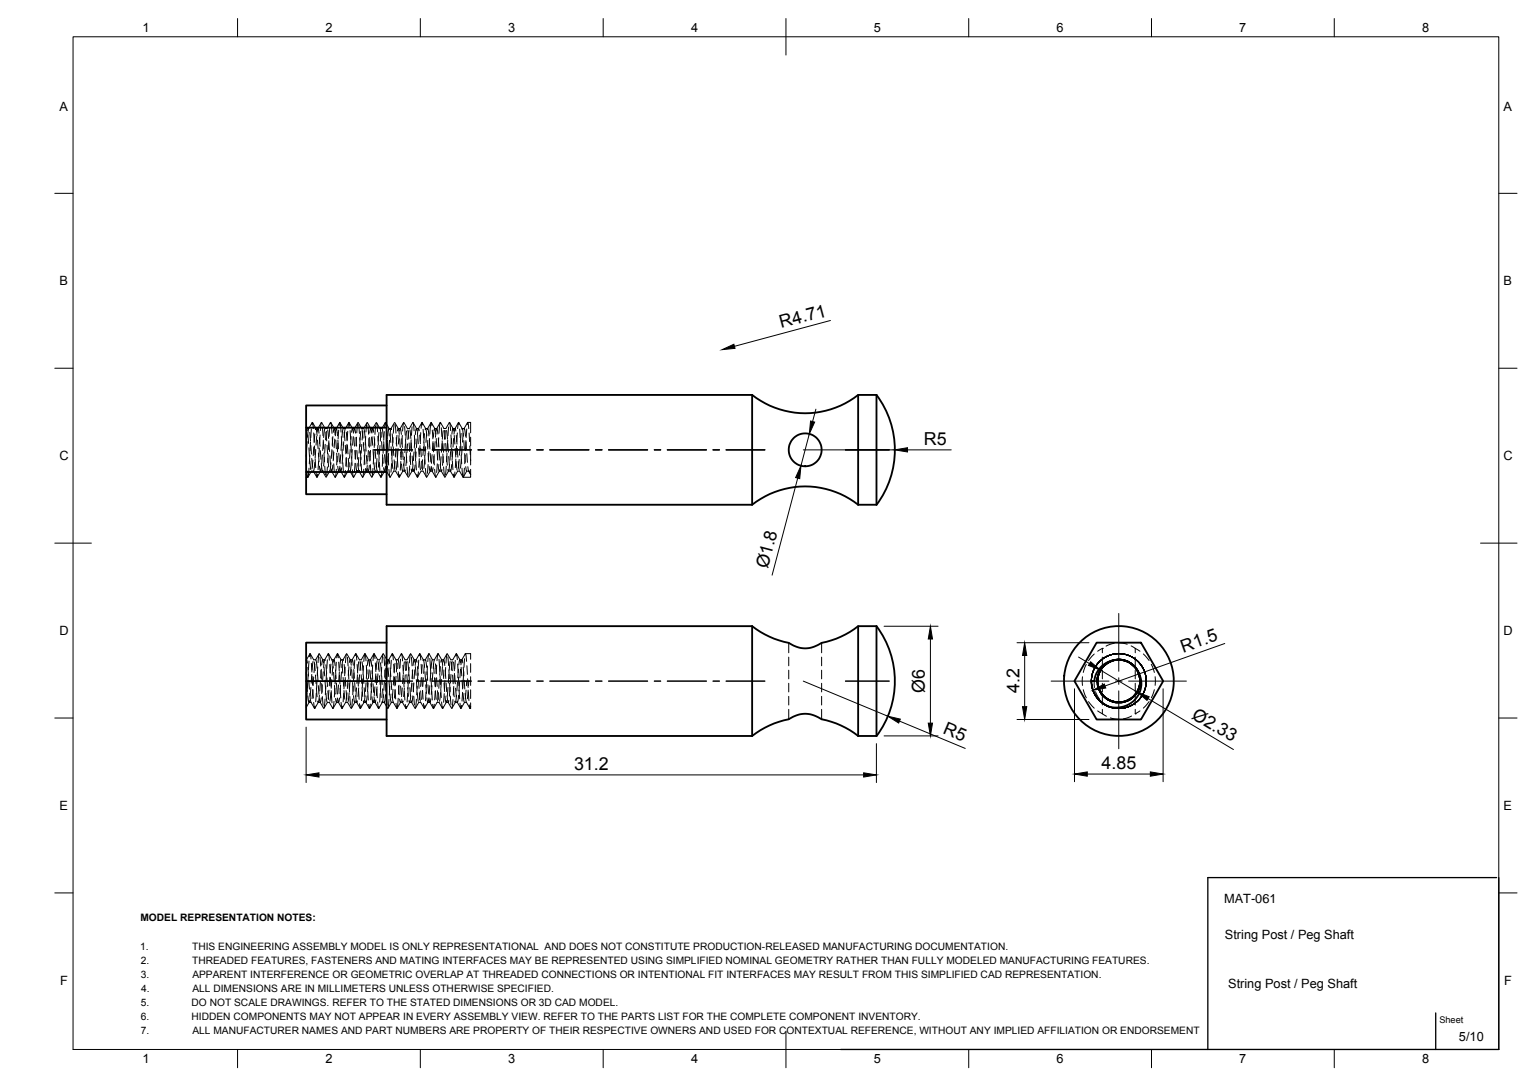
ISO-10303-21;
HEADER;
/* Generated by software containing ST-Developer
 * from STEP Tools, Inc. (www.steptools.com) 
 */

FILE_DESCRIPTION(
/* description */ ('', 'CAx-IF Rec.Pracs.---Representation and Presentation of Product Manufa
cturing Information (PMI)---4.0---2014-10-13'),
/* implementation_level */ '2;1');

FILE_NAME(
/* name */ 'String Post _ Peg Shaft.step',
/* time_stamp */ '2026-10-28T14:45:12+01:00',
/* author */ (''),
/* organization */ (''),
/* preprocessor_version */ 'ST-DEVELOPER v20.2',
/* originating_system */ 'Autodesk Translation Framework v15.17.0.0',
/* authorisation */ '');

FILE_SCHEMA (('AP242_MANAGED_MODEL_BASED_3D_ENGINEERING_MIM_LF { 1 0 10303 442 2 1 4 }'));
ENDSEC;

DATA;
#10=MECHANICAL_DESIGN_GEOMETRIC_PRESENTATION_REPRESENTATION('',(#260),#52164);
#207=TOROIDAL_SURFACE('',#9675,6.705,4.705);
#234=SHAPE_REPRESENTATION_RELATIONSHIP('SRR','None',#52213,#247);
#247=ADVANCED_BREP_SHAPE_REPRESENTATION('',(#273),#52153);
#260=STYLED_ITEM('',(#52318),#273);
#273=MANIFOLD_SOLID_BREP('Body1',#9120);
#285=SPHERICAL_SURFACE('',#9677,5.);
#293=FACE_BOUND('',#1236,.T.);
#294=FACE_BOUND('',#1240,.T.);
#295=FACE_BOUND('',#1241,.T.);
#296=FACE_BOUND('',#1251,.T.);
#343=B_SPLINE_SURFACE_WITH_KNOTS('',3,3,((#20414,#20415,#20416,#20417,#20418,
#20419,#20420,#20421,#20422,#20423,#20424,#20425,#20426,#20427,#20428,#20429,
#20430,#20431,#20432,#20433,#20434,#20435,#20436,#20437,#20438,#20439,#20440,
#20441,#20442,#20443,#20444,#20445,#20446,#20447,#20448),(#20449,#20450,
#20451,#20452,#20453,#20454,#20455,#20456,#20457,#20458,#20459,#20460,#20461,
#20462,#20463,#20464,#20465,#20466,#20467,#20468,#20469,#20470,#20471,#20472,
#20473,#20474,#20475,#20476,#20477,#20478,#20479,#20480,#20481,#20482,#20483),
(#20484,#20485,#20486,#20487,#20488,#20489,#20490,#20491,#20492,#20493,
#20494,#20495,#20496,#20497,#20498,#20499,#20500,#20501,#20502,#20503,#20504,
#20505,#20506,#20507,#20508,#20509,#20510,#20511,#20512,#20513,#20514,#20515,
#20516,#20517,#20518),(#20519,#20520,#20521,#20522,#20523,#20524,#20525,
#20526,#20527,#20528,#20529,#20530,#20531,#20532,#20533,#20534,#20535,#20536,
#20537,#20538,#20539,#20540,#20541,#20542,#20543,#20544,#20545,#20546,#20547,
#20548,#20549,#20550,#20551,#20552,#20553)),.UNSPECIFIED.,.F.,.F.,.F.,(4,
4),(4,1,1,1,1,1,1,1,1,1,1,1,1,1,1,1,1,1,1,1,1,1,1,1,1,1,1,1,1,1,1,1,4),
(-0.1053316651847,1.105331665185),(-0.01760502747868,0.01100314217417,0.03961131182703,
0.06821948147988,0.09682765113273,0.1254358207856,0.1540439904384,0.1826521600913,
0.2112603297441,0.239868499397,0.2684766690498,0.2970848387027,0.3256930083555,
0.3543011780084,0.3829093476613,0.4115175173141,0.440125686967,0.4687338566198,
0.4973420262727,0.5259501959255,0.5545583655784,0.5831665352312,0.6117747048841,
0.6403828745369,0.6689910441898,0.6975992138426,0.7262073834955,0.7548155531483,
0.7834237228012,0.812031892454,0.8406400621069,0.8692482317597,0.8978564014126),
 .UNSPECIFIED.);
#344=B_SPLINE_SURFACE_WITH_KNOTS('',3,3,((#20875,#20876,#20877,#20878,#20879,
#20880,#20881,#20882,#20883,#20884,#20885,#20886,#20887,#20888,#20889,#20890,
#20891,#20892,#20893,#20894,#20895,#20896,#20897,#20898,#20899,#20900,#20901,
#20902,#20903,#20904,#20905,#20906,#20907,#20908,#20909),(#20910,#20911,
#20912,#20913,#20914,#20915,#20916,#20917,#20918,#20919,#20920,#20921,#20922,
#20923,#20924,#20925,#20926,#20927,#20928,#20929,#20930,#20931,#20932,#20933,
#20934,#20935,#20936,#20937,#20938,#20939,#20940,#20941,#20942,#20943,#20944),
(#20945,#20946,#20947,#20948,#20949,#20950,#20951,#20952,#20953,#20954,
#20955,#20956,#20957,#20958,#20959,#20960,#20961,#20962,#20963,#20964,#20965,
#20966,#20967,#20968,#20969,#20970,#20971,#20972,#20973,#20974,#20975,#20976,
#20977,#20978,#20979),(#20980,#20981,#20982,#20983,#20984,#20985,#20986,
#20987,#20988,#20989,#20990,#20991,#20992,#20993,#20994,#20995,#20996,#20997,
#20998,#20999,#21000,#21001,#21002,#21003,#21004,#21005,#21006,#21007,#21008,
#21009,#21010,#21011,#21012,#21013,#21014)),.UNSPECIFIED.,.F.,.F.,.F.,(4,
4),(4,1,1,1,1,1,1,1,1,1,1,1,1,1,1,1,1,1,1,1,1,1,1,1,1,1,1,1,1,1,1,1,4),
(-0.1053316651848,1.105331665185),(-0.02,0.0125,0.045,0.0775,0.11,0.1425,
0.175,0.2075,0.24,0.2725,0.305,0.3375,0.37,0.4025,0.435,0.4675,0.5,0.5325,
0.565,0.5975,0.63,0.6625,0.695,0.7275,0.76,0.7925,0.825,0.8575,0.89,0.9225,
0.955,0.9875,1.02),.UNSPECIFIED.);
#345=B_SPLINE_SURFACE_WITH_KNOTS('',3,3,((#21330,#21331,#21332,#21333,#21334,
#21335,#21336,#21337,#21338,#21339,#21340,#21341,#21342,#21343,#21344,#21345,
#21346,#21347,#21348,#21349,#21350,#21351,#21352,#21353,#21354,#21355,#21356,
#21357,#21358,#21359,#21360,#21361,#21362,#21363,#21364),(#21365,#21366,
#21367,#21368,#21369,#21370,#21371,#21372,#21373,#21374,#21375,#21376,#21377,
#21378,#21379,#21380,#21381,#21382,#21383,#21384,#21385,#21386,#21387,#21388,
#21389,#21390,#21391,#21392,#21393,#21394,#21395,#21396,#21397,#21398,#21399),
(#21400,#21401,#21402,#21403,#21404,#21405,#21406,#21407,#21408,#21409,
#21410,#21411,#21412,#21413,#21414,#21415,#21416,#21417,#21418,#21419,#21420,
#21421,#21422,#21423,#21424,#21425,#21426,#21427,#21428,#21429,#21430,#21431,
#21432,#21433,#21434),(#21435,#21436,#21437,#21438,#21439,#21440,#21441,
#21442,#21443,#21444,#21445,#21446,#21447,#21448,#21449,#21450,#21451,#21452,
#21453,#21454,#21455,#21456,#21457,#21458,#21459,#21460,#21461,#21462,#21463,
#21464,#21465,#21466,#21467,#21468,#21469)),.UNSPECIFIED.,.F.,.F.,.F.,(4,
4),(4,1,1,1,1,1,1,1,1,1,1,1,1,1,1,1,1,1,1,1,1,1,1,1,1,1,1,1,1,1,1,1,4),
(-0.3507678241798,1.35076782418),(-0.01888802807688,0.01180501754805,0.04249806317297,
0.0731911087979,0.1038841544228,0.1345772000478,0.1652702456727,0.1959632912976,
0.2266563369225,0.2573493825475,0.2880424281724,0.3187354737973,0.3494285194222,
0.3801215650472,0.4108146106721,0.441507656297,0.4722007019219,0.5028937475469,
0.5335867931718,0.5642798387967,0.5949728844216,0.6256659300466,0.6563589756715,
0.6870520212964,0.7177450669213,0.7484381125463,0.7791311581712,0.8098242037961,
0.840517249421,0.871210295046,0.9019033406709,0.9325963862958,0.9632894319207),
 .UNSPECIFIED.);
#346=B_SPLINE_SURFACE_WITH_KNOTS('',3,3,((#21471,#21472,#21473,#21474,#21475,
#21476,#21477,#21478,#21479,#21480,#21481,#21482,#21483,#21484,#21485,#21486,
#21487,#21488,#21489,#21490,#21491,#21492,#21493,#21494,#21495,#21496,#21497,
#21498,#21499,#21500,#21501,#21502,#21503,#21504,#21505),(#21506,#21507,
#21508,#21509,#21510,#21511,#21512,#21513,#21514,#21515,#21516,#21517,#21518,
#21519,#21520,#21521,#21522,#21523,#21524,#21525,#21526,#21527,#21528,#21529,
#21530,#21531,#21532,#21533,#21534,#21535,#21536,#21537,#21538,#21539,#21540),
(#21541,#21542,#21543,#21544,#21545,#21546,#21547,#21548,#21549,#21550,
#21551,#21552,#21553,#21554,#21555,#21556,#21557,#21558,#21559,#21560,#21561,
#21562,#21563,#21564,#21565,#21566,#21567,#21568,#21569,#21570,#21571,#21572,
#21573,#21574,#21575),(#21576,#21577,#21578,#21579,#21580,#21581,#21582,
#21583,#21584,#21585,#21586,#21587,#21588,#21589,#21590,#21591,#21592,#21593,
#21594,#21595,#21596,#21597,#21598,#21599,#21600,#21601,#21602,#21603,#21604,
#21605,#21606,#21607,#21608,#21609,#21610)),.UNSPECIFIED.,.F.,.F.,.F.,(4,
4),(4,1,1,1,1,1,1,1,1,1,1,1,1,1,1,1,1,1,1,1,1,1,1,1,1,1,1,1,1,1,1,1,4),
(-0.3507678241798,1.35076782418),(-0.02,0.0125,0.045,0.0775,0.11,0.1425,
0.175,0.2075,0.24,0.2725,0.305,0.3375,0.37,0.4025,0.435,0.4675,0.5,0.5325,
0.565,0.5975,0.63,0.6625,0.695,0.7275,0.76,0.7925,0.825,0.8575,0.89,0.9225,
0.955,0.9875,1.02),.UNSPECIFIED.);
#347=B_SPLINE_SURFACE_WITH_KNOTS('',3,3,((#21858,#21859,#21860,#21861,#21862,
#21863,#21864,#21865,#21866,#21867,#21868,#21869,#21870,#21871,#21872,#21873,
#21874,#21875,#21876,#21877,#21878,#21879,#21880,#21881,#21882,#21883,#21884,
#21885,#21886,#21887,#21888,#21889,#21890,#21891,#21892),(#21893,#21894,
#21895,#21896,#21897,#21898,#21899,#21900,#21901,#21902,#21903,#21904,#21905,
#21906,#21907,#21908,#21909,#21910,#21911,#21912,#21913,#21914,#21915,#21916,
#21917,#21918,#21919,#21920,#21921,#21922,#21923,#21924,#21925,#21926,#21927),
(#21928,#21929,#21930,#21931,#21932,#21933,#21934,#21935,#21936,#21937,
#21938,#21939,#21940,#21941,#21942,#21943,#21944,#21945,#21946,#21947,#21948,
#21949,#21950,#21951,#21952,#21953,#21954,#21955,#21956,#21957,#21958,#21959,
#21960,#21961,#21962),(#21963,#21964,#21965,#21966,#21967,#21968,#21969,
#21970,#21971,#21972,#21973,#21974,#21975,#21976,#21977,#21978,#21979,#21980,
#21981,#21982,#21983,#21984,#21985,#21986,#21987,#21988,#21989,#21990,#21991,
#21992,#21993,#21994,#21995,#21996,#21997)),.UNSPECIFIED.,.F.,.F.,.F.,(4,
4),(4,1,1,1,1,1,1,1,1,1,1,1,1,1,1,1,1,1,1,1,1,1,1,1,1,1,1,1,1,1,1,1,4),
(-0.3507678241798,1.35076782418),(-0.02,0.0125,0.045,0.0775,0.11,0.1425,
0.175,0.2075,0.24,0.2725,0.305,0.3375,0.37,0.4025,0.435,0.4675,0.5,0.5325,
0.565,0.5975,0.63,0.6625,0.695,0.7275,0.76,0.7925,0.825,0.8575,0.89,0.9225,
0.955,0.9875,1.02),.UNSPECIFIED.);
#348=B_SPLINE_SURFACE_WITH_KNOTS('',3,3,((#22245,#22246,#22247,#22248,#22249,
#22250,#22251,#22252,#22253,#22254,#22255,#22256,#22257,#22258,#22259,#22260,
#22261,#22262,#22263,#22264,#22265,#22266,#22267,#22268,#22269,#22270,#22271,
#22272,#22273,#22274,#22275,#22276,#22277,#22278,#22279),(#22280,#22281,
#22282,#22283,#22284,#22285,#22286,#22287,#22288,#22289,#22290,#22291,#22292,
#22293,#22294,#22295,#22296,#22297,#22298,#22299,#22300,#22301,#22302,#22303,
#22304,#22305,#22306,#22307,#22308,#22309,#22310,#22311,#22312,#22313,#22314),
(#22315,#22316,#22317,#22318,#22319,#22320,#22321,#22322,#22323,#22324,
#22325,#22326,#22327,#22328,#22329,#22330,#22331,#22332,#22333,#22334,#22335,
#22336,#22337,#22338,#22339,#22340,#22341,#22342,#22343,#22344,#22345,#22346,
#22347,#22348,#22349),(#22350,#22351,#22352,#22353,#22354,#22355,#22356,
#22357,#22358,#22359,#22360,#22361,#22362,#22363,#22364,#22365,#22366,#22367,
#22368,#22369,#22370,#22371,#22372,#22373,#22374,#22375,#22376,#22377,#22378,
#22379,#22380,#22381,#22382,#22383,#22384)),.UNSPECIFIED.,.F.,.F.,.F.,(4,
4),(4,1,1,1,1,1,1,1,1,1,1,1,1,1,1,1,1,1,1,1,1,1,1,1,1,1,1,1,1,1,1,1,4),
(-0.3507678241798,1.35076782418),(-0.02,0.0125,0.045,0.0775,0.11,0.1425,
0.175,0.2075,0.24,0.2725,0.305,0.3375,0.37,0.4025,0.435,0.4675,0.5,0.5325,
0.565,0.5975,0.63,0.6625,0.695,0.7275,0.76,0.7925,0.825,0.8575,0.89,0.9225,
0.955,0.9875,1.02),.UNSPECIFIED.);
#349=B_SPLINE_SURFACE_WITH_KNOTS('',3,3,((#22632,#22633,#22634,#22635,#22636,
#22637,#22638,#22639,#22640,#22641,#22642,#22643,#22644,#22645,#22646,#22647,
#22648,#22649,#22650,#22651,#22652,#22653,#22654,#22655,#22656,#22657,#22658,
#22659,#22660,#22661,#22662,#22663,#22664,#22665,#22666),(#22667,#22668,
#22669,#22670,#22671,#22672,#22673,#22674,#22675,#22676,#22677,#22678,#22679,
#22680,#22681,#22682,#22683,#22684,#22685,#22686,#22687,#22688,#22689,#22690,
#22691,#22692,#22693,#22694,#22695,#22696,#22697,#22698,#22699,#22700,#22701),
(#22702,#22703,#22704,#22705,#22706,#22707,#22708,#22709,#22710,#22711,
#22712,#22713,#22714,#22715,#22716,#22717,#22718,#22719,#22720,#22721,#22722,
#22723,#22724,#22725,#22726,#22727,#22728,#22729,#22730,#22731,#22732,#22733,
#22734,#22735,#22736),(#22737,#22738,#22739,#22740,#22741,#22742,#22743,
#22744,#22745,#22746,#22747,#22748,#22749,#22750,#22751,#22752,#22753,#22754,
#22755,#22756,#22757,#22758,#22759,#22760,#22761,#22762,#22763,#22764,#22765,
#22766,#22767,#22768,#22769,#22770,#22771)),.UNSPECIFIED.,.F.,.F.,.F.,(4,
4),(4,1,1,1,1,1,1,1,1,1,1,1,1,1,1,1,1,1,1,1,1,1,1,1,1,1,1,1,1,1,1,1,4),
(-0.3507678241798,1.35076782418),(-0.02,0.0125,0.045,0.0775,0.11,0.1425,
0.175,0.2075,0.24,0.2725,0.305,0.3375,0.37,0.4025,0.435,0.4675,0.5,0.5325,
0.565,0.5975,0.63,0.6625,0.695,0.7275,0.76,0.7925,0.825,0.8575,0.89,0.9225,
0.955,0.9875,1.02),.UNSPECIFIED.);
#350=B_SPLINE_SURFACE_WITH_KNOTS('',3,3,((#23060,#23061,#23062,#23063,#23064,
#23065,#23066,#23067,#23068,#23069,#23070,#23071,#23072,#23073,#23074,#23075,
#23076,#23077,#23078,#23079,#23080,#23081,#23082,#23083,#23084,#23085,#23086,
#23087,#23088,#23089,#23090,#23091,#23092,#23093,#23094),(#23095,#23096,
#23097,#23098,#23099,#23100,#23101,#23102,#23103,#23104,#23105,#23106,#23107,
#23108,#23109,#23110,#23111,#23112,#23113,#23114,#23115,#23116,#23117,#23118,
#23119,#23120,#23121,#23122,#23123,#23124,#23125,#23126,#23127,#23128,#23129),
(#23130,#23131,#23132,#23133,#23134,#23135,#23136,#23137,#23138,#23139,
#23140,#23141,#23142,#23143,#23144,#23145,#23146,#23147,#23148,#23149,#23150,
#23151,#23152,#23153,#23154,#23155,#23156,#23157,#23158,#23159,#23160,#23161,
#23162,#23163,#23164),(#23165,#23166,#23167,#23168,#23169,#23170,#23171,
#23172,#23173,#23174,#23175,#23176,#23177,#23178,#23179,#23180,#23181,#23182,
#23183,#23184,#23185,#23186,#23187,#23188,#23189,#23190,#23191,#23192,#23193,
#23194,#23195,#23196,#23197,#23198,#23199)),.UNSPECIFIED.,.F.,.F.,.F.,(4,
4),(4,1,1,1,1,1,1,1,1,1,1,1,1,1,1,1,1,1,1,1,1,1,1,1,1,1,1,1,1,1,1,1,4),
(-0.1053316651848,1.105331665185),(-0.02,0.0125,0.045,0.0775,0.11,0.1425,
0.175,0.2075,0.24,0.2725,0.305,0.3375,0.37,0.4025,0.435,0.4675,0.5,0.5325,
0.565,0.5975,0.63,0.6625,0.695,0.7275,0.76,0.7925,0.825,0.8575,0.89,0.9225,
0.955,0.9875,1.02),.UNSPECIFIED.);
#351=B_SPLINE_SURFACE_WITH_KNOTS('',3,3,((#23447,#23448,#23449,#23450,#23451,
#23452,#23453,#23454,#23455,#23456,#23457,#23458,#23459,#23460,#23461,#23462,
#23463,#23464,#23465,#23466,#23467,#23468,#23469,#23470,#23471,#23472,#23473,
#23474,#23475,#23476,#23477,#23478,#23479,#23480,#23481),(#23482,#23483,
#23484,#23485,#23486,#23487,#23488,#23489,#23490,#23491,#23492,#23493,#23494,
#23495,#23496,#23497,#23498,#23499,#23500,#23501,#23502,#23503,#23504,#23505,
#23506,#23507,#23508,#23509,#23510,#23511,#23512,#23513,#23514,#23515,#23516),
(#23517,#23518,#23519,#23520,#23521,#23522,#23523,#23524,#23525,#23526,
#23527,#23528,#23529,#23530,#23531,#23532,#23533,#23534,#23535,#23536,#23537,
#23538,#23539,#23540,#23541,#23542,#23543,#23544,#23545,#23546,#23547,#23548,
#23549,#23550,#23551),(#23552,#23553,#23554,#23555,#23556,#23557,#23558,
#23559,#23560,#23561,#23562,#23563,#23564,#23565,#23566,#23567,#23568,#23569,
#23570,#23571,#23572,#23573,#23574,#23575,#23576,#23577,#23578,#23579,#23580,
#23581,#23582,#23583,#23584,#23585,#23586)),.UNSPECIFIED.,.F.,.F.,.F.,(4,
4),(4,1,1,1,1,1,1,1,1,1,1,1,1,1,1,1,1,1,1,1,1,1,1,1,1,1,1,1,1,1,1,1,4),
(-0.1053316651847,1.105331665185),(-0.02,0.0125,0.045,0.0775,0.11,0.1425,
0.175,0.2075,0.24,0.2725,0.305,0.3375,0.37,0.4025,0.435,0.4675,0.5,0.5325,
0.565,0.5975,0.63,0.6625,0.695,0.7275,0.76,0.7925,0.825,0.8575,0.89,0.9225,
0.955,0.9875,1.02),.UNSPECIFIED.);
#352=B_SPLINE_SURFACE_WITH_KNOTS('',3,3,((#23641,#23642,#23643,#23644,#23645,
#23646,#23647,#23648,#23649,#23650,#23651,#23652,#23653,#23654,#23655,#23656,
#23657,#23658,#23659,#23660,#23661,#23662,#23663,#23664,#23665,#23666,#23667,
#23668,#23669,#23670,#23671,#23672,#23673,#23674,#23675),(#23676,#23677,
#23678,#23679,#23680,#23681,#23682,#23683,#23684,#23685,#23686,#23687,#23688,
#23689,#23690,#23691,#23692,#23693,#23694,#23695,#23696,#23697,#23698,#23699,
#23700,#23701,#23702,#23703,#23704,#23705,#23706,#23707,#23708,#23709,#23710),
(#23711,#23712,#23713,#23714,#23715,#23716,#23717,#23718,#23719,#23720,
#23721,#23722,#23723,#23724,#23725,#23726,#23727,#23728,#23729,#23730,#23731,
#23732,#23733,#23734,#23735,#23736,#23737,#23738,#23739,#23740,#23741,#23742,
#23743,#23744,#23745),(#23746,#23747,#23748,#23749,#23750,#23751,#23752,
#23753,#23754,#23755,#23756,#23757,#23758,#23759,#23760,#23761,#23762,#23763,
#23764,#23765,#23766,#23767,#23768,#23769,#23770,#23771,#23772,#23773,#23774,
#23775,#23776,#23777,#23778,#23779,#23780)),.UNSPECIFIED.,.F.,.F.,.F.,(4,
4),(4,1,1,1,1,1,1,1,1,1,1,1,1,1,1,1,1,1,1,1,1,1,1,1,1,1,1,1,1,1,1,1,4),
(-0.1053316651847,1.105331665185),(-0.02,0.0125,0.045,0.0775,0.11,0.1425,
0.175,0.2075,0.24,0.2725,0.305,0.3375,0.37,0.4025,0.435,0.4675,0.5,0.5325,
0.565,0.5975,0.63,0.6625,0.695,0.7275,0.76,0.7925,0.825,0.8575,0.89,0.9225,
0.955,0.9875,1.02),.UNSPECIFIED.);
#353=B_SPLINE_SURFACE_WITH_KNOTS('',3,3,((#24018,#24019,#24020,#24021,#24022,
#24023,#24024,#24025,#24026,#24027,#24028,#24029,#24030,#24031,#24032,#24033,
#24034,#24035,#24036,#24037,#24038,#24039,#24040,#24041,#24042,#24043,#24044,
#24045,#24046,#24047,#24048,#24049,#24050,#24051,#24052),(#24053,#24054,
#24055,#24056,#24057,#24058,#24059,#24060,#24061,#24062,#24063,#24064,#24065,
#24066,#24067,#24068,#24069,#24070,#24071,#24072,#24073,#24074,#24075,#24076,
#24077,#24078,#24079,#24080,#24081,#24082,#24083,#24084,#24085,#24086,#24087),
(#24088,#24089,#24090,#24091,#24092,#24093,#24094,#24095,#24096,#24097,
#24098,#24099,#24100,#24101,#24102,#24103,#24104,#24105,#24106,#24107,#24108,
#24109,#24110,#24111,#24112,#24113,#24114,#24115,#24116,#24117,#24118,#24119,
#24120,#24121,#24122),(#24123,#24124,#24125,#24126,#24127,#24128,#24129,
#24130,#24131,#24132,#24133,#24134,#24135,#24136,#24137,#24138,#24139,#24140,
#24141,#24142,#24143,#24144,#24145,#24146,#24147,#24148,#24149,#24150,#24151,
#24152,#24153,#24154,#24155,#24156,#24157)),.UNSPECIFIED.,.F.,.F.,.F.,(4,
4),(4,1,1,1,1,1,1,1,1,1,1,1,1,1,1,1,1,1,1,1,1,1,1,1,1,1,1,1,1,1,1,1,4),
(-0.1053316651848,1.105331665185),(-0.02,0.0125,0.045,0.0775,0.11,0.1425,
0.175,0.2075,0.24,0.2725,0.305,0.3375,0.37,0.4025,0.435,0.4675,0.5,0.5325,
0.565,0.5975,0.63,0.6625,0.695,0.7275,0.76,0.7925,0.825,0.8575,0.89,0.9225,
0.955,0.9875,1.02),.UNSPECIFIED.);
#354=B_SPLINE_SURFACE_WITH_KNOTS('',3,3,((#24159,#24160,#24161,#24162,#24163,
#24164,#24165,#24166,#24167,#24168,#24169,#24170,#24171,#24172,#24173,#24174,
#24175,#24176,#24177,#24178,#24179,#24180,#24181,#24182,#24183,#24184,#24185,
#24186,#24187,#24188,#24189,#24190,#24191,#24192,#24193),(#24194,#24195,
#24196,#24197,#24198,#24199,#24200,#24201,#24202,#24203,#24204,#24205,#24206,
#24207,#24208,#24209,#24210,#24211,#24212,#24213,#24214,#24215,#24216,#24217,
#24218,#24219,#24220,#24221,#24222,#24223,#24224,#24225,#24226,#24227,#24228),
(#24229,#24230,#24231,#24232,#24233,#24234,#24235,#24236,#24237,#24238,
#24239,#24240,#24241,#24242,#24243,#24244,#24245,#24246,#24247,#24248,#24249,
#24250,#24251,#24252,#24253,#24254,#24255,#24256,#24257,#24258,#24259,#24260,
#24261,#24262,#24263),(#24264,#24265,#24266,#24267,#24268,#24269,#24270,
#24271,#24272,#24273,#24274,#24275,#24276,#24277,#24278,#24279,#24280,#24281,
#24282,#24283,#24284,#24285,#24286,#24287,#24288,#24289,#24290,#24291,#24292,
#24293,#24294,#24295,#24296,#24297,#24298)),.UNSPECIFIED.,.F.,.F.,.F.,(4,
4),(4,1,1,1,1,1,1,1,1,1,1,1,1,1,1,1,1,1,1,1,1,1,1,1,1,1,1,1,1,1,1,1,4),
(-0.1053316651848,1.105331665185),(-0.02,0.0125,0.045,0.0775,0.11,0.1425,
0.175,0.2075,0.24,0.2725,0.305,0.3375,0.37,0.4025,0.435,0.4675,0.5,0.5325,
0.565,0.5975,0.63,0.6625,0.695,0.7275,0.76,0.7925,0.825,0.8575,0.89,0.9225,
0.955,0.9875,1.02),.UNSPECIFIED.);
#355=B_SPLINE_SURFACE_WITH_KNOTS('',3,3,((#24485,#24486,#24487,#24488,#24489,
#24490,#24491,#24492,#24493,#24494,#24495,#24496,#24497,#24498,#24499,#24500,
#24501,#24502,#24503,#24504,#24505,#24506,#24507,#24508,#24509,#24510,#24511,
#24512,#24513,#24514,#24515,#24516,#24517,#24518,#24519),(#24520,#24521,
#24522,#24523,#24524,#24525,#24526,#24527,#24528,#24529,#24530,#24531,#24532,
#24533,#24534,#24535,#24536,#24537,#24538,#24539,#24540,#24541,#24542,#24543,
#24544,#24545,#24546,#24547,#24548,#24549,#24550,#24551,#24552,#24553,#24554),
(#24555,#24556,#24557,#24558,#24559,#24560,#24561,#24562,#24563,#24564,
#24565,#24566,#24567,#24568,#24569,#24570,#24571,#24572,#24573,#24574,#24575,
#24576,#24577,#24578,#24579,#24580,#24581,#24582,#24583,#24584,#24585,#24586,
#24587,#24588,#24589),(#24590,#24591,#24592,#24593,#24594,#24595,#24596,
#24597,#24598,#24599,#24600,#24601,#24602,#24603,#24604,#24605,#24606,#24607,
#24608,#24609,#24610,#24611,#24612,#24613,#24614,#24615,#24616,#24617,#24618,
#24619,#24620,#24621,#24622,#24623,#24624)),.UNSPECIFIED.,.F.,.F.,.F.,(4,
4),(4,1,1,1,1,1,1,1,1,1,1,1,1,1,1,1,1,1,1,1,1,1,1,1,1,1,1,1,1,1,1,1,4),
(-0.1053316651847,1.105331665185),(-0.02,0.0125,0.045,0.0775,0.11,0.1425,
0.175,0.2075,0.24,0.2725,0.305,0.3375,0.37,0.4025,0.435,0.4675,0.5,0.5325,
0.565,0.5975,0.63,0.6625,0.695,0.7275,0.76,0.7925,0.825,0.8575,0.89,0.9225,
0.955,0.9875,1.02),.UNSPECIFIED.);
#356=B_SPLINE_SURFACE_WITH_KNOTS('',3,3,((#24675,#24676,#24677,#24678,#24679,
#24680,#24681,#24682,#24683,#24684,#24685,#24686,#24687,#24688,#24689,#24690,
#24691,#24692,#24693,#24694,#24695,#24696,#24697,#24698,#24699,#24700,#24701,
#24702,#24703,#24704,#24705,#24706,#24707,#24708,#24709),(#24710,#24711,
#24712,#24713,#24714,#24715,#24716,#24717,#24718,#24719,#24720,#24721,#24722,
#24723,#24724,#24725,#24726,#24727,#24728,#24729,#24730,#24731,#24732,#24733,
#24734,#24735,#24736,#24737,#24738,#24739,#24740,#24741,#24742,#24743,#24744),
(#24745,#24746,#24747,#24748,#24749,#24750,#24751,#24752,#24753,#24754,
#24755,#24756,#24757,#24758,#24759,#24760,#24761,#24762,#24763,#24764,#24765,
#24766,#24767,#24768,#24769,#24770,#24771,#24772,#24773,#24774,#24775,#24776,
#24777,#24778,#24779),(#24780,#24781,#24782,#24783,#24784,#24785,#24786,
#24787,#24788,#24789,#24790,#24791,#24792,#24793,#24794,#24795,#24796,#24797,
#24798,#24799,#24800,#24801,#24802,#24803,#24804,#24805,#24806,#24807,#24808,
#24809,#24810,#24811,#24812,#24813,#24814)),.UNSPECIFIED.,.F.,.F.,.F.,(4,
4),(4,1,1,1,1,1,1,1,1,1,1,1,1,1,1,1,1,1,1,1,1,1,1,1,1,1,1,1,1,1,1,1,4),
(-0.1053316651847,1.105331665185),(-0.02,0.0125,0.045,0.0775,0.11,0.1425,
0.175,0.2075,0.24,0.2725,0.305,0.3375,0.37,0.4025,0.435,0.4675,0.5,0.5325,
0.565,0.5975,0.63,0.6625,0.695,0.7275,0.76,0.7925,0.825,0.8575,0.89,0.9225,
0.955,0.9875,1.02),.UNSPECIFIED.);
#357=B_SPLINE_SURFACE_WITH_KNOTS('',3,3,((#24997,#24998,#24999,#25000,#25001,
#25002,#25003,#25004,#25005,#25006,#25007,#25008,#25009,#25010,#25011,#25012,
#25013,#25014,#25015,#25016,#25017,#25018,#25019,#25020,#25021,#25022,#25023,
#25024,#25025,#25026,#25027,#25028,#25029,#25030,#25031),(#25032,#25033,
#25034,#25035,#25036,#25037,#25038,#25039,#25040,#25041,#25042,#25043,#25044,
#25045,#25046,#25047,#25048,#25049,#25050,#25051,#25052,#25053,#25054,#25055,
#25056,#25057,#25058,#25059,#25060,#25061,#25062,#25063,#25064,#25065,#25066),
(#25067,#25068,#25069,#25070,#25071,#25072,#25073,#25074,#25075,#25076,
#25077,#25078,#25079,#25080,#25081,#25082,#25083,#25084,#25085,#25086,#25087,
#25088,#25089,#25090,#25091,#25092,#25093,#25094,#25095,#25096,#25097,#25098,
#25099,#25100,#25101),(#25102,#25103,#25104,#25105,#25106,#25107,#25108,
#25109,#25110,#25111,#25112,#25113,#25114,#25115,#25116,#25117,#25118,#25119,
#25120,#25121,#25122,#25123,#25124,#25125,#25126,#25127,#25128,#25129,#25130,
#25131,#25132,#25133,#25134,#25135,#25136)),.UNSPECIFIED.,.F.,.F.,.F.,(4,
4),(4,1,1,1,1,1,1,1,1,1,1,1,1,1,1,1,1,1,1,1,1,1,1,1,1,1,1,1,1,1,1,1,4),
(-0.1053316651848,1.105331665185),(-0.02,0.0125,0.045,0.0775,0.11,0.1425,
0.175,0.2075,0.24,0.2725,0.305,0.3375,0.37,0.4025,0.435,0.4675,0.5,0.5325,
0.565,0.5975,0.63,0.6625,0.695,0.7275,0.76,0.7925,0.825,0.8575,0.89,0.9225,
0.955,0.9875,1.02),.UNSPECIFIED.);
#425=PLANE('',#9668);
#426=PLANE('',#9680);
#427=PLANE('',#9681);
#428=PLANE('',#9682);
#429=PLANE('',#9683);
#430=PLANE('',#9684);
#431=PLANE('',#9685);
#432=PLANE('',#9686);
#433=PLANE('',#9689);
#434=PLANE('',#9690);
#435=PLANE('',#9693);
#693=FACE_OUTER_BOUND('',#1235,.T.);
#694=FACE_OUTER_BOUND('',#1237,.T.);
#695=FACE_OUTER_BOUND('',#1238,.T.);
#696=FACE_OUTER_BOUND('',#1239,.T.);
#697=FACE_OUTER_BOUND('',#1242,.T.);
#698=FACE_OUTER_BOUND('',#1243,.T.);
#699=FACE_OUTER_BOUND('',#1244,.T.);
#700=FACE_OUTER_BOUND('',#1245,.T.);
#701=FACE_OUTER_BOUND('',#1246,.T.);
#702=FACE_OUTER_BOUND('',#1247,.T.);
#703=FACE_OUTER_BOUND('',#1248,.T.);
#704=FACE_OUTER_BOUND('',#1249,.T.);
#705=FACE_OUTER_BOUND('',#1250,.T.);
#706=FACE_OUTER_BOUND('',#1252,.T.);
#707=FACE_OUTER_BOUND('',#1253,.T.);
#708=FACE_OUTER_BOUND('',#1254,.T.);
#709=FACE_OUTER_BOUND('',#1255,.T.);
#710=FACE_OUTER_BOUND('',#1256,.T.);
#711=FACE_OUTER_BOUND('',#1257,.T.);
#712=FACE_OUTER_BOUND('',#1258,.T.);
#713=FACE_OUTER_BOUND('',#1259,.T.);
#714=FACE_OUTER_BOUND('',#1260,.T.);
#715=FACE_OUTER_BOUND('',#1261,.T.);
#716=FACE_OUTER_BOUND('',#1262,.T.);
#717=FACE_OUTER_BOUND('',#1263,.T.);
#718=FACE_OUTER_BOUND('',#1264,.T.);
#719=FACE_OUTER_BOUND('',#1265,.T.);
#720=FACE_OUTER_BOUND('',#1266,.T.);
#721=FACE_OUTER_BOUND('',#1267,.T.);
#722=FACE_OUTER_BOUND('',#1268,.T.);
#723=FACE_OUTER_BOUND('',#1269,.T.);
#724=FACE_OUTER_BOUND('',#1270,.T.);
#725=FACE_OUTER_BOUND('',#1271,.T.);
#1235=EDGE_LOOP('',(#6606));
#1236=EDGE_LOOP('',(#6607,#6608,#6609,#6610,#6611,#6612));
#1237=EDGE_LOOP('',(#6613,#6614,#6615,#6616));
#1238=EDGE_LOOP('',(#6617,#6618,#6619,#6620));
#1239=EDGE_LOOP('',(#6621,#6622,#6623,#6624));
#1240=EDGE_LOOP('',(#6625));
#1241=EDGE_LOOP('',(#6626,#6627));
#1242=EDGE_LOOP('',(#6628,#6629,#6630));
#1243=EDGE_LOOP('',(#6631,#6632,#6633,#6634,#6635));
#1244=EDGE_LOOP('',(#6636,#6637,#6638,#6639));
#1245=EDGE_LOOP('',(#6640,#6641,#6642,#6643));
#1246=EDGE_LOOP('',(#6644,#6645,#6646,#6647));
#1247=EDGE_LOOP('',(#6648,#6649,#6650,#6651));
#1248=EDGE_LOOP('',(#6652,#6653,#6654,#6655));
#1249=EDGE_LOOP('',(#6656,#6657,#6658,#6659));
#1250=EDGE_LOOP('',(#6660,#6661,#6662,#6663,#6664,#6665));
#1251=EDGE_LOOP('',(#6666,#6667,#6668,#6669,#6670,#6671));
#1252=EDGE_LOOP('',(#6672,#6673,#6674));
#1253=EDGE_LOOP('',(#6675,#6676,#6677,#6678,#6679,#6680));
#1254=EDGE_LOOP('',(#6681,#6682,#6683,#6684,#6685,#6686));
#1255=EDGE_LOOP('',(#6687,#6688,#6689,#6690));
#1256=EDGE_LOOP('',(#6691,#6692,#6693,#6694));
#1257=EDGE_LOOP('',(#6695,#6696,#6697,#6698));
#1258=EDGE_LOOP('',(#6699,#6700,#6701,#6702));
#1259=EDGE_LOOP('',(#6703,#6704,#6705,#6706));
#1260=EDGE_LOOP('',(#6707,#6708,#6709,#6710,#6711));
#1261=EDGE_LOOP('',(#6712,#6713,#6714,#6715));
#1262=EDGE_LOOP('',(#6716,#6717,#6718,#6719,#6720,#6721,#6722));
#1263=EDGE_LOOP('',(#6723,#6724,#6725));
#1264=EDGE_LOOP('',(#6726,#6727,#6728,#6729,#6730));
#1265=EDGE_LOOP('',(#6731,#6732,#6733,#6734,#6735));
#1266=EDGE_LOOP('',(#6736,#6737,#6738,#6739,#6740));
#1267=EDGE_LOOP('',(#6741,#6742,#6743,#6744,#6745));
#1268=EDGE_LOOP('',(#6746,#6747,#6748,#6749,#6750));
#1269=EDGE_LOOP('',(#6751,#6752,#6753,#6754,#6755));
#1270=EDGE_LOOP('',(#6756,#6757,#6758,#6759,#6760));
#1271=EDGE_LOOP('',(#6761,#6762,#6763));
#1861=CIRCLE('',#9669,3.);
#1862=CIRCLE('',#9671,3.);
#1863=CIRCLE('',#9673,3.);
#1864=CIRCLE('',#9674,3.);
#1865=CIRCLE('',#9676,4.705);
#1866=CIRCLE('',#9678,5.);
#1867=CIRCLE('',#9687,1.5);
#1868=CIRCLE('',#9691,1.5);
#2179=B_SPLINE_CURVE_WITH_KNOTS('',3,(#20178,#20179,#20180,#20181,#20182,
#20183,#20184,#20185,#20186,#20187,#20188,#20189,#20190,#20191,#20192,#20193,
#20194,#20195,#20196,#20197,#20198,#20199,#20200,#20201,#20202,#20203,#20204,
#20205,#20206,#20207,#20208,#20209,#20210,#20211,#20212,#20213,#20214,#20215,
#20216,#20217,#20218,#20219,#20220,#20221,#20222,#20223),.UNSPECIFIED.,
 .T.,.F.,(4,2,2,2,2,2,2,2,2,2,2,2,2,2,2,2,2,2,2,2,2,2,4),(0.,0.0303279803851074,
0.0648320646553547,0.102562075792128,0.126671294216712,0.141186647288206,
0.154035410358203,0.170137123542524,0.200563378583841,0.234595595843345,
0.269428299352715,0.300434782253784,0.331382982474387,0.368306307376294,
0.405848054427407,0.42449623685392,0.437619477079292,0.451067252290898,
0.470635743932431,0.508603340981971,0.544438969378365,0.563834514230334,
0.582682105035748),.UNSPECIFIED.);
#2180=B_SPLINE_CURVE_WITH_KNOTS('',3,(#20226,#20227,#20228,#20229,#20230,
#20231,#20232,#20233,#20234,#20235,#20236,#20237,#20238,#20239,#20240,#20241,
#20242,#20243,#20244,#20245,#20246,#20247,#20248,#20249,#20250,#20251,#20252,
#20253,#20254),.UNSPECIFIED.,.F.,.F.,(4,2,2,2,2,2,2,3,2,2,2,2,2,4),(0.437146516074455,
0.437619477079327,0.451067252290927,0.470635743932452,0.508603340981988,
0.544438969378375,0.563834514230342,0.582682105035755,0.613010085420863,
0.647514169691112,0.685244180827893,0.709353399252473,0.723868752323962,
0.728371798153077),.UNSPECIFIED.);
#2181=B_SPLINE_CURVE_WITH_KNOTS('',3,(#20255,#20256,#20257,#20258,#20259,
#20260,#20261,#20262,#20263,#20264,#20265,#20266,#20267,#20268,#20269,#20270,
#20271,#20272,#20273,#20274,#20275,#20276,#20277,#20278),.UNSPECIFIED.,
 .F.,.F.,(4,2,2,2,2,2,2,2,2,2,2,4),(0.728371798153077,0.736717515393956,
0.752819228578281,0.783245483619599,0.817277700879103,0.852110404388476,
0.883116887289549,0.914065087510156,0.95098841241207,0.988530159463189,
1.00717834188971,1.01982862111021),.UNSPECIFIED.);
#2182=B_SPLINE_CURVE_WITH_KNOTS('',3,(#20311,#20312,#20313,#20314),
 .UNSPECIFIED.,.F.,.F.,(4,4),(0.,0.00439307035085368),.UNSPECIFIED.);
#2183=B_SPLINE_CURVE_WITH_KNOTS('',3,(#20320,#20321,#20322,#20323,#20324,
#20325,#20326,#20327,#20328,#20329),.UNSPECIFIED.,.F.,.F.,(4,2,2,2,4),(5.13627280805781E-5,
0.0320258340472732,0.0612702767974556,0.0930309669729081,0.134040491070964),
 .UNSPECIFIED.);
#2184=B_SPLINE_CURVE_WITH_KNOTS('',3,(#20331,#20332,#20333,#20334,#20335,
#20336,#20337,#20338,#20339,#20340,#20341,#20342,#20343,#20344,#20345,#20346,
#20347,#20348,#20349,#20350,#20351,#20352,#20353,#20354,#20355,#20356,#20357,
#20358,#20359,#20360,#20361,#20362,#20363,#20364,#20365,#20366,#20367,#20368,
#20369,#20370,#20371,#20372,#20373,#20374,#20375,#20376,#20377,#20378,#20379,
#20380,#20381,#20382),.UNSPECIFIED.,.F.,.F.,(4,3,3,3,3,3,3,3,3,3,3,3,3,
3,3,3,3,4),(0.000145335606066559,0.0558438614877374,0.112231630436153,0.148456034280231,
0.227748495028953,0.282789424752488,0.337741461975064,0.401442660385716,
0.446139981200921,0.53876827776481,0.628638367340173,0.701989458203041,
0.775601617992821,0.816653167456479,0.865359231836614,0.925223109102549,
0.98460838252849,1.),.UNSPECIFIED.);
#2185=B_SPLINE_CURVE_WITH_KNOTS('',3,(#20383,#20384,#20385,#20386,#20387,
#20388,#20389,#20390,#20391,#20392,#20393,#20394,#20395,#20396,#20397,#20398),
 .UNSPECIFIED.,.F.,.F.,(4,2,2,2,2,2,2,4),(0.,0.0366659264051676,0.0723720753432845,
0.124708624882515,0.177690395521786,0.229019615948737,0.276645523150972,
0.335263057882293),.UNSPECIFIED.);
#2186=B_SPLINE_CURVE_WITH_KNOTS('',3,(#20401,#20402,#20403,#20404,#20405,
#20406,#20407,#20408,#20409,#20410,#20411,#20412),.UNSPECIFIED.,.F.,.F.,
(4,2,2,2,2,4),(3.49458439059213E-5,0.0453289864597133,0.0881005201250716,
0.109209349263548,0.131675926651336,0.173631899173032),.UNSPECIFIED.);
#2187=B_SPLINE_CURVE_WITH_KNOTS('',3,(#20555,#20556,#20557,#20558,#20559,
#20560,#20561,#20562,#20563,#20564,#20565,#20566,#20567,#20568,#20569,#20570,
#20571,#20572,#20573,#20574,#20575,#20576,#20577,#20578,#20579,#20580,#20581,
#20582,#20583,#20584,#20585,#20586,#20587,#20588,#20589,#20590,#20591,#20592,
#20593,#20594,#20595,#20596,#20597,#20598,#20599,#20600,#20601,#20602,#20603,
#20604,#20605,#20606,#20607,#20608,#20609,#20610,#20611,#20612,#20613,#20614,
#20615,#20616,#20617,#20618,#20619,#20620,#20621,#20622,#20623,#20624,#20625,
#20626,#20627,#20628,#20629,#20630,#20631,#20632,#20633,#20634,#20635,#20636,
#20637,#20638,#20639,#20640,#20641,#20642,#20643,#20644,#20645,#20646,#20647,
#20648,#20649,#20650,#20651,#20652,#20653,#20654,#20655,#20656,#20657,#20658,
#20659,#20660,#20661,#20662,#20663,#20664,#20665,#20666,#20667,#20668,#20669,
#20670,#20671,#20672,#20673,#20674,#20675,#20676,#20677,#20678,#20679,#20680,
#20681,#20682,#20683,#20684,#20685,#20686,#20687,#20688,#20689,#20690,#20691,
#20692,#20693,#20694,#20695,#20696,#20697,#20698,#20699,#20700,#20701,#20702,
#20703,#20704,#20705,#20706,#20707,#20708,#20709,#20710,#20711,#20712,#20713,
#20714,#20715,#20716,#20717,#20718,#20719,#20720,#20721,#20722,#20723,#20724,
#20725,#20726,#20727,#20728,#20729,#20730,#20731,#20732,#20733,#20734,#20735,
#20736,#20737,#20738,#20739,#20740,#20741,#20742,#20743,#20744,#20745,#20746,
#20747,#20748,#20749,#20750,#20751,#20752,#20753,#20754),.UNSPECIFIED.,
 .F.,.F.,(4,2,2,2,2,2,2,2,2,2,2,2,2,2,2,2,2,2,2,2,2,2,2,2,2,2,2,2,2,2,2,
2,2,2,2,2,2,2,2,2,2,2,2,2,2,2,2,2,2,2,2,2,2,2,2,2,2,2,2,2,2,2,2,2,2,2,2,
2,2,2,2,2,2,2,2,2,2,2,2,2,2,2,2,2,2,2,2,2,2,2,2,2,2,2,2,2,2,2,2,4),(7.45212108627149E-5,
0.0390859205350479,0.0725343883639714,0.0923685642265828,0.10913469384073,
0.129155095331907,0.162486409684089,0.180608217655252,0.197291535945613,
0.206770940019813,0.225188684952061,0.243528078049337,0.256462991620191,
0.264518834073687,0.280147599046037,0.296305916680565,0.308456488246771,
0.318005525489979,0.326611674502013,0.343989855479804,0.352023793262373,
0.368259649578705,0.379849408566588,0.394029573187565,0.407680306645622,
0.424415770043147,0.43678227704562,0.450244531707888,0.463053111242432,
0.477324221391811,0.492271306083695,0.509239387041698,0.517031504020095,
0.539706652015012,0.549548685711017,0.563677913026186,0.572928012382314,
0.589291627420903,0.604168007251376,0.616383894352015,0.627484328862961,
0.655655883221415,0.66902740806289,0.683521944564165,0.715231655167139,
0.748094638169843,0.78081393145294,0.820255058267261,0.86511658506511,0.8872313920142,
0.93278922862096,0.970291556017733,1.01383492275163,1.03578068793651,1.05134433691653,
1.07348802880114,1.09404302061058,1.10953987000782,1.12475427757661,1.1409239918375,
1.16865195202472,1.18227448258818,1.20307890941387,1.22478565953238,1.24693285450956,
1.25844545792802,1.2837125731859,1.29455662461225,1.31868739711981,1.33090099941074,
1.34615816441378,1.36164027989683,1.3801960490241,1.40077714225269,1.42078748038377,
1.44154422431501,1.45889752043253,1.47881011912306,1.48990219432189,1.51418923130129,
1.52701547654404,1.53949488816994,1.55641883911018,1.57834720388455,1.60230105640136,
1.6148609138865,1.63693381184042,1.65424351253927,1.68439231036836,1.69912008127496,
1.71980420571561,1.7480963978574,1.79484207024713,1.82938593412522,1.87669821849617,
1.92347052961058,1.97673507695957,2.02673097417545,2.05162657191679,2.07670782789279),
 .UNSPECIFIED.);
#2188=B_SPLINE_CURVE_WITH_KNOTS('',3,(#20757,#20758,#20759,#20760,#20761,
#20762,#20763,#20764,#20765,#20766,#20767,#20768,#20769,#20770,#20771,#20772,
#20773,#20774,#20775,#20776,#20777,#20778,#20779,#20780,#20781,#20782,#20783,
#20784,#20785,#20786,#20787,#20788,#20789,#20790,#20791,#20792,#20793,#20794,
#20795,#20796,#20797,#20798,#20799,#20800,#20801,#20802,#20803,#20804,#20805,
#20806,#20807,#20808,#20809,#20810,#20811,#20812,#20813,#20814,#20815,#20816,
#20817,#20818,#20819,#20820,#20821,#20822,#20823,#20824,#20825,#20826,#20827,
#20828,#20829,#20830,#20831,#20832,#20833,#20834,#20835,#20836,#20837,#20838,
#20839,#20840,#20841,#20842,#20843,#20844,#20845,#20846,#20847,#20848,#20849,
#20850,#20851,#20852,#20853,#20854,#20855,#20856,#20857,#20858,#20859,#20860,
#20861,#20862,#20863,#20864,#20865,#20866,#20867,#20868,#20869,#20870,#20871,
#20872,#20873,#20874),.UNSPECIFIED.,.F.,.F.,(4,2,2,2,2,2,2,2,2,2,2,2,2,
2,2,2,2,2,2,2,2,2,2,2,2,2,2,2,2,2,2,2,2,2,2,2,2,2,2,2,2,2,2,2,2,2,2,2,2,
2,2,2,2,2,2,2,2,2,4),(-1.76933842521691,-1.75674576879776,-1.74490053734257,
-1.73208561542255,-1.72272120633228,-1.70518992653856,-1.69490789137764,
-1.67805988019643,-1.66693268245685,-1.65308325501219,-1.64232441419012,
-1.62057361832964,-1.59364721685683,-1.56003185692642,-1.54329842415155,
-1.52594121987271,-1.49668326282551,-1.46639000558743,-1.44829465608857,
-1.43030111448265,-1.40351884475363,-1.3794702173695,-1.347081159001,-1.33381533931789,
-1.31924278076883,-1.30492051384824,-1.28667377582415,-1.25919462303656,
-1.23249275230696,-1.20410316074078,-1.16947353335439,-1.12643013051659,
-1.10551542910693,-1.06375425104976,-1.02128477547816,-0.980831861829275,
-0.957773368677078,-0.933456655940948,-0.916552189219702,-0.886703502045147,
-0.838519038842251,-0.816226780787853,-0.779667415609276,-0.750538622619109,
-0.722803539353438,-0.684732734627719,-0.63056648173689,-0.582545875778306,
-0.526120615833343,-0.469754166438239,-0.405799756718641,-0.366097308625937,
-0.288199258420126,-0.212956502445796,-0.174214028651596,-0.130497935980871,
-0.0721693074289823,-0.0379539402192462,-3.50852568431468E-5),
 .UNSPECIFIED.);
#2189=B_SPLINE_CURVE_WITH_KNOTS('',3,(#21015,#21016,#21017,#21018,#21019,
#21020),.UNSPECIFIED.,.F.,.F.,(4,2,4),(-0.0184844970402346,-0.00927720086146568,
0.),.UNSPECIFIED.);
#2190=B_SPLINE_CURVE_WITH_KNOTS('',3,(#21022,#21023,#21024,#21025,#21026,
#21027,#21028,#21029,#21030,#21031,#21032,#21033,#21034,#21035,#21036,#21037,
#21038,#21039,#21040,#21041,#21042,#21043,#21044,#21045,#21046,#21047,#21048,
#21049,#21050,#21051,#21052,#21053,#21054,#21055,#21056,#21057,#21058,#21059,
#21060,#21061,#21062,#21063,#21064,#21065,#21066,#21067,#21068,#21069,#21070,
#21071,#21072,#21073),.UNSPECIFIED.,.F.,.F.,(4,2,2,2,2,2,2,2,2,2,2,2,2,
2,2,2,2,2,2,2,2,2,2,2,2,4),(-1.09405986636961,-1.03730632127397,-0.984374802569,
-0.948133535627927,-0.91402589190069,-0.850789144110965,-0.814114574656998,
-0.780501482328998,-0.716513557400044,-0.679267127882597,-0.643435469696746,
-0.583663696479992,-0.54471419772387,-0.506138779451838,-0.461835275143851,
-0.39250853791068,-0.355884669271099,-0.316987624288024,-0.259015545363003,
-0.231144290960428,-0.199057203738863,-0.150397488973068,-0.120980335034911,
-0.0899477105086688,-0.0466030340969419,-5.56419646036315E-5),
 .UNSPECIFIED.);
#2191=B_SPLINE_CURVE_WITH_KNOTS('',3,(#21076,#21077,#21078,#21079,#21080,
#21081,#21082,#21083,#21084,#21085,#21086,#21087,#21088,#21089,#21090,#21091,
#21092,#21093,#21094,#21095,#21096,#21097,#21098,#21099,#21100,#21101,#21102,
#21103,#21104,#21105,#21106,#21107,#21108,#21109,#21110,#21111,#21112,#21113,
#21114,#21115,#21116,#21117,#21118,#21119,#21120,#21121,#21122,#21123,#21124,
#21125,#21126,#21127,#21128,#21129,#21130,#21131,#21132,#21133,#21134,#21135,
#21136,#21137,#21138,#21139,#21140,#21141,#21142,#21143,#21144,#21145,#21146,
#21147,#21148,#21149,#21150,#21151,#21152,#21153,#21154,#21155,#21156,#21157,
#21158,#21159,#21160,#21161,#21162,#21163,#21164,#21165,#21166,#21167,#21168,
#21169,#21170,#21171,#21172,#21173,#21174,#21175,#21176,#21177,#21178,#21179,
#21180,#21181,#21182,#21183,#21184,#21185,#21186,#21187,#21188,#21189,#21190,
#21191,#21192,#21193,#21194,#21195,#21196,#21197,#21198,#21199,#21200,#21201,
#21202,#21203,#21204,#21205,#21206,#21207,#21208,#21209,#21210,#21211,#21212,
#21213,#21214,#21215,#21216,#21217,#21218,#21219,#21220,#21221,#21222,#21223,
#21224,#21225,#21226,#21227,#21228,#21229,#21230,#21231,#21232,#21233,#21234,
#21235,#21236,#21237,#21238,#21239,#21240,#21241,#21242,#21243,#21244,#21245,
#21246,#21247,#21248,#21249,#21250,#21251,#21252,#21253,#21254,#21255,#21256,
#21257,#21258,#21259,#21260,#21261,#21262,#21263,#21264,#21265,#21266,#21267,
#21268,#21269,#21270,#21271,#21272,#21273,#21274,#21275,#21276,#21277,#21278,
#21279,#21280,#21281,#21282,#21283,#21284,#21285,#21286,#21287,#21288,#21289,
#21290,#21291,#21292,#21293,#21294,#21295,#21296,#21297,#21298,#21299,#21300,
#21301,#21302,#21303,#21304,#21305,#21306,#21307,#21308,#21309,#21310,#21311,
#21312,#21313,#21314,#21315,#21316,#21317,#21318,#21319,#21320,#21321,#21322,
#21323,#21324,#21325,#21326,#21327,#21328,#21329),.UNSPECIFIED.,.F.,.F.,
(4,2,2,2,2,2,2,2,2,2,2,2,2,2,2,2,2,2,2,2,2,2,2,2,2,2,2,2,2,2,2,2,2,2,2,
2,2,2,2,2,2,2,2,2,2,2,2,2,2,2,2,2,2,2,2,2,2,2,2,2,2,2,2,2,2,2,2,2,2,2,2,
2,2,2,2,2,2,2,2,2,2,2,2,2,2,2,2,2,2,2,2,2,2,2,2,2,2,2,2,2,2,2,2,2,2,2,2,
2,2,2,2,2,2,2,2,2,2,2,2,2,2,2,2,2,2,2,4),(-2.31862914046342,-2.30598459560142,
-2.29322331448155,-2.26919964602539,-2.23871046157128,-2.20609463722988,
-2.17715977999077,-2.14857178018608,-2.12800173401574,-2.10976412741253,
-2.09678253199906,-2.06436414565108,-2.05021195659004,-2.03710558827847,
-2.02490475911032,-2.01275974712957,-1.98702230972913,-1.97538681221731,
-1.95227026199713,-1.94055624090361,-1.91498597580451,-1.90307437360638,
-1.89286574714465,-1.87531068965113,-1.86433811381829,-1.85060718835371,
-1.83345320402823,-1.82220775146935,-1.80786671595337,-1.79551979175111,
-1.78621940477618,-1.77205815369256,-1.75736766324443,-1.74722923140104,
-1.73487864132895,-1.72037909406407,-1.71062825530799,-1.69720351050645,
-1.68276010187228,-1.6728467018132,-1.65468232035854,-1.64247978973589,
-1.63324908992537,-1.61865169207853,-1.60287432863603,-1.59272290269745,
-1.57124401799536,-1.55901554706166,-1.53874326856615,-1.52983643237255,
-1.51914916776934,-1.49583562913336,-1.48234772897258,-1.46493554956798,
-1.45513129319181,-1.44234818132605,-1.41884037090298,-1.40791211922436,
-1.39089691669365,-1.37873487026916,-1.34705513798498,-1.33325150317816,
-1.31752727667309,-1.29910947364165,-1.26674177398155,-1.24752045398081,
-1.23764981543001,-1.20676151180157,-1.18595570121478,-1.14928178402936,
-1.10487254736548,-1.05929884339584,-1.01376099768513,-0.991553150184975,
-0.94723622571489,-0.901647859959443,-0.863968021765192,-0.823058375200254,
-0.802486538092744,-0.766643131386914,-0.750637145057582,-0.73409787754341,
-0.714972538383972,-0.687593860600446,-0.674119836891209,-0.65541070815958,
-0.642501778422718,-0.616363274107068,-0.602275722486382,-0.591795878439827,
-0.571857089189573,-0.554787342092337,-0.523577187953407,-0.507577460823363,
-0.488587404355769,-0.475906376724585,-0.457344106224095,-0.441767668728689,
-0.429619159785518,-0.409110064596727,-0.398911849538941,-0.388838821593165,
-0.366526384232034,-0.355541293851422,-0.337324434191078,-0.31779737053968,
-0.306781814244162,-0.290837862688885,-0.276447811819492,-0.264989855802201,
-0.24860774289435,-0.233365138216303,-0.223005678297635,-0.208979820090255,
-0.193064202825831,-0.180273554774194,-0.16105706518809,-0.147432461814324,
-0.136032304756679,-0.117900485873948,-0.106267693488742,-0.0858274261946478,
-0.0626305750766336,-0.0507041395934779,-0.0300644165754477,-0.0158174060505365,
-5.54591562635499E-5),.UNSPECIFIED.);
#2192=B_SPLINE_CURVE_WITH_KNOTS('',3,(#21614,#21615,#21616,#21617,#21618,
#21619,#21620,#21621,#21622,#21623,#21624,#21625,#21626,#21627,#21628,#21629,
#21630,#21631,#21632,#21633,#21634,#21635,#21636,#21637,#21638,#21639,#21640,
#21641,#21642,#21643,#21644,#21645,#21646,#21647,#21648,#21649,#21650,#21651,
#21652,#21653,#21654,#21655,#21656,#21657,#21658,#21659,#21660,#21661,#21662,
#21663,#21664,#21665,#21666,#21667,#21668,#21669,#21670,#21671,#21672,#21673,
#21674,#21675,#21676,#21677,#21678,#21679,#21680,#21681,#21682,#21683,#21684,
#21685,#21686,#21687,#21688,#21689,#21690,#21691,#21692,#21693,#21694,#21695,
#21696,#21697,#21698,#21699,#21700,#21701,#21702,#21703,#21704,#21705,#21706,
#21707,#21708,#21709,#21710,#21711,#21712,#21713,#21714,#21715,#21716,#21717,
#21718,#21719,#21720,#21721,#21722,#21723,#21724,#21725,#21726,#21727,#21728,
#21729,#21730,#21731,#21732,#21733,#21734,#21735),.UNSPECIFIED.,.F.,.F.,
(4,2,2,2,2,2,2,2,2,2,2,2,2,2,2,2,2,2,2,2,2,2,2,2,2,2,2,2,2,2,2,2,2,2,2,
2,2,2,2,2,2,2,2,2,2,2,2,2,2,2,2,2,2,2,2,2,2,2,2,2,4),(8.30537880068429E-5,
0.0254958373655499,0.0511669758667031,0.0975715295513944,0.144549119666171,
0.190555985985661,0.237173157637105,0.28220739695801,0.33535113383606,0.396327999244979,
0.470573317964654,0.557317906359429,0.662806278007236,0.782445093948236,
0.910467302271474,1.00941636377096,1.09790968723056,1.1703108289258,1.23501882107797,
1.3004731712299,1.36686574863236,1.43393918358028,1.4996857682952,1.56559133213915,
1.62879053162939,1.703133303482,1.788306343389,1.89158296556634,2.0119211065547,
2.17079601025095,2.38272456897449,2.59465312769801,2.75352803139522,2.87386617238471,
2.97714279456311,3.06231583447097,3.13665860632426,3.19985780581505,3.2657633696595,
3.33150995437481,3.39858338932318,3.46497596672612,3.53043031687846,3.59513830903091,
3.66753945072645,3.75603277418654,3.85498183568668,3.98300404401062,4.10264285995221,
4.20813123160079,4.29487581999634,4.36912113871677,4.4300980041263,4.48324174100491,
4.52827598032626,4.57489315197818,4.62090001829821,4.6678776084135,4.71428216209869,
4.73994899132534,4.76536580002195),.UNSPECIFIED.);
#2193=B_SPLINE_CURVE_WITH_KNOTS('',3,(#21736,#21737,#21738,#21739,#21740,
#21741,#21742,#21743,#21744,#21745,#21746,#21747,#21748,#21749,#21750,#21751,
#21752,#21753,#21754,#21755,#21756,#21757,#21758,#21759,#21760,#21761,#21762,
#21763,#21764,#21765,#21766,#21767,#21768,#21769,#21770,#21771,#21772,#21773,
#21774,#21775,#21776,#21777,#21778,#21779,#21780,#21781,#21782,#21783,#21784,
#21785,#21786,#21787,#21788,#21789,#21790,#21791,#21792,#21793,#21794,#21795,
#21796,#21797,#21798,#21799,#21800,#21801,#21802,#21803,#21804,#21805,#21806,
#21807,#21808,#21809,#21810,#21811,#21812,#21813,#21814,#21815,#21816,#21817,
#21818,#21819,#21820,#21821,#21822,#21823,#21824,#21825,#21826,#21827,#21828,
#21829,#21830,#21831,#21832,#21833,#21834,#21835,#21836,#21837,#21838,#21839,
#21840,#21841,#21842,#21843,#21844,#21845,#21846,#21847,#21848,#21849,#21850,
#21851,#21852,#21853,#21854,#21855,#21856,#21857),.UNSPECIFIED.,.F.,.F.,
(4,2,2,2,2,2,2,2,2,2,2,2,2,2,2,2,2,2,2,2,2,2,2,2,2,2,2,2,2,2,2,2,2,2,2,
2,2,2,2,2,2,2,2,2,2,2,2,2,2,2,2,2,2,2,2,2,2,2,2,2,4),(-4.76536595170222,
-4.73995314110334,-4.71428195744723,-4.66787732213782,-4.62089964939037,
-4.57489270214569,-4.52827544849554,-4.48324112996028,-4.43009729960343,
-4.36912032693738,-4.29487487762162,-4.20813013664478,-4.10264157944498,
-3.98300255306166,-3.85498011954989,-3.75603088400096,-3.66753740488334,
-3.59513613583592,-3.53042802986368,-3.46497356457885,-3.39858087039315,
-3.33150731746439,-3.26576061710252,-3.19985493733199,-3.13665562667562,
-3.06231272405554,-2.97713953433084,-2.87386273049197,-2.75352437783121,
-2.59464919467714,-2.38272026317545,-2.17079133167378,-2.0119161485187,
-1.89157779585674,-1.78830099201675,-1.70312780229116,-1.62878489967036,
-1.5655855890134,-1.49967990924233,-1.43393320888005,-1.3668596559508,-1.3004669617646,
-1.23501249647932,-1.17030439050675,-1.09790312145899,-1.00940964234083,
-0.910460406791192,-0.782437973278634,-0.662798946894652,-0.55731038969403,
-0.470565648716402,-0.396320199399856,-0.335343226733173,-0.282199396375739,
-0.237165077840018,-0.190547824189379,-0.144540876944152,-0.097563204196169,
-0.0511585688862554,-0.0254916578336772,-7.48059887998284E-5),
 .UNSPECIFIED.);
#2194=B_SPLINE_CURVE_WITH_KNOTS('',3,(#22001,#22002,#22003,#22004,#22005,
#22006,#22007,#22008,#22009,#22010,#22011,#22012,#22013,#22014,#22015,#22016,
#22017,#22018,#22019,#22020,#22021,#22022,#22023,#22024,#22025,#22026,#22027,
#22028,#22029,#22030,#22031,#22032,#22033,#22034,#22035,#22036,#22037,#22038,
#22039,#22040,#22041,#22042,#22043,#22044,#22045,#22046,#22047,#22048,#22049,
#22050,#22051,#22052,#22053,#22054,#22055,#22056,#22057,#22058,#22059,#22060,
#22061,#22062,#22063,#22064,#22065,#22066,#22067,#22068,#22069,#22070,#22071,
#22072,#22073,#22074,#22075,#22076,#22077,#22078,#22079,#22080,#22081,#22082,
#22083,#22084,#22085,#22086,#22087,#22088,#22089,#22090,#22091,#22092,#22093,
#22094,#22095,#22096,#22097,#22098,#22099,#22100,#22101,#22102,#22103,#22104,
#22105,#22106,#22107,#22108,#22109,#22110,#22111,#22112,#22113,#22114,#22115,
#22116,#22117,#22118,#22119,#22120,#22121,#22122),.UNSPECIFIED.,.F.,.F.,
(4,2,2,2,2,2,2,2,2,2,2,2,2,2,2,2,2,2,2,2,2,2,2,2,2,2,2,2,2,2,2,2,2,2,2,
2,2,2,2,2,2,2,2,2,2,2,2,2,2,2,2,2,2,2,2,2,2,2,2,2,4),(8.30537880068975E-5,
0.025495837365562,0.0511669758667308,0.0975715295513951,0.144549119666162,
0.190555985985693,0.237173157637078,0.282207396957804,0.33535113383566,
0.396327999244494,0.470573317964095,0.557317906358615,0.662806278005663,
0.782445093944814,0.910467302266539,1.00941636376502,1.09790968722332,1.17031082891732,
1.23501882106856,1.30047317121971,1.36686574862139,1.43393918356847,1.49968576828256,
1.56559133212574,1.62879053161532,1.70313330346716,1.78830634337317,1.89158296554934,
2.01192110653645,2.17079601023056,2.38272456894982,2.59465312766908,2.75352803136314,
2.8738661723502,2.97714279452633,3.0623158344323,3.1366586062841,3.19985780577366,
3.26576336961681,3.33150995433086,3.39858338927791,3.46497596667956,3.53043031683068,
3.59513830898189,3.66753945067584,3.75603277413411,3.85498183563256,3.98300404395421,
4.10264285989329,4.20813123154037,4.29487581993493,4.36912113865456,4.43009800406343,
4.48324174094132,4.52827598026207,4.57489315191348,4.62090001823304,4.66787760834784,
4.71428216203254,4.73995330053361,4.76536606643197),.UNSPECIFIED.);
#2195=B_SPLINE_CURVE_WITH_KNOTS('',3,(#22123,#22124,#22125,#22126,#22127,
#22128,#22129,#22130,#22131,#22132,#22133,#22134,#22135,#22136,#22137,#22138,
#22139,#22140,#22141,#22142,#22143,#22144,#22145,#22146,#22147,#22148,#22149,
#22150,#22151,#22152,#22153,#22154,#22155,#22156,#22157,#22158,#22159,#22160,
#22161,#22162,#22163,#22164,#22165,#22166,#22167,#22168,#22169,#22170,#22171,
#22172,#22173,#22174,#22175,#22176,#22177,#22178,#22179,#22180,#22181,#22182,
#22183,#22184,#22185,#22186,#22187,#22188,#22189,#22190,#22191,#22192,#22193,
#22194,#22195,#22196,#22197,#22198,#22199,#22200,#22201,#22202,#22203,#22204,
#22205,#22206,#22207,#22208,#22209,#22210,#22211,#22212,#22213,#22214,#22215,
#22216,#22217,#22218,#22219,#22220,#22221,#22222,#22223,#22224,#22225,#22226,
#22227,#22228,#22229,#22230,#22231,#22232,#22233,#22234,#22235,#22236,#22237,
#22238,#22239,#22240,#22241,#22242,#22243,#22244),.UNSPECIFIED.,.F.,.F.,
(4,2,2,2,2,2,2,2,2,2,2,2,2,2,2,2,2,2,2,2,2,2,2,2,2,2,2,2,2,2,2,2,2,2,2,
2,2,2,2,2,2,2,2,2,2,2,2,2,2,2,2,2,2,2,2,2,2,2,2,2,4),(-4.76536606643129,
-4.73995330053298,-4.71428216203189,-4.66787760834723,-4.62090001823246,
-4.57489315191293,-4.52827598026155,-4.48324174094082,-4.43009800406296,
-4.36912113865412,-4.29487581993452,-4.20813123154001,-4.10264285989297,
-3.98300404395383,-3.85498183563211,-3.75603277413363,-3.66753945067534,
-3.59513830898134,-3.53043031683011,-3.46497596667895,-3.39858338927727,
-3.33150995433019,-3.26576336961609,-3.19985780577291,-3.13665860628333,
-3.06231583443149,-2.97714279452547,-2.8738661723493,-2.75352803136218,
-2.59465312766806,-2.38272456894879,-2.17079601022952,-2.01192110653546,
-1.89158296554841,-1.78830634337229,-1.70313330346632,-1.62879053161452,
-1.56559133212497,-1.49968576828183,-1.43393918356779,-1.36686574862076,
-1.30047317121913,-1.23501882106803,-1.17031082891684,-1.09790968722292,
-1.00941636376468,-0.910467302266278,-0.782445093944685,-0.662806278005648,
-0.557317906358621,-0.470573317964106,-0.396327999244519,-0.33535113383569,
-0.282207396957838,-0.237173157637114,-0.190555985985732,-0.144549119666206,
-0.0975715295514422,-0.05116697586678,-0.0254958373655863,-8.30537880621146E-5),
 .UNSPECIFIED.);
#2196=B_SPLINE_CURVE_WITH_KNOTS('',3,(#22388,#22389,#22390,#22391,#22392,
#22393,#22394,#22395,#22396,#22397,#22398,#22399,#22400,#22401,#22402,#22403,
#22404,#22405,#22406,#22407,#22408,#22409,#22410,#22411,#22412,#22413,#22414,
#22415,#22416,#22417,#22418,#22419,#22420,#22421,#22422,#22423,#22424,#22425,
#22426,#22427,#22428,#22429,#22430,#22431,#22432,#22433,#22434,#22435,#22436,
#22437,#22438,#22439,#22440,#22441,#22442,#22443,#22444,#22445,#22446,#22447,
#22448,#22449,#22450,#22451,#22452,#22453,#22454,#22455,#22456,#22457,#22458,
#22459,#22460,#22461,#22462,#22463,#22464,#22465,#22466,#22467,#22468,#22469,
#22470,#22471,#22472,#22473,#22474,#22475,#22476,#22477,#22478,#22479,#22480,
#22481,#22482,#22483,#22484,#22485,#22486,#22487,#22488,#22489,#22490,#22491,
#22492,#22493,#22494,#22495,#22496,#22497,#22498,#22499,#22500,#22501,#22502,
#22503,#22504,#22505,#22506,#22507,#22508,#22509),.UNSPECIFIED.,.F.,.F.,
(4,2,2,2,2,2,2,2,2,2,2,2,2,2,2,2,2,2,2,2,2,2,2,2,2,2,2,2,2,2,2,2,2,2,2,
2,2,2,2,2,2,2,2,2,2,2,2,2,2,2,2,2,2,2,2,2,2,2,2,2,4),(8.30537880269274E-5,
0.0254958373655947,0.0511669758667937,0.0975715295514548,0.14454911966622,
0.190555985985725,0.237173157637119,0.28220739695796,0.335351133835972,
0.396327999244821,0.470573317964426,0.557317906358994,0.662806278006377,
0.782445093946579,0.910467302269029,1.00941636376802,1.09790968722708,1.17031082892178,
1.23501882107348,1.30047317122506,1.36686574862723,1.43393918357483,1.49968576828938,
1.56559133213308,1.62879053162317,1.70313330347564,1.78830634338255,1.89158296555981,
2.01192110654796,2.17079601024335,2.38272456896422,2.59465312768512,2.75352803137944,
2.87386617236633,2.97714279454242,3.06231583444839,3.1366586063001,3.19985780578957,
3.26576336963271,3.33150995434681,3.3985833892939,3.46497596669554,3.53043031684666,
3.59513830899801,3.66753945069234,3.75603277415084,3.85498183564909,3.9830040439707,
4.1026428599102,4.20813123155683,4.29487581995069,4.36912113866951,4.43009800407772,
4.48324174095536,4.52827598027589,4.57489315192683,4.62090001824586,4.66787760836021,
4.71428216204449,4.73995330054531,4.76536606644342),.UNSPECIFIED.);
#2197=B_SPLINE_CURVE_WITH_KNOTS('',3,(#22510,#22511,#22512,#22513,#22514,
#22515,#22516,#22517,#22518,#22519,#22520,#22521,#22522,#22523,#22524,#22525,
#22526,#22527,#22528,#22529,#22530,#22531,#22532,#22533,#22534,#22535,#22536,
#22537,#22538,#22539,#22540,#22541,#22542,#22543,#22544,#22545,#22546,#22547,
#22548,#22549,#22550,#22551,#22552,#22553,#22554,#22555,#22556,#22557,#22558,
#22559,#22560,#22561,#22562,#22563,#22564,#22565,#22566,#22567,#22568,#22569,
#22570,#22571,#22572,#22573,#22574,#22575,#22576,#22577,#22578,#22579,#22580,
#22581,#22582,#22583,#22584,#22585,#22586,#22587,#22588,#22589,#22590,#22591,
#22592,#22593,#22594,#22595,#22596,#22597,#22598,#22599,#22600,#22601,#22602,
#22603,#22604,#22605,#22606,#22607,#22608,#22609,#22610,#22611,#22612,#22613,
#22614,#22615,#22616,#22617,#22618,#22619,#22620,#22621,#22622,#22623,#22624,
#22625,#22626,#22627,#22628,#22629,#22630,#22631),.UNSPECIFIED.,.F.,.F.,
(4,2,2,2,2,2,2,2,2,2,2,2,2,2,2,2,2,2,2,2,2,2,2,2,2,2,2,2,2,2,2,2,2,2,2,
2,2,2,2,2,2,2,2,2,2,2,2,2,2,2,2,2,2,2,2,2,2,2,2,2,4),(-4.76536606648679,
-4.73995330058825,-4.71428216208692,-4.66787760840187,-4.62090001828672,
-4.57489315196683,-4.52827598031504,-4.48324174099382,-4.43009800411536,
-4.369121138706,-4.29487581998578,-4.20813123159048,-4.10264285994218,-3.98300404400089,
-3.85498183567728,-3.75603277417739,-3.66753945071753,-3.59513830902217,
-3.53043031686988,-3.46497596671772,-3.39858338931495,-3.33150995436675,
-3.26576336965161,-3.19985780580732,-3.13665860631666,-3.06231583446353,
-2.97714279455585,-2.87386617237767,-2.75352803138844,-2.59465312769161,
-2.38272456896879,-2.17079601024594,-2.01192110655013,-1.8915829655621,
-1.78830634338503,-1.70313330347825,-1.62879053162583,-1.56559133213577,
-1.499685768292,-1.43393918357727,-1.36686574862954,-1.30047317122726,-1.23501882107553,
-1.17031082892357,-1.09790968722854,-1.00941636376919,-0.910467302270004,
-0.78244509394716,-0.662806278006525,-0.557317906358945,-0.470573317964312,
-0.396327999244839,-0.335351133836078,-0.282207396957964,-0.237173157637031,
-0.19055598598568,-0.144549119666231,-0.0975715295514552,-0.0511669758667642,
-0.0254958373655805,-8.30537880556699E-5),.UNSPECIFIED.);
#2198=B_SPLINE_CURVE_WITH_KNOTS('',3,(#22774,#22775,#22776,#22777,#22778,
#22779),.UNSPECIFIED.,.F.,.F.,(4,2,4),(-0.0116317960480669,-0.00585615791721894,
-8.47905377083857E-5),.UNSPECIFIED.);
#2199=B_SPLINE_CURVE_WITH_KNOTS('',3,(#22780,#22781,#22782,#22783,#22784,
#22785,#22786,#22787,#22788,#22789,#22790,#22791,#22792,#22793,#22794,#22795,
#22796,#22797,#22798,#22799,#22800,#22801,#22802,#22803,#22804,#22805,#22806,
#22807,#22808,#22809,#22810,#22811,#22812,#22813,#22814,#22815,#22816,#22817,
#22818,#22819,#22820,#22821,#22822,#22823,#22824,#22825,#22826,#22827,#22828,
#22829,#22830,#22831,#22832,#22833,#22834,#22835,#22836,#22837,#22838,#22839,
#22840,#22841,#22842,#22843,#22844,#22845,#22846,#22847,#22848,#22849,#22850,
#22851,#22852,#22853,#22854,#22855,#22856,#22857,#22858,#22859,#22860,#22861,
#22862,#22863,#22864,#22865,#22866,#22867,#22868,#22869,#22870,#22871,#22872,
#22873,#22874,#22875,#22876,#22877,#22878,#22879,#22880,#22881,#22882,#22883,
#22884,#22885,#22886,#22887,#22888,#22889,#22890,#22891,#22892,#22893,#22894,
#22895,#22896,#22897,#22898,#22899,#22900,#22901),.UNSPECIFIED.,.F.,.F.,
(4,2,2,2,2,2,2,2,2,2,2,2,2,2,2,2,2,2,2,2,2,2,2,2,2,2,2,2,2,2,2,2,2,2,2,
2,2,2,2,2,2,2,2,2,2,2,2,2,2,2,2,2,2,2,2,2,2,2,2,2,4),(8.23445128364946E-5,
0.0254955919483662,0.0511664822196668,0.097571040701871,0.144548635673389,
0.190555506749416,0.237172683220333,0.282206927196841,0.335350669568886,
0.396327541281621,0.470572867676824,0.557317465039227,0.662805847592082,
0.782444675900308,0.910466897457627,1.00941596918587,1.0979093017932,1.17031045097264,
1.23501844981379,1.30047280673184,1.36686539099743,1.43393883287884,1.49968542438998,
1.56559099504675,1.62879020107028,1.70313298060813,1.78830602931986,1.89158266217341,
2.0119208156019,2.17079573572116,2.3827243163491,2.59465289697705,2.75352781709642,
2.87386597052503,2.97714260337883,3.06231565209077,3.13665843162885,3.19985763765255,
3.26576320830941,3.33150979982066,3.39858324170221,3.46497582596794,3.53043018288608,
3.59513818172725,3.66753933090672,3.75603266351411,3.85498173524235,3.98300395679958,
4.10264278510785,4.20813116766099,4.2948757650237,4.36912109141912,4.43009796313204,
4.48324170550436,4.5282759494811,4.57489312595195,4.6208999970278,4.6678775919993,
4.71428215048147,4.73995329163655,4.76536606016219),.UNSPECIFIED.);
#2200=B_SPLINE_CURVE_WITH_KNOTS('',3,(#22902,#22903,#22904,#22905,#22906,
#22907,#22908,#22909,#22910,#22911,#22912,#22913,#22914,#22915,#22916,#22917,
#22918,#22919,#22920,#22921,#22922,#22923,#22924,#22925,#22926,#22927,#22928,
#22929,#22930,#22931,#22932,#22933,#22934,#22935,#22936,#22937,#22938,#22939,
#22940,#22941,#22942,#22943,#22944,#22945,#22946,#22947,#22948,#22949,#22950,
#22951,#22952,#22953,#22954,#22955,#22956,#22957,#22958,#22959,#22960,#22961,
#22962,#22963,#22964,#22965,#22966,#22967,#22968,#22969,#22970,#22971,#22972,
#22973,#22974,#22975,#22976,#22977,#22978,#22979,#22980,#22981,#22982,#22983,
#22984,#22985,#22986,#22987,#22988,#22989,#22990,#22991,#22992,#22993,#22994,
#22995,#22996,#22997,#22998,#22999,#23000,#23001,#23002,#23003,#23004,#23005,
#23006,#23007,#23008,#23009,#23010,#23011,#23012,#23013,#23014,#23015,#23016,
#23017,#23018,#23019,#23020,#23021,#23022,#23023),.UNSPECIFIED.,.F.,.F.,
(4,2,2,2,2,2,2,2,2,2,2,2,2,2,2,2,2,2,2,2,2,2,2,2,2,2,2,2,2,2,2,2,2,2,2,
2,2,2,2,2,2,2,2,2,2,2,2,2,2,2,2,2,2,2,2,2,2,2,2,2,4),(-4.76536629622447,
-4.73995309969356,-4.71428216203548,-4.66787760835079,-4.62090001823604,
-4.57489315191641,-4.528275980265,-4.48324174094435,-4.43009800406656,-4.36912113865791,
-4.29487581993855,-4.20813123154422,-4.10264285989725,-3.98300404395784,
-3.85498183563605,-3.75603277413762,-3.66753945067915,-3.59513830898487,
-3.53043031683354,-3.46497596668246,-3.39858338928084,-3.3315099543338,
-3.26576336961984,-3.19985780577669,-3.136658606287,-3.06231583443505,-2.97714279452891,
-2.87386617235258,-2.75352803136521,-2.59465312767118,-2.3827245689534,
-2.17079601023561,-2.01192110654139,-1.89158296555381,-1.78830634337716,
-1.70313330347075,-1.62879053161852,-1.56559133212861,-1.49968576828534,
-1.43393918357123,-1.36686574862399,-1.30047317122219,-1.23501882107098,
-1.17031082891958,-1.09790968722523,-1.00941636376664,-0.91046730226815,
-0.782445093946358,-0.662806278006812,-0.557317906359464,-0.470573317964745,
-0.396327999245099,-0.335351133836203,-0.282207396958087,-0.237173157637164,
-0.190555985985781,-0.144549119666305,-0.0975715295515277,-0.0511669758668496,
-0.0254958373656227,-8.30537880558869E-5),.UNSPECIFIED.);
#2201=B_SPLINE_CURVE_WITH_KNOTS('',3,(#23030,#23031,#23032,#23033,#23034,
#23035),.UNSPECIFIED.,.F.,.F.,(4,2,4),(-0.0385635633195077,-0.0192648014145305,
-5.6512677524232E-5),.UNSPECIFIED.);
#2202=B_SPLINE_CURVE_WITH_KNOTS('',3,(#23036,#23037,#23038,#23039,#23040,
#23041),.UNSPECIFIED.,.F.,.F.,(4,2,4),(-0.020013276506786,-0.010090500778054,
-1.26246806509996E-5),.UNSPECIFIED.);
#2203=B_SPLINE_CURVE_WITH_KNOTS('',3,(#23044,#23045,#23046,#23047,#23048,
#23049,#23050,#23051,#23052,#23053),.UNSPECIFIED.,.F.,.F.,(4,2,2,2,4),(-0.164908287572566,
-0.122123473574902,-0.0806835746227668,-0.039806081275496,-5.30404670007887E-5),
 .UNSPECIFIED.);
#2204=B_SPLINE_CURVE_WITH_KNOTS('',3,(#23055,#23056,#23057,#23058),
 .UNSPECIFIED.,.F.,.F.,(4,4),(-0.00327039655086957,0.),.UNSPECIFIED.);
#2205=B_SPLINE_CURVE_WITH_KNOTS('',3,(#23202,#23203,#23204,#23205,#23206,
#23207,#23208,#23209,#23210,#23211,#23212,#23213,#23214,#23215,#23216,#23217,
#23218,#23219,#23220,#23221,#23222,#23223,#23224,#23225,#23226,#23227,#23228,
#23229,#23230,#23231,#23232,#23233,#23234,#23235,#23236,#23237,#23238,#23239,
#23240,#23241,#23242,#23243,#23244,#23245,#23246,#23247,#23248,#23249,#23250,
#23251,#23252,#23253,#23254,#23255,#23256,#23257,#23258,#23259,#23260,#23261,
#23262,#23263,#23264,#23265,#23266,#23267,#23268,#23269,#23270,#23271,#23272,
#23273,#23274,#23275,#23276,#23277,#23278,#23279,#23280,#23281,#23282,#23283,
#23284,#23285,#23286,#23287,#23288,#23289,#23290,#23291,#23292,#23293,#23294,
#23295,#23296,#23297,#23298,#23299,#23300,#23301,#23302,#23303,#23304,#23305,
#23306,#23307,#23308,#23309,#23310,#23311,#23312,#23313,#23314,#23315,#23316,
#23317,#23318,#23319,#23320,#23321,#23322,#23323,#23324,#23325,#23326,#23327,
#23328,#23329,#23330,#23331,#23332,#23333,#23334,#23335,#23336,#23337,#23338,
#23339,#23340,#23341,#23342,#23343,#23344,#23345,#23346,#23347,#23348,#23349,
#23350,#23351,#23352,#23353,#23354,#23355,#23356,#23357,#23358,#23359,#23360,
#23361,#23362,#23363,#23364,#23365,#23366,#23367,#23368,#23369,#23370,#23371,
#23372,#23373,#23374,#23375,#23376,#23377,#23378,#23379,#23380,#23381,#23382,
#23383),.UNSPECIFIED.,.F.,.F.,(4,2,2,2,2,2,2,2,2,2,2,2,2,2,2,2,2,2,2,2,
2,2,2,2,2,2,2,2,2,2,2,2,2,2,2,2,2,2,2,2,2,2,2,2,2,2,2,2,2,2,2,2,2,2,2,2,
2,2,2,2,2,2,2,2,2,2,2,2,2,2,2,2,2,2,2,2,2,2,2,2,2,2,2,2,2,2,2,2,2,2,4),
(-2.59382312359622,-2.56809909206607,-2.54791923390964,-2.51910185607888,
-2.50034924577938,-2.46359383453845,-2.44228542443783,-2.40669510295705,
-2.38725922606837,-2.35093961748984,-2.32890149074397,-2.29239847801421,
-2.27292633852247,-2.23609702873241,-2.21402640049839,-2.17733101201315,
-2.15768968532709,-2.12058782546055,-2.09831665072369,-2.06132017512561,
-2.04151153117669,-2.00410711813897,-1.98164874928756,-1.94433785593902,
-1.92436895247648,-1.88665456227707,-1.86401301910331,-1.82639412910864,
-1.80626110387503,-1.76824586383648,-1.7454134243349,-1.70746632183097,
-1.68717332827363,-1.64888670526784,-1.62585024949674,-1.58750854158364,
-1.56707629965118,-1.52867376524863,-1.50537210168194,-1.46632826658595,
-1.44585935678816,-1.40809290140965,-1.3842352254204,-1.34299194673546,
-1.32298293946475,-1.29075419136106,-1.25234706644214,-1.23077326808129,
-1.19286916386442,-1.16895424934302,-1.13063711273809,-1.10923927510981,
-1.07184448765126,-1.04819507852277,-1.0102014896849,-0.989011098243588,
-0.952022048741237,-0.928617115515581,-0.890994268266284,-0.870016399552206,
-0.833407705734039,-0.810240713299895,-0.772995938467394,-0.752229959132093,
-0.715993811809521,-0.693062394391416,-0.65619295215658,-0.635637857528421,
-0.599765415733702,-0.577063393911802,-0.540570727917672,-0.520220615948578,
-0.484721518808244,-0.46225404518635,-0.426125838650698,-0.405988720282876,
-0.370840574739169,-0.34861332772549,-0.312828499163541,-0.29289941060862,
-0.258015550215702,-0.235878653318305,-0.200645947107353,-0.18079872486045,
-0.14688892260254,-0.125531840866317,-0.0899005543185674,-0.0708164474537418,
-0.0422875992108556,-0.0109151062078881,-4.06978878030363E-5),
 .UNSPECIFIED.);
#2206=B_SPLINE_CURVE_WITH_KNOTS('',3,(#23384,#23385,#23386,#23387,#23388,
#23389,#23390,#23391,#23392,#23393,#23394,#23395,#23396,#23397,#23398,#23399,
#23400,#23401,#23402,#23403,#23404,#23405,#23406,#23407,#23408,#23409,#23410,
#23411,#23412,#23413,#23414,#23415,#23416,#23417,#23418,#23419,#23420,#23421,
#23422,#23423,#23424,#23425,#23426,#23427,#23428,#23429,#23430,#23431,#23432,
#23433,#23434,#23435,#23436,#23437,#23438,#23439,#23440,#23441,#23442,#23443,
#23444,#23445),.UNSPECIFIED.,.F.,.F.,(4,2,2,2,2,2,2,2,2,2,2,2,2,2,2,2,2,
2,2,2,2,2,2,2,2,2,2,2,2,2,4),(3.71452156639363E-5,0.018383146637255,0.0405642397108187,
0.0668325597898111,0.111436908431686,0.126394165236214,0.15274397121657,
0.178584594200384,0.215756491831179,0.233810618177999,0.252791145534099,
0.282553240098289,0.311403566815716,0.338930071939597,0.357138036654115,
0.385287554485539,0.412804972902094,0.43983249965415,0.4635752087772,0.479766666968338,
0.500014603141655,0.528593762245753,0.559905689917596,0.578104831901803,
0.599380635704931,0.630875077930314,0.656634519607673,0.683634545887361,
0.699020384949516,0.735639212358386,0.769952845650509),.UNSPECIFIED.);
#2207=B_SPLINE_CURVE_WITH_KNOTS('',3,(#23588,#23589,#23590,#23591,#23592,
#23593,#23594,#23595,#23596,#23597,#23598,#23599,#23600,#23601,#23602,#23603,
#23604,#23605,#23606,#23607,#23608,#23609,#23610,#23611,#23612,#23613,#23614,
#23615,#23616,#23617,#23618,#23619,#23620,#23621,#23622,#23623,#23624,#23625,
#23626,#23627,#23628,#23629,#23630,#23631,#23632,#23633,#23634,#23635,#23636,
#23637,#23638,#23639),.UNSPECIFIED.,.F.,.F.,(4,2,2,2,2,2,2,2,2,2,2,2,2,
2,2,2,2,2,2,2,2,2,2,2,2,4),(-0.949553103265687,-0.906923078453489,-0.866427431983837,
-0.832934013363288,-0.799266013989078,-0.750746029004779,-0.70890633730406,
-0.678129159719416,-0.648036604752675,-0.612823612183411,-0.578073771721634,
-0.53409955835586,-0.500240107263163,-0.466498951022295,-0.429736799555293,
-0.373388222676778,-0.338335060909048,-0.302283409606239,-0.272030647531648,
-0.24247187701457,-0.198686709372544,-0.149970580195427,-0.114177073472312,
-0.0775700325473158,-0.0396702823667157,-5.56419586003635E-5),
 .UNSPECIFIED.);
#2208=B_SPLINE_CURVE_WITH_KNOTS('',3,(#23782,#23783,#23784,#23785,#23786,
#23787,#23788,#23789,#23790,#23791,#23792,#23793,#23794,#23795,#23796,#23797,
#23798,#23799,#23800,#23801,#23802,#23803,#23804,#23805,#23806,#23807,#23808,
#23809,#23810,#23811,#23812,#23813,#23814,#23815,#23816,#23817,#23818,#23819,
#23820,#23821,#23822,#23823,#23824,#23825,#23826,#23827,#23828,#23829,#23830,
#23831,#23832,#23833,#23834,#23835,#23836,#23837,#23838,#23839,#23840,#23841,
#23842,#23843,#23844,#23845,#23846,#23847,#23848,#23849,#23850,#23851,#23852,
#23853,#23854,#23855,#23856,#23857,#23858,#23859,#23860,#23861,#23862,#23863,
#23864,#23865,#23866,#23867,#23868,#23869,#23870,#23871,#23872,#23873,#23874,
#23875,#23876,#23877,#23878,#23879,#23880,#23881,#23882,#23883,#23884,#23885,
#23886,#23887,#23888,#23889,#23890,#23891,#23892,#23893,#23894,#23895,#23896,
#23897,#23898,#23899,#23900,#23901,#23902,#23903,#23904,#23905,#23906,#23907,
#23908,#23909,#23910,#23911,#23912,#23913,#23914,#23915,#23916,#23917,#23918,
#23919,#23920,#23921,#23922,#23923,#23924,#23925,#23926,#23927,#23928,#23929,
#23930,#23931,#23932,#23933,#23934,#23935,#23936,#23937,#23938,#23939,#23940,
#23941,#23942,#23943,#23944,#23945,#23946,#23947,#23948,#23949,#23950,#23951,
#23952,#23953,#23954,#23955,#23956,#23957,#23958,#23959,#23960,#23961,#23962,
#23963,#23964,#23965),.UNSPECIFIED.,.F.,.F.,(4,2,2,2,2,2,2,2,2,2,2,2,2,
2,2,2,2,2,2,2,2,2,2,2,2,2,2,2,2,2,2,2,2,2,2,2,2,2,2,2,2,2,2,2,2,2,2,2,2,
2,2,2,2,2,2,2,2,2,2,2,2,2,2,2,2,2,2,2,2,2,2,2,2,2,2,2,2,2,2,2,2,2,2,2,2,
2,2,2,2,2,2,4),(-2.59123053346005,-2.56554791306885,-2.5453719157918,-2.51664536202888,
-2.4979272184796,-2.46123935800588,-2.4399701154689,-2.40444522219546,-2.38504506442642,
-2.34879218067922,-2.32679457228015,-2.29035871364016,-2.27092234335711,
-2.23416057794242,-2.21213057161506,-2.17550291691656,-2.15589759275248,
-2.11886322652973,-2.09663324953121,-2.05970612839742,-2.03993342751461,
-2.00259445787734,-1.98017860959789,-1.94294268966605,-1.92300829110486,
-1.88534761025334,-1.86275354289858,-1.82523398778967,-1.80512758745354,
-1.7671085292704,-1.74434570998078,-1.70661417579985,-1.68630796422811,
-1.6477334822438,-1.62487351397267,-1.58731784522435,-1.56667351509398,
-1.52656870737691,-1.50396763108559,-1.46858519930174,-1.44687021778233,
-1.41609830641339,-1.38781739596686,-1.36318087074456,-1.3319839559769,
-1.30633301324762,-1.27148566807694,-1.24636686706974,-1.21848731795896,
-1.19235118508901,-1.16802264402101,-1.13083394326271,-1.10959551436729,
-1.07173452508517,-1.04799931079223,-1.0102484851039,-0.989093753270532,
-0.95200616560291,-0.928584032070876,-0.891015553096991,-0.87004651572887,
-0.833418504136608,-0.810249040962625,-0.773017999631342,-0.752255039993863,
-0.716016661261408,-0.693085938451044,-0.656221436670924,-0.635668095014566,
-0.599797092346128,-0.577096436314295,-0.540606791511633,-0.520258147978269,
-0.484761262636764,-0.462295287128823,-0.426169667909789,-0.406033944974079,
-0.370888159493564,-0.348662426167541,-0.312880073138577,-0.292952353160038,
-0.258070871960243,-0.235935489472284,-0.200705201839718,-0.180859339822398,
-0.146951858120951,-0.125596238893428,-0.0899673941394749,-0.0708845946511137,
-0.0423960687609541,-0.0111460198812575,-0.000107286410718428),
 .UNSPECIFIED.);
#2209=B_SPLINE_CURVE_WITH_KNOTS('',3,(#23967,#23968,#23969,#23970,#23971,
#23972,#23973,#23974,#23975,#23976,#23977,#23978,#23979,#23980,#23981,#23982,
#23983,#23984,#23985,#23986,#23987,#23988,#23989,#23990,#23991,#23992,#23993,
#23994,#23995,#23996,#23997,#23998,#23999,#24000,#24001,#24002,#24003,#24004,
#24005,#24006,#24007,#24008,#24009,#24010,#24011,#24012,#24013,#24014,#24015,
#24016),.UNSPECIFIED.,.F.,.F.,(4,2,2,2,2,2,2,2,2,2,2,2,2,2,2,2,2,2,2,2,
2,2,2,2,4),(-0.956982439280623,-0.903526122456605,-0.854507497013016,-0.826934563946404,
-0.799146057249082,-0.74241914188856,-0.714801687201639,-0.686583728369467,
-0.629857984674878,-0.602328820691834,-0.574130057528638,-0.517525223454158,
-0.478071053229473,-0.434312794595821,-0.37788167184512,-0.351722969094686,
-0.322816305907384,-0.266404182629574,-0.239982209276222,-0.194476830584044,
-0.150231700054167,-0.115576342024155,-0.0803424134121,-0.0412201593161153,
-5.56420009251838E-5),.UNSPECIFIED.);
#2210=B_SPLINE_CURVE_WITH_KNOTS('',3,(#24301,#24302,#24303,#24304,#24305,
#24306,#24307,#24308,#24309,#24310,#24311,#24312,#24313,#24314,#24315,#24316,
#24317,#24318,#24319,#24320,#24321,#24322,#24323,#24324,#24325,#24326,#24327,
#24328,#24329,#24330,#24331,#24332,#24333,#24334,#24335,#24336,#24337,#24338,
#24339,#24340,#24341,#24342,#24343,#24344,#24345,#24346,#24347,#24348,#24349,
#24350,#24351,#24352,#24353,#24354,#24355,#24356,#24357,#24358,#24359,#24360,
#24361,#24362,#24363,#24364,#24365,#24366,#24367,#24368,#24369,#24370,#24371,
#24372,#24373,#24374,#24375,#24376,#24377,#24378,#24379,#24380,#24381,#24382,
#24383,#24384,#24385,#24386,#24387,#24388,#24389,#24390,#24391,#24392,#24393,
#24394,#24395,#24396,#24397,#24398,#24399,#24400,#24401,#24402,#24403,#24404,
#24405,#24406,#24407,#24408,#24409,#24410,#24411,#24412,#24413,#24414,#24415,
#24416,#24417,#24418,#24419,#24420,#24421,#24422,#24423,#24424,#24425,#24426,
#24427,#24428,#24429,#24430,#24431,#24432,#24433,#24434,#24435,#24436,#24437,
#24438,#24439,#24440,#24441,#24442,#24443,#24444,#24445,#24446,#24447,#24448,
#24449,#24450,#24451,#24452,#24453,#24454,#24455,#24456,#24457,#24458,#24459,
#24460,#24461,#24462,#24463,#24464,#24465,#24466,#24467,#24468,#24469,#24470,
#24471,#24472,#24473,#24474,#24475,#24476,#24477,#24478,#24479,#24480,#24481,
#24482,#24483,#24484),.UNSPECIFIED.,.F.,.F.,(4,2,2,2,2,2,2,2,2,2,2,2,2,
2,2,2,2,2,2,2,2,2,2,2,2,2,2,2,2,2,2,2,2,2,2,2,2,2,2,2,2,2,2,2,2,2,2,2,2,
2,2,2,2,2,2,2,2,2,2,2,2,2,2,2,2,2,2,2,2,2,2,2,2,2,2,2,2,2,2,2,2,2,2,2,2,
2,2,2,2,2,2,4),(-2.59926568599725,-2.57341790284738,-2.55311215565756,-2.52420086050638,
-2.50536234343823,-2.46843855566556,-2.44703252902056,-2.4112791597983,
-2.391754247624,-2.35526827028152,-2.33312917976257,-2.29645891621898,-2.27689758284438,
-2.23989962259838,-2.21772786179071,-2.18086423847728,-2.16113297812973,
-2.12386146986842,-2.10148814969433,-2.06432157510582,-2.04442239771826,
-2.00684813433544,-1.98428631780977,-1.94680159503098,-1.92674221101307,
-1.88886214023063,-1.86611421132941,-1.82830927241362,-1.80808872880043,
-1.76993282004507,-1.74698320390566,-1.70879753274252,-1.68843379724343,
-1.65012993509938,-1.62692839119727,-1.58810546149191,-1.56768405599013,
-1.52985794423679,-1.50616290607375,-1.47839724920395,-1.45176005974334,
-1.42617681964575,-1.39187166363256,-1.36625834747285,-1.33310974750308,
-1.307442980506,-1.27425765223016,-1.24797027958099,-1.2221641264784,-1.19225399591173,
-1.16784392150644,-1.13087222960183,-1.10966347390913,-1.07171391025553,
-1.04796213922683,-1.01025663207545,-0.989108333184153,-0.952001711293397,
-0.928576033211906,-0.891017281638817,-0.870049615157352,-0.833417556059424,
-0.81024734024633,-0.773018372760037,-0.752255709310832,-0.71601645648305,
-0.693085571189003,-0.656221517262033,-0.635668239582674,-0.599797048122477,
-0.577096356996304,-0.540606808908221,-0.520258179190347,-0.484761253088374,
-0.46229527000396,-0.426169671671616,-0.406033951720906,-0.370888157427394,
-0.348662422463881,-0.312880073953667,-0.292952354619784,-0.258070871518592,
-0.235935488676309,-0.200705202010143,-0.180859340129984,-0.14695185802523,
-0.125596238723843,-0.0899673941804166,-0.0708845947225205,-0.0423960687560085,
-0.011146019861744,-0.000107286410493566),.UNSPECIFIED.);
#2211=B_SPLINE_CURVE_WITH_KNOTS('',3,(#24626,#24627,#24628,#24629,#24630,
#24631,#24632,#24633,#24634,#24635,#24636,#24637,#24638,#24639,#24640,#24641,
#24642,#24643,#24644,#24645,#24646,#24647,#24648,#24649,#24650,#24651,#24652,
#24653,#24654,#24655,#24656,#24657,#24658,#24659,#24660,#24661,#24662,#24663,
#24664,#24665,#24666,#24667,#24668,#24669,#24670,#24671,#24672,#24673),
 .UNSPECIFIED.,.F.,.F.,(4,2,2,2,2,2,2,2,2,2,2,2,2,2,2,2,2,2,2,2,2,2,2,4),
(-1.10411146984742,-1.03533191665006,-0.976118742178351,-0.919309605921176,
-0.852147695059822,-0.818850329922423,-0.78710553631429,-0.719605202451663,
-0.685897537282491,-0.653720218096601,-0.58591693177771,-0.533253067073543,
-0.48048894685478,-0.412938810261147,-0.380861562376602,-0.345537529156284,
-0.278404282958939,-0.244685076002604,-0.208482114930744,-0.147691075996069,
-0.119500524352719,-0.0875443739883855,-0.0452588878587829,-5.56419715291266E-5),
 .UNSPECIFIED.);
#2212=B_SPLINE_CURVE_WITH_KNOTS('',3,(#24815,#24816,#24817,#24818,#24819,
#24820,#24821,#24822,#24823,#24824,#24825,#24826,#24827,#24828,#24829,#24830,
#24831,#24832,#24833,#24834,#24835,#24836,#24837,#24838,#24839,#24840,#24841,
#24842,#24843,#24844,#24845,#24846,#24847,#24848,#24849,#24850,#24851,#24852,
#24853,#24854,#24855,#24856,#24857,#24858,#24859,#24860,#24861,#24862,#24863,
#24864,#24865,#24866,#24867,#24868,#24869,#24870,#24871,#24872,#24873,#24874,
#24875,#24876,#24877,#24878,#24879,#24880,#24881,#24882,#24883,#24884,#24885,
#24886,#24887,#24888,#24889,#24890,#24891,#24892,#24893,#24894,#24895,#24896,
#24897,#24898,#24899,#24900,#24901,#24902,#24903,#24904,#24905,#24906,#24907,
#24908,#24909,#24910,#24911,#24912,#24913,#24914,#24915,#24916,#24917,#24918,
#24919,#24920,#24921,#24922,#24923,#24924,#24925,#24926,#24927,#24928,#24929,
#24930,#24931,#24932,#24933,#24934,#24935,#24936,#24937,#24938,#24939,#24940,
#24941,#24942,#24943,#24944,#24945,#24946,#24947,#24948,#24949,#24950,#24951,
#24952,#24953,#24954,#24955,#24956,#24957,#24958,#24959,#24960,#24961,#24962,
#24963,#24964,#24965,#24966,#24967,#24968,#24969,#24970,#24971,#24972,#24973,
#24974,#24975,#24976,#24977,#24978,#24979,#24980,#24981,#24982,#24983,#24984,
#24985,#24986,#24987,#24988,#24989,#24990,#24991,#24992,#24993,#24994,#24995,
#24996),.UNSPECIFIED.,.F.,.F.,(4,2,2,2,2,2,2,2,2,2,2,2,2,2,2,2,2,2,2,2,
2,2,2,2,2,2,2,2,2,2,2,2,2,2,2,2,2,2,2,2,2,2,2,2,2,2,2,2,2,2,2,2,2,2,2,2,
2,2,2,2,2,2,2,2,2,2,2,2,2,2,2,2,2,2,2,2,2,2,2,2,2,2,2,2,2,2,2,2,2,2,4),
(-2.59260712215313,-2.56690100601658,-2.54670662204792,-2.51795361125489,
-2.49921831040747,-2.46249682575997,-2.44120808436947,-2.40565061488907,
-2.38623267798292,-2.34994659263002,-2.32792880857738,-2.2914594924406,
-2.27200532567065,-2.23521000439549,-2.21315975079308,-2.17649824646819,
-2.15687504523822,-2.1198074010745,-2.09755679524307,-2.06059452890559,
-2.04080414862994,-2.0034341153344,-1.98099653145175,-1.94372036045755,
-1.92376979199521,-1.88608952366635,-1.86346913878391,-1.825886307371,-1.80577140708762,
-1.7677879985442,-1.74497785805425,-1.70707208286967,-1.68679565593267,
-1.64852898921098,-1.62551957915289,-1.58724299799866,-1.5668194156521,
-1.52837962022198,-1.50512689617436,-1.46625959367599,-1.445761725099,-1.4076809055734,
-1.38397962847684,-1.34347567036628,-1.32325230788248,-1.28842096624431,
-1.25281821723327,-1.23161829626377,-1.19259825825371,-1.16847365331844,
-1.13073625058469,-1.10942156761083,-1.07178747146495,-1.04809462598784,
-1.01022758913448,-0.989056327476576,-0.952017607520454,-0.928604568917411,
-0.891011047611388,-0.870038435830354,-0.833420975844612,-0.810253474529773,
-0.773017026933345,-0.75225329511157,-0.716017195124668,-0.693086895893007,
-0.656221226579299,-0.635667718134776,-0.599797207642169,-0.577096643100117,
-0.540606746163167,-0.520258066612007,-0.48476128753358,-0.462295331776445,
-0.42616965811013,-0.406033927396684,-0.370888164878453,-0.34866243581743,
-0.312880071015608,-0.292952349354644,-0.25807087311542,-0.235935491552819,
-0.200705201394322,-0.18085933901615,-0.146951858374274,-0.125596239341413,
-0.0899673940341012,-0.0708845944680406,-0.0423960687726755,-0.0111460199290559,
-0.000107286410655352),.UNSPECIFIED.);
#2636=LINE('',#20155,#3101);
#2637=LINE('',#20157,#3102);
#2638=LINE('',#20159,#3103);
#2639=LINE('',#20161,#3104);
#2640=LINE('',#20163,#3105);
#2641=LINE('',#20164,#3106);
#2642=LINE('',#20167,#3107);
#2643=LINE('',#20173,#3108);
#2644=LINE('',#20283,#3109);
#2645=LINE('',#20286,#3110);
#2646=LINE('',#20288,#3111);
#2647=LINE('',#20289,#3112);
#2648=LINE('',#20292,#3113);
#2649=LINE('',#20293,#3114);
#2650=LINE('',#20296,#3115);
#2651=LINE('',#20297,#3116);
#2652=LINE('',#20300,#3117);
#2653=LINE('',#20301,#3118);
#2654=LINE('',#20304,#3119);
#2655=LINE('',#20305,#3120);
#2656=LINE('',#20307,#3121);
#2657=LINE('',#20318,#3122);
#2658=LINE('',#20413,#3123);
#2659=LINE('',#20756,#3124);
#2660=LINE('',#21075,#3125);
#2661=LINE('',#21470,#3126);
#2662=LINE('',#21613,#3127);
#2663=LINE('',#22000,#3128);
#2664=LINE('',#22387,#3129);
#2665=LINE('',#23027,#3130);
#2666=LINE('',#23029,#3131);
#2667=LINE('',#23201,#3132);
#2668=LINE('',#23640,#3133);
#2669=LINE('',#24017,#3134);
#2670=LINE('',#24158,#3135);
#2671=LINE('',#24300,#3136);
#2672=LINE('',#24674,#3137);
#3101=VECTOR('',#11174,2.42487113059592);
#3102=VECTOR('',#11175,2.424871130596);
#3103=VECTOR('',#11176,2.42487113059592);
#3104=VECTOR('',#11177,2.42487113059592);
#3105=VECTOR('',#11178,2.424871130596);
#3106=VECTOR('',#11179,2.42487113059592);
#3107=VECTOR('',#11182,3.);
#3108=VECTOR('',#11189,3.);
#3109=VECTOR('',#11202,0.9);
#3110=VECTOR('',#11205,4.4);
#3111=VECTOR('',#11206,2.42487113059592);
#3112=VECTOR('',#11207,4.4);
#3113=VECTOR('',#11210,2.424871130596);
#3114=VECTOR('',#11211,4.4);
#3115=VECTOR('',#11214,2.42487113059592);
#3116=VECTOR('',#11215,4.4);
#3117=VECTOR('',#11218,2.42487113059592);
#3118=VECTOR('',#11219,4.4);
#3119=VECTOR('',#11222,2.424871130596);
#3120=VECTOR('',#11223,4.4);
#3121=VECTOR('',#11226,2.42487113059592);
#3122=VECTOR('',#11231,0.1596734338228);
#3123=VECTOR('',#11234,0.09218749999999);
#3124=VECTOR('',#11235,0.384529946162085);
#3125=VECTOR('',#11236,0.384529946162085);
#3126=VECTOR('',#11237,0.1154700538379);
#3127=VECTOR('',#11238,0.1154700538379);
#3128=VECTOR('',#11239,0.1154700538379);
#3129=VECTOR('',#11240,0.1154700538379);
#3130=VECTOR('',#11243,0.1596734338228);
#3131=VECTOR('',#11244,0.4078125);
#3132=VECTOR('',#11249,0.384529946162085);
#3133=VECTOR('',#11252,0.384529946162085);
#3134=VECTOR('',#11253,0.384529946162088);
#3135=VECTOR('',#11254,0.384529946162088);
#3136=VECTOR('',#11255,0.384529946162088);
#3137=VECTOR('',#11256,0.384529946162088);
#3717=VERTEX_POINT('',#20151);
#3718=VERTEX_POINT('',#20153);
#3719=VERTEX_POINT('',#20154);
#3720=VERTEX_POINT('',#20156);
#3721=VERTEX_POINT('',#20158);
#3722=VERTEX_POINT('',#20160);
#3723=VERTEX_POINT('',#20162);
#3724=VERTEX_POINT('',#20166);
#3725=VERTEX_POINT('',#20170);
#3726=VERTEX_POINT('',#20172);
#3727=VERTEX_POINT('',#20177);
#3728=VERTEX_POINT('',#20224);
#3729=VERTEX_POINT('',#20225);
#3730=VERTEX_POINT('',#20280);
#3731=VERTEX_POINT('',#20285);
#3732=VERTEX_POINT('',#20287);
#3733=VERTEX_POINT('',#20291);
#3734=VERTEX_POINT('',#20295);
#3735=VERTEX_POINT('',#20299);
#3736=VERTEX_POINT('',#20303);
#3737=VERTEX_POINT('',#20309);
#3738=VERTEX_POINT('',#20310);
#3739=VERTEX_POINT('',#20315);
#3740=VERTEX_POINT('',#20317);
#3741=VERTEX_POINT('',#20319);
#3742=VERTEX_POINT('',#20330);
#3743=VERTEX_POINT('',#20400);
#3744=VERTEX_POINT('',#20554);
#3745=VERTEX_POINT('',#20755);
#3746=VERTEX_POINT('',#21021);
#3747=VERTEX_POINT('',#21074);
#3748=VERTEX_POINT('',#21611);
#3749=VERTEX_POINT('',#21612);
#3750=VERTEX_POINT('',#21998);
#3751=VERTEX_POINT('',#21999);
#3752=VERTEX_POINT('',#22385);
#3753=VERTEX_POINT('',#22386);
#3754=VERTEX_POINT('',#22772);
#3755=VERTEX_POINT('',#22773);
#3756=VERTEX_POINT('',#23025);
#3757=VERTEX_POINT('',#23026);
#3758=VERTEX_POINT('',#23028);
#3759=VERTEX_POINT('',#23043);
#3760=VERTEX_POINT('',#23054);
#3761=VERTEX_POINT('',#23200);
#3762=VERTEX_POINT('',#23587);
#3763=VERTEX_POINT('',#23781);
#3764=VERTEX_POINT('',#23966);
#3765=VERTEX_POINT('',#24299);
#3766=VERTEX_POINT('',#24625);
#4749=EDGE_CURVE('',#3717,#3717,#1861,.T.);
#4750=EDGE_CURVE('',#3718,#3719,#2636,.T.);
#4751=EDGE_CURVE('',#3720,#3718,#2637,.T.);
#4752=EDGE_CURVE('',#3721,#3720,#2638,.T.);
#4753=EDGE_CURVE('',#3722,#3721,#2639,.T.);
#4754=EDGE_CURVE('',#3723,#3722,#2640,.T.);
#4755=EDGE_CURVE('',#3719,#3723,#2641,.T.);
#4756=EDGE_CURVE('',#3717,#3724,#2642,.T.);
#4757=EDGE_CURVE('',#3724,#3724,#1862,.T.);
#4758=EDGE_CURVE('',#3725,#3725,#1863,.T.);
#4759=EDGE_CURVE('',#3725,#3726,#2643,.T.);
#4760=EDGE_CURVE('',#3726,#3726,#1864,.T.);
#4761=EDGE_CURVE('',#3724,#3725,#1865,.T.);
#4762=EDGE_CURVE('',#3727,#3727,#2179,.T.);
#4763=EDGE_CURVE('',#3728,#3729,#2180,.T.);
#4764=EDGE_CURVE('',#3729,#3728,#2181,.T.);
#4765=EDGE_CURVE('',#3726,#3730,#1866,.T.);
#4766=EDGE_CURVE('',#3729,#3727,#2644,.T.);
#4767=EDGE_CURVE('',#3719,#3731,#2645,.T.);
#4768=EDGE_CURVE('',#3732,#3731,#2646,.T.);
#4769=EDGE_CURVE('',#3718,#3732,#2647,.T.);
#4770=EDGE_CURVE('',#3733,#3732,#2648,.T.);
#4771=EDGE_CURVE('',#3720,#3733,#2649,.T.);
#4772=EDGE_CURVE('',#3734,#3733,#2650,.T.);
#4773=EDGE_CURVE('',#3721,#3734,#2651,.T.);
#4774=EDGE_CURVE('',#3735,#3734,#2652,.T.);
#4775=EDGE_CURVE('',#3722,#3735,#2653,.T.);
#4776=EDGE_CURVE('',#3736,#3735,#2654,.T.);
#4777=EDGE_CURVE('',#3723,#3736,#2655,.T.);
#4778=EDGE_CURVE('',#3731,#3736,#2656,.T.);
#4779=EDGE_CURVE('',#3737,#3738,#2182,.T.);
#4780=EDGE_CURVE('',#3739,#3737,#1867,.T.);
#4781=EDGE_CURVE('',#3739,#3740,#2657,.T.);
#4782=EDGE_CURVE('',#3741,#3740,#2183,.T.);
#4783=EDGE_CURVE('',#3742,#3741,#2184,.T.);
#4784=EDGE_CURVE('',#3738,#3742,#2185,.T.);
#4785=EDGE_CURVE('',#3743,#3737,#2186,.T.);
#4786=EDGE_CURVE('',#3743,#3739,#2658,.T.);
#4787=EDGE_CURVE('',#3744,#3742,#2187,.T.);
#4788=EDGE_CURVE('',#3744,#3745,#2659,.T.);
#4789=EDGE_CURVE('',#3745,#3743,#2188,.T.);
#4790=EDGE_CURVE('',#3743,#3740,#2189,.T.);
#4791=EDGE_CURVE('',#3745,#3746,#2190,.T.);
#4792=EDGE_CURVE('',#3746,#3747,#2660,.T.);
#4793=EDGE_CURVE('',#3747,#3741,#2191,.T.);
#4794=EDGE_CURVE('',#3747,#3744,#2661,.T.);
#4795=EDGE_CURVE('',#3748,#3749,#2662,.T.);
#4796=EDGE_CURVE('',#3749,#3744,#2192,.T.);
#4797=EDGE_CURVE('',#3748,#3747,#2193,.T.);
#4798=EDGE_CURVE('',#3750,#3751,#2663,.T.);
#4799=EDGE_CURVE('',#3751,#3749,#2194,.T.);
#4800=EDGE_CURVE('',#3750,#3748,#2195,.T.);
#4801=EDGE_CURVE('',#3752,#3753,#2664,.T.);
#4802=EDGE_CURVE('',#3753,#3751,#2196,.T.);
#4803=EDGE_CURVE('',#3752,#3750,#2197,.T.);
#4804=EDGE_CURVE('',#3754,#3755,#2198,.T.);
#4805=EDGE_CURVE('',#3755,#3753,#2199,.T.);
#4806=EDGE_CURVE('',#3754,#3752,#2200,.T.);
#4807=EDGE_CURVE('',#3756,#3757,#2665,.T.);
#4808=EDGE_CURVE('',#3756,#3758,#2666,.T.);
#4809=EDGE_CURVE('',#3755,#3758,#2201,.T.);
#4810=EDGE_CURVE('',#3757,#3754,#2202,.T.);
#4811=EDGE_CURVE('',#3759,#3757,#2203,.T.);
#4812=EDGE_CURVE('',#3759,#3760,#2204,.T.);
#4813=EDGE_CURVE('',#3760,#3756,#1868,.T.);
#4814=EDGE_CURVE('',#3761,#3752,#2667,.T.);
#4815=EDGE_CURVE('',#3758,#3761,#2205,.F.);
#4816=EDGE_CURVE('',#3758,#3760,#2206,.T.);
#4817=EDGE_CURVE('',#3761,#3762,#2207,.T.);
#4818=EDGE_CURVE('',#3753,#3762,#2668,.T.);
#4819=EDGE_CURVE('',#3762,#3763,#2208,.T.);
#4820=EDGE_CURVE('',#3763,#3764,#2209,.T.);
#4821=EDGE_CURVE('',#3751,#3764,#2669,.T.);
#4822=EDGE_CURVE('',#3763,#3750,#2670,.T.);
#4823=EDGE_CURVE('',#3765,#3748,#2671,.T.);
#4824=EDGE_CURVE('',#3764,#3765,#2210,.F.);
#4825=EDGE_CURVE('',#3765,#3766,#2211,.T.);
#4826=EDGE_CURVE('',#3749,#3766,#2672,.T.);
#4827=EDGE_CURVE('',#3766,#3746,#2212,.T.);
#6606=ORIENTED_EDGE('',*,*,#4749,.F.);
#6607=ORIENTED_EDGE('',*,*,#4750,.F.);
#6608=ORIENTED_EDGE('',*,*,#4751,.F.);
#6609=ORIENTED_EDGE('',*,*,#4752,.F.);
#6610=ORIENTED_EDGE('',*,*,#4753,.F.);
#6611=ORIENTED_EDGE('',*,*,#4754,.F.);
#6612=ORIENTED_EDGE('',*,*,#4755,.F.);
#6613=ORIENTED_EDGE('',*,*,#4749,.T.);
#6614=ORIENTED_EDGE('',*,*,#4756,.T.);
#6615=ORIENTED_EDGE('',*,*,#4757,.T.);
#6616=ORIENTED_EDGE('',*,*,#4756,.F.);
#6617=ORIENTED_EDGE('',*,*,#4758,.F.);
#6618=ORIENTED_EDGE('',*,*,#4759,.T.);
#6619=ORIENTED_EDGE('',*,*,#4760,.T.);
#6620=ORIENTED_EDGE('',*,*,#4759,.F.);
#6621=ORIENTED_EDGE('',*,*,#4757,.F.);
#6622=ORIENTED_EDGE('',*,*,#4761,.T.);
#6623=ORIENTED_EDGE('',*,*,#4758,.T.);
#6624=ORIENTED_EDGE('',*,*,#4761,.F.);
#6625=ORIENTED_EDGE('',*,*,#4762,.T.);
#6626=ORIENTED_EDGE('',*,*,#4763,.T.);
#6627=ORIENTED_EDGE('',*,*,#4764,.T.);
#6628=ORIENTED_EDGE('',*,*,#4760,.F.);
#6629=ORIENTED_EDGE('',*,*,#4765,.T.);
#6630=ORIENTED_EDGE('',*,*,#4765,.F.);
#6631=ORIENTED_EDGE('',*,*,#4763,.F.);
#6632=ORIENTED_EDGE('',*,*,#4764,.F.);
#6633=ORIENTED_EDGE('',*,*,#4766,.T.);
#6634=ORIENTED_EDGE('',*,*,#4762,.F.);
#6635=ORIENTED_EDGE('',*,*,#4766,.F.);
#6636=ORIENTED_EDGE('',*,*,#4750,.T.);
#6637=ORIENTED_EDGE('',*,*,#4767,.T.);
#6638=ORIENTED_EDGE('',*,*,#4768,.F.);
#6639=ORIENTED_EDGE('',*,*,#4769,.F.);
#6640=ORIENTED_EDGE('',*,*,#4751,.T.);
#6641=ORIENTED_EDGE('',*,*,#4769,.T.);
#6642=ORIENTED_EDGE('',*,*,#4770,.F.);
#6643=ORIENTED_EDGE('',*,*,#4771,.F.);
#6644=ORIENTED_EDGE('',*,*,#4752,.T.);
#6645=ORIENTED_EDGE('',*,*,#4771,.T.);
#6646=ORIENTED_EDGE('',*,*,#4772,.F.);
#6647=ORIENTED_EDGE('',*,*,#4773,.F.);
#6648=ORIENTED_EDGE('',*,*,#4753,.T.);
#6649=ORIENTED_EDGE('',*,*,#4773,.T.);
#6650=ORIENTED_EDGE('',*,*,#4774,.F.);
#6651=ORIENTED_EDGE('',*,*,#4775,.F.);
#6652=ORIENTED_EDGE('',*,*,#4754,.T.);
#6653=ORIENTED_EDGE('',*,*,#4775,.T.);
#6654=ORIENTED_EDGE('',*,*,#4776,.F.);
#6655=ORIENTED_EDGE('',*,*,#4777,.F.);
#6656=ORIENTED_EDGE('',*,*,#4755,.T.);
#6657=ORIENTED_EDGE('',*,*,#4777,.T.);
#6658=ORIENTED_EDGE('',*,*,#4778,.F.);
#6659=ORIENTED_EDGE('',*,*,#4767,.F.);
#6660=ORIENTED_EDGE('',*,*,#4768,.T.);
#6661=ORIENTED_EDGE('',*,*,#4778,.T.);
#6662=ORIENTED_EDGE('',*,*,#4776,.T.);
#6663=ORIENTED_EDGE('',*,*,#4774,.T.);
#6664=ORIENTED_EDGE('',*,*,#4772,.T.);
#6665=ORIENTED_EDGE('',*,*,#4770,.T.);
#6666=ORIENTED_EDGE('',*,*,#4779,.F.);
#6667=ORIENTED_EDGE('',*,*,#4780,.F.);
#6668=ORIENTED_EDGE('',*,*,#4781,.T.);
#6669=ORIENTED_EDGE('',*,*,#4782,.F.);
#6670=ORIENTED_EDGE('',*,*,#4783,.F.);
#6671=ORIENTED_EDGE('',*,*,#4784,.F.);
#6672=ORIENTED_EDGE('',*,*,#4780,.T.);
#6673=ORIENTED_EDGE('',*,*,#4785,.F.);
#6674=ORIENTED_EDGE('',*,*,#4786,.T.);
#6675=ORIENTED_EDGE('',*,*,#4784,.T.);
#6676=ORIENTED_EDGE('',*,*,#4787,.F.);
#6677=ORIENTED_EDGE('',*,*,#4788,.T.);
#6678=ORIENTED_EDGE('',*,*,#4789,.T.);
#6679=ORIENTED_EDGE('',*,*,#4785,.T.);
#6680=ORIENTED_EDGE('',*,*,#4779,.T.);
#6681=ORIENTED_EDGE('',*,*,#4782,.T.);
#6682=ORIENTED_EDGE('',*,*,#4790,.F.);
#6683=ORIENTED_EDGE('',*,*,#4789,.F.);
#6684=ORIENTED_EDGE('',*,*,#4791,.T.);
#6685=ORIENTED_EDGE('',*,*,#4792,.T.);
#6686=ORIENTED_EDGE('',*,*,#4793,.T.);
#6687=ORIENTED_EDGE('',*,*,#4783,.T.);
#6688=ORIENTED_EDGE('',*,*,#4793,.F.);
#6689=ORIENTED_EDGE('',*,*,#4794,.T.);
#6690=ORIENTED_EDGE('',*,*,#4787,.T.);
#6691=ORIENTED_EDGE('',*,*,#4795,.T.);
#6692=ORIENTED_EDGE('',*,*,#4796,.T.);
#6693=ORIENTED_EDGE('',*,*,#4794,.F.);
#6694=ORIENTED_EDGE('',*,*,#4797,.F.);
#6695=ORIENTED_EDGE('',*,*,#4798,.T.);
#6696=ORIENTED_EDGE('',*,*,#4799,.T.);
#6697=ORIENTED_EDGE('',*,*,#4795,.F.);
#6698=ORIENTED_EDGE('',*,*,#4800,.F.);
#6699=ORIENTED_EDGE('',*,*,#4801,.T.);
#6700=ORIENTED_EDGE('',*,*,#4802,.T.);
#6701=ORIENTED_EDGE('',*,*,#4798,.F.);
#6702=ORIENTED_EDGE('',*,*,#4803,.F.);
#6703=ORIENTED_EDGE('',*,*,#4804,.T.);
#6704=ORIENTED_EDGE('',*,*,#4805,.T.);
#6705=ORIENTED_EDGE('',*,*,#4801,.F.);
#6706=ORIENTED_EDGE('',*,*,#4806,.F.);
#6707=ORIENTED_EDGE('',*,*,#4807,.F.);
#6708=ORIENTED_EDGE('',*,*,#4808,.T.);
#6709=ORIENTED_EDGE('',*,*,#4809,.F.);
#6710=ORIENTED_EDGE('',*,*,#4804,.F.);
#6711=ORIENTED_EDGE('',*,*,#4810,.F.);
#6712=ORIENTED_EDGE('',*,*,#4811,.F.);
#6713=ORIENTED_EDGE('',*,*,#4812,.T.);
#6714=ORIENTED_EDGE('',*,*,#4813,.T.);
#6715=ORIENTED_EDGE('',*,*,#4807,.T.);
#6716=ORIENTED_EDGE('',*,*,#4811,.T.);
#6717=ORIENTED_EDGE('',*,*,#4810,.T.);
#6718=ORIENTED_EDGE('',*,*,#4806,.T.);
#6719=ORIENTED_EDGE('',*,*,#4814,.F.);
#6720=ORIENTED_EDGE('',*,*,#4815,.F.);
#6721=ORIENTED_EDGE('',*,*,#4816,.T.);
#6722=ORIENTED_EDGE('',*,*,#4812,.F.);
#6723=ORIENTED_EDGE('',*,*,#4813,.F.);
#6724=ORIENTED_EDGE('',*,*,#4816,.F.);
#6725=ORIENTED_EDGE('',*,*,#4808,.F.);
#6726=ORIENTED_EDGE('',*,*,#4815,.T.);
#6727=ORIENTED_EDGE('',*,*,#4817,.T.);
#6728=ORIENTED_EDGE('',*,*,#4818,.F.);
#6729=ORIENTED_EDGE('',*,*,#4805,.F.);
#6730=ORIENTED_EDGE('',*,*,#4809,.T.);
#6731=ORIENTED_EDGE('',*,*,#4819,.T.);
#6732=ORIENTED_EDGE('',*,*,#4820,.T.);
#6733=ORIENTED_EDGE('',*,*,#4821,.F.);
#6734=ORIENTED_EDGE('',*,*,#4802,.F.);
#6735=ORIENTED_EDGE('',*,*,#4818,.T.);
#6736=ORIENTED_EDGE('',*,*,#4817,.F.);
#6737=ORIENTED_EDGE('',*,*,#4814,.T.);
#6738=ORIENTED_EDGE('',*,*,#4803,.T.);
#6739=ORIENTED_EDGE('',*,*,#4822,.F.);
#6740=ORIENTED_EDGE('',*,*,#4819,.F.);
#6741=ORIENTED_EDGE('',*,*,#4820,.F.);
#6742=ORIENTED_EDGE('',*,*,#4822,.T.);
#6743=ORIENTED_EDGE('',*,*,#4800,.T.);
#6744=ORIENTED_EDGE('',*,*,#4823,.F.);
#6745=ORIENTED_EDGE('',*,*,#4824,.F.);
#6746=ORIENTED_EDGE('',*,*,#4824,.T.);
#6747=ORIENTED_EDGE('',*,*,#4825,.T.);
#6748=ORIENTED_EDGE('',*,*,#4826,.F.);
#6749=ORIENTED_EDGE('',*,*,#4799,.F.);
#6750=ORIENTED_EDGE('',*,*,#4821,.T.);
#6751=ORIENTED_EDGE('',*,*,#4827,.T.);
#6752=ORIENTED_EDGE('',*,*,#4791,.F.);
#6753=ORIENTED_EDGE('',*,*,#4788,.F.);
#6754=ORIENTED_EDGE('',*,*,#4796,.F.);
#6755=ORIENTED_EDGE('',*,*,#4826,.T.);
#6756=ORIENTED_EDGE('',*,*,#4825,.F.);
#6757=ORIENTED_EDGE('',*,*,#4823,.T.);
#6758=ORIENTED_EDGE('',*,*,#4797,.T.);
#6759=ORIENTED_EDGE('',*,*,#4792,.F.);
#6760=ORIENTED_EDGE('',*,*,#4827,.F.);
#6761=ORIENTED_EDGE('',*,*,#4781,.F.);
#6762=ORIENTED_EDGE('',*,*,#4786,.F.);
#6763=ORIENTED_EDGE('',*,*,#4790,.T.);
#8486=CYLINDRICAL_SURFACE('',#9670,3.);
#8487=CYLINDRICAL_SURFACE('',#9672,3.);
#8488=CYLINDRICAL_SURFACE('',#9679,0.9);
#8489=CYLINDRICAL_SURFACE('',#9688,1.5);
#8490=CYLINDRICAL_SURFACE('',#9692,1.5);
#8756=ADVANCED_FACE('',(#693,#293),#425,.T.);
#8757=ADVANCED_FACE('',(#694),#8486,.T.);
#8758=ADVANCED_FACE('',(#695),#8487,.T.);
#8759=ADVANCED_FACE('',(#696,#294,#295),#207,.F.);
#8760=ADVANCED_FACE('',(#697),#285,.T.);
#8761=ADVANCED_FACE('',(#698),#8488,.F.);
#8762=ADVANCED_FACE('',(#699),#426,.T.);
#8763=ADVANCED_FACE('',(#700),#427,.T.);
#8764=ADVANCED_FACE('',(#701),#428,.T.);
#8765=ADVANCED_FACE('',(#702),#429,.T.);
#8766=ADVANCED_FACE('',(#703),#430,.T.);
#8767=ADVANCED_FACE('',(#704),#431,.T.);
#8768=ADVANCED_FACE('',(#705,#296),#432,.T.);
#8769=ADVANCED_FACE('',(#706),#8489,.F.);
#8770=ADVANCED_FACE('',(#707),#343,.T.);
#8771=ADVANCED_FACE('',(#708),#344,.T.);
#8772=ADVANCED_FACE('',(#709),#345,.T.);
#8773=ADVANCED_FACE('',(#710),#346,.T.);
#8774=ADVANCED_FACE('',(#711),#347,.T.);
#8775=ADVANCED_FACE('',(#712),#348,.T.);
#8776=ADVANCED_FACE('',(#713),#349,.T.);
#8777=ADVANCED_FACE('',(#714),#433,.F.);
#8778=ADVANCED_FACE('',(#715),#434,.T.);
#8779=ADVANCED_FACE('',(#716),#350,.T.);
#8780=ADVANCED_FACE('',(#717),#8490,.F.);
#8781=ADVANCED_FACE('',(#718),#351,.T.);
#8782=ADVANCED_FACE('',(#719),#352,.T.);
#8783=ADVANCED_FACE('',(#720),#353,.T.);
#8784=ADVANCED_FACE('',(#721),#354,.T.);
#8785=ADVANCED_FACE('',(#722),#355,.T.);
#8786=ADVANCED_FACE('',(#723),#356,.T.);
#8787=ADVANCED_FACE('',(#724),#357,.T.);
#8788=ADVANCED_FACE('',(#725),#435,.T.);
#9120=CLOSED_SHELL('',(#8756,#8757,#8758,#8759,#8760,#8761,#8762,#8763,
#8764,#8765,#8766,#8767,#8768,#8769,#8770,#8771,#8772,#8773,#8774,#8775,
#8776,#8777,#8778,#8779,#8780,#8781,#8782,#8783,#8784,#8785,#8786,#8787,
#8788));
#9667=AXIS2_PLACEMENT_3D('',#20149,#11168,#11169);
#9668=AXIS2_PLACEMENT_3D('',#20150,#11170,#11171);
#9669=AXIS2_PLACEMENT_3D('',#20152,#11172,#11173);
#9670=AXIS2_PLACEMENT_3D('',#20165,#11180,#11181);
#9671=AXIS2_PLACEMENT_3D('',#20168,#11183,#11184);
#9672=AXIS2_PLACEMENT_3D('',#20169,#11185,#11186);
#9673=AXIS2_PLACEMENT_3D('',#20171,#11187,#11188);
#9674=AXIS2_PLACEMENT_3D('',#20174,#11190,#11191);
#9675=AXIS2_PLACEMENT_3D('',#20175,#11192,#11193);
#9676=AXIS2_PLACEMENT_3D('',#20176,#11194,#11195);
#9677=AXIS2_PLACEMENT_3D('',#20279,#11196,#11197);
#9678=AXIS2_PLACEMENT_3D('',#20281,#11198,#11199);
#9679=AXIS2_PLACEMENT_3D('',#20282,#11200,#11201);
#9680=AXIS2_PLACEMENT_3D('',#20284,#11203,#11204);
#9681=AXIS2_PLACEMENT_3D('',#20290,#11208,#11209);
#9682=AXIS2_PLACEMENT_3D('',#20294,#11212,#11213);
#9683=AXIS2_PLACEMENT_3D('',#20298,#11216,#11217);
#9684=AXIS2_PLACEMENT_3D('',#20302,#11220,#11221);
#9685=AXIS2_PLACEMENT_3D('',#20306,#11224,#11225);
#9686=AXIS2_PLACEMENT_3D('',#20308,#11227,#11228);
#9687=AXIS2_PLACEMENT_3D('',#20316,#11229,#11230);
#9688=AXIS2_PLACEMENT_3D('',#20399,#11232,#11233);
#9689=AXIS2_PLACEMENT_3D('',#23024,#11241,#11242);
#9690=AXIS2_PLACEMENT_3D('',#23042,#11245,#11246);
#9691=AXIS2_PLACEMENT_3D('',#23059,#11247,#11248);
#9692=AXIS2_PLACEMENT_3D('',#23446,#11250,#11251);
#9693=AXIS2_PLACEMENT_3D('',#25137,#11257,#11258);
#11168=DIRECTION('axis',(0.,0.,1.));
#11169=DIRECTION('refdir',(1.,0.,0.));
#11170=DIRECTION('center_axis',(0.,0.,-1.));
#11171=DIRECTION('ref_axis',(0.,-1.,0.));
#11172=DIRECTION('center_axis',(0.,0.,1.));
#11173=DIRECTION('ref_axis',(0.,1.,0.));
#11174=DIRECTION('',(0.866025403784429,0.500000000000017,0.));
#11175=DIRECTION('',(0.,1.,0.));
#11176=DIRECTION('',(-0.866025403784429,0.500000000000017,0.));
#11177=DIRECTION('',(-0.866025403784429,-0.500000000000017,0.));
#11178=DIRECTION('',(0.,-1.,0.));
#11179=DIRECTION('',(0.866025403784429,-0.500000000000017,0.));
#11180=DIRECTION('center_axis',(0.,0.,-1.));
#11181=DIRECTION('ref_axis',(0.,-1.,0.));
#11182=DIRECTION('',(0.,0.,1.));
#11183=DIRECTION('center_axis',(0.,0.,-1.));
#11184=DIRECTION('ref_axis',(0.,-1.,0.));
#11185=DIRECTION('center_axis',(0.,0.,-1.));
#11186=DIRECTION('ref_axis',(0.,-1.,0.));
#11187=DIRECTION('center_axis',(0.,0.,-1.));
#11188=DIRECTION('ref_axis',(0.,-1.,0.));
#11189=DIRECTION('',(0.,0.,1.));
#11190=DIRECTION('center_axis',(0.,0.,-1.));
#11191=DIRECTION('ref_axis',(0.,-1.,0.));
#11192=DIRECTION('center_axis',(0.,0.,-1.));
#11193=DIRECTION('ref_axis',(0.,-1.,0.));
#11194=DIRECTION('center_axis',(-1.,1.22464679914735E-16,0.));
#11195=DIRECTION('ref_axis',(1.22464679914735E-16,1.,0.));
#11196=DIRECTION('center_axis',(0.,-6.12323399573677E-17,-1.));
#11197=DIRECTION('ref_axis',(0.,-1.,0.));
#11198=DIRECTION('center_axis',(1.,-1.22464679914735E-16,0.));
#11199=DIRECTION('ref_axis',(1.22464679914735E-16,1.,0.));
#11200=DIRECTION('center_axis',(1.,0.,0.));
#11201=DIRECTION('ref_axis',(0.,-1.,0.));
#11202=DIRECTION('',(1.,0.,0.));
#11203=DIRECTION('center_axis',(-0.500000000000017,0.866025403784429,0.));
#11204=DIRECTION('ref_axis',(0.866025403784429,0.500000000000017,0.));
#11205=DIRECTION('',(0.,0.,-1.));
#11206=DIRECTION('',(0.866025403784429,0.500000000000017,0.));
#11207=DIRECTION('',(0.,0.,-1.));
#11208=DIRECTION('center_axis',(-1.,0.,0.));
#11209=DIRECTION('ref_axis',(0.,1.,0.));
#11210=DIRECTION('',(0.,1.,0.));
#11211=DIRECTION('',(0.,0.,-1.));
#11212=DIRECTION('center_axis',(-0.500000000000017,-0.866025403784429,0.));
#11213=DIRECTION('ref_axis',(-0.866025403784429,0.500000000000017,0.));
#11214=DIRECTION('',(-0.866025403784429,0.500000000000017,0.));
#11215=DIRECTION('',(0.,0.,-1.));
#11216=DIRECTION('center_axis',(0.500000000000017,-0.866025403784429,0.));
#11217=DIRECTION('ref_axis',(-0.866025403784429,-0.500000000000017,0.));
#11218=DIRECTION('',(-0.866025403784429,-0.500000000000017,0.));
#11219=DIRECTION('',(0.,0.,-1.));
#11220=DIRECTION('center_axis',(1.,0.,0.));
#11221=DIRECTION('ref_axis',(0.,-1.,0.));
#11222=DIRECTION('',(0.,-1.,0.));
#11223=DIRECTION('',(0.,0.,-1.));
#11224=DIRECTION('center_axis',(0.500000000000017,0.866025403784429,0.));
#11225=DIRECTION('ref_axis',(0.866025403784429,-0.500000000000017,0.));
#11226=DIRECTION('',(0.866025403784429,-0.500000000000017,0.));
#11227=DIRECTION('center_axis',(0.,0.,-1.));
#11228=DIRECTION('ref_axis',(0.,-1.,0.));
#11229=DIRECTION('center_axis',(0.,0.,-1.));
#11230=DIRECTION('ref_axis',(0.,-1.,0.));
#11231=DIRECTION('',(0.,1.,0.));
#11232=DIRECTION('center_axis',(0.,0.,-1.));
#11233=DIRECTION('ref_axis',(0.,-1.,0.));
#11234=DIRECTION('',(0.,0.,-1.));
#11235=DIRECTION('',(-0.50903696045512,0.700629269222028,-0.50000000000002));
#11236=DIRECTION('',(0.50903696045512,-0.700629269222028,-0.50000000000002));
#11237=DIRECTION('',(0.,0.,-1.));
#11238=DIRECTION('',(0.,0.,-1.));
#11239=DIRECTION('',(0.,0.,-1.));
#11240=DIRECTION('',(0.,0.,-1.));
#11241=DIRECTION('center_axis',(-1.,0.,0.));
#11242=DIRECTION('ref_axis',(0.,1.,0.));
#11243=DIRECTION('',(0.,1.,0.));
#11244=DIRECTION('',(0.,0.,-1.));
#11245=DIRECTION('center_axis',(0.,0.,-1.));
#11246=DIRECTION('ref_axis',(0.,-1.,0.));
#11247=DIRECTION('center_axis',(0.,0.,-1.));
#11248=DIRECTION('ref_axis',(-0.916187957117145,-0.40074883310312,0.));
#11249=DIRECTION('',(-0.50903696045512,-0.700629269222028,-0.50000000000002));
#11250=DIRECTION('center_axis',(0.,0.,-1.));
#11251=DIRECTION('ref_axis',(0.548802039292154,0.835952344137375,0.));
#11252=DIRECTION('',(0.50903696045512,0.700629269222028,-0.50000000000002));
#11253=DIRECTION('',(-0.823639103546326,-0.267616567329808,-0.500000000000015));
#11254=DIRECTION('',(0.823639103546326,0.267616567329808,-0.500000000000015));
#11255=DIRECTION('',(-0.823639103546326,0.267616567329808,-0.500000000000015));
#11256=DIRECTION('',(0.823639103546326,-0.267616567329808,-0.500000000000015));
#11257=DIRECTION('center_axis',(-1.,0.,0.));
#11258=DIRECTION('ref_axis',(0.,1.,0.));
#20149=CARTESIAN_POINT('',(0.,0.,0.));
#20150=CARTESIAN_POINT('Origin',(0.,0.,-27.8));
#20151=CARTESIAN_POINT('',(3.67394039744206E-16,3.,-27.8));
#20152=CARTESIAN_POINT('Origin',(0.,0.,-27.8));
#20153=CARTESIAN_POINT('',(-2.1,1.212435565298,-27.8));
#20154=CARTESIAN_POINT('',(0.,2.424871130596,-27.8));
#20155=CARTESIAN_POINT('',(-2.1,1.212435565298,-27.8));
#20156=CARTESIAN_POINT('',(-2.1,-1.212435565298,-27.8));
#20157=CARTESIAN_POINT('',(-2.1,-1.212435565298,-27.8));
#20158=CARTESIAN_POINT('',(0.,-2.424871130596,-27.8));
#20159=CARTESIAN_POINT('',(0.,-2.424871130596,-27.8));
#20160=CARTESIAN_POINT('',(2.1,-1.212435565298,-27.8));
#20161=CARTESIAN_POINT('',(2.1,-1.212435565298,-27.8));
#20162=CARTESIAN_POINT('',(2.1,1.212435565298,-27.8));
#20163=CARTESIAN_POINT('',(2.1,1.212435565298,-27.8));
#20164=CARTESIAN_POINT('',(0.,2.424871130596,-27.8));
#20165=CARTESIAN_POINT('Origin',(0.,0.,0.79));
#20166=CARTESIAN_POINT('',(3.67394039744206E-16,3.,-7.8));
#20167=CARTESIAN_POINT('',(3.67394039744206E-16,3.,0.79));
#20168=CARTESIAN_POINT('Origin',(0.,0.,-7.8));
#20169=CARTESIAN_POINT('Origin',(0.,0.,0.79));
#20170=CARTESIAN_POINT('',(0.,3.,-2.));
#20171=CARTESIAN_POINT('Origin',(0.,0.,-2.));
#20172=CARTESIAN_POINT('',(0.,3.,-1.));
#20173=CARTESIAN_POINT('',(3.67394039744206E-16,3.,0.79));
#20174=CARTESIAN_POINT('Origin',(0.,0.,-1.));
#20175=CARTESIAN_POINT('Origin',(0.,0.,-4.9));
#20176=CARTESIAN_POINT('Origin',(8.211256788283E-16,6.705,-4.9));
#20177=CARTESIAN_POINT('',(1.786057109949,0.9,-4.9));
#20178=CARTESIAN_POINT('Ctrl Pts',(2.08688079408944,-6.93889390390723E-17,
-5.8));
#20179=CARTESIAN_POINT('Ctrl Pts',(2.08688079408944,-0.101093267950358,
-5.8));
#20180=CARTESIAN_POINT('Ctrl Pts',(2.07606256936626,-0.200116780800449,
-5.78306010664896));
#20181=CARTESIAN_POINT('Ctrl Pts',(2.03456000012612,-0.400564730585056,
-5.7138100508258));
#20182=CARTESIAN_POINT('Ctrl Pts',(2.00198415673787,-0.497484683785943,
-5.65792591947954));
#20183=CARTESIAN_POINT('Ctrl Pts',(1.92762106375197,-0.672219726341367,
-5.51024657908061));
#20184=CARTESIAN_POINT('Ctrl Pts',(1.88521703073068,-0.747655625946073,
-5.41535484251112));
#20185=CARTESIAN_POINT('Ctrl Pts',(1.82963665913354,-0.837307075018212,
-5.23892457904444));
#20186=CARTESIAN_POINT('Ctrl Pts',(1.81154384378188,-0.863748989480202,
-5.16502186650821));
#20187=CARTESIAN_POINT('Ctrl Pts',(1.79307858729398,-0.890223641153724,
-5.04065959660885));
#20188=CARTESIAN_POINT('Ctrl Pts',(1.78858372602067,-0.896476659347317,
-4.99305285657899));
#20189=CARTESIAN_POINT('Ctrl Pts',(1.78533316749339,-0.901010715882009,
-4.90218285810826));
#20190=CARTESIAN_POINT('Ctrl Pts',(1.78599302794454,-0.900100579704181,
-4.85952137824838));
#20191=CARTESIAN_POINT('Ctrl Pts',(1.79231868802101,-0.891241854858108,
-4.76381818537325));
#20192=CARTESIAN_POINT('Ctrl Pts',(1.79916641606907,-0.881638078648367,
-4.71160904837683));
#20193=CARTESIAN_POINT('Ctrl Pts',(1.82686643689218,-0.84116912475279,-4.56481378587192));
#20194=CARTESIAN_POINT('Ctrl Pts',(1.85446030150783,-0.799437867210863,
-4.47550957740264));
#20195=CARTESIAN_POINT('Ctrl Pts',(1.91932437559004,-0.684995961096764,
-4.30636138511348));
#20196=CARTESIAN_POINT('Ctrl Pts',(1.95740679794227,-0.608819659462653,
-4.22838203723553));
#20197=CARTESIAN_POINT('Ctrl Pts',(2.02485323182035,-0.430006700487911,
-4.1016362333799));
#20198=CARTESIAN_POINT('Ctrl Pts',(2.05383693479979,-0.327023915525718,
-4.05368786483531));
#20199=CARTESIAN_POINT('Ctrl Pts',(2.08565111645498,-0.116269187541378,
-4.00170605857396));
#20200=CARTESIAN_POINT('Ctrl Pts',(2.09048597736785,-0.0135717077347775,
-3.99421211556224));
#20201=CARTESIAN_POINT('Ctrl Pts',(2.07776710291235,0.191484033440727,-4.01460189690483));
#20202=CARTESIAN_POINT('Ctrl Pts',(2.06053976427926,0.289671925625122,-4.04202503782963));
#20203=CARTESIAN_POINT('Ctrl Pts',(2.00671918893296,0.488728582767382,-4.13487097478375));
#20204=CARTESIAN_POINT('Ctrl Pts',(1.96758297172864,0.5844436089876,-4.20573850098139));
#20205=CARTESIAN_POINT('Ctrl Pts',(1.88908829229802,0.743279797016495,-4.37887910454814));
#20206=CARTESIAN_POINT('Ctrl Pts',(1.84955679967837,0.806500365822469,-4.48238860864025));
#20207=CARTESIAN_POINT('Ctrl Pts',(1.80880106698392,0.867867222875822,-4.65409622882472));
#20208=CARTESIAN_POINT('Ctrl Pts',(1.79841793711201,0.882619607672314,-4.7134689255317));
#20209=CARTESIAN_POINT('Ctrl Pts',(1.7880296495206,0.897274433692566,-4.81762265188009));
#20210=CARTESIAN_POINT('Ctrl Pts',(1.78590159063484,0.900216573916412,-4.86106047100695));
#20211=CARTESIAN_POINT('Ctrl Pts',(1.78623446722923,0.899753015094058,-4.94945829210191));
#20212=CARTESIAN_POINT('Ctrl Pts',(1.78880867985365,0.896191473409593,-4.99391013963609));
#20213=CARTESIAN_POINT('Ctrl Pts',(1.80063381565783,0.879464182449665,-5.10182083332412));
#20214=CARTESIAN_POINT('Ctrl Pts',(1.81229274734386,0.862820879832989,-5.16372701080558));
#20215=CARTESIAN_POINT('Ctrl Pts',(1.85616772350585,0.796015468290225,-5.33756367316692));
#20216=CARTESIAN_POINT('Ctrl Pts',(1.89697738935018,0.729525882843482,-5.44051832736629));
#20217=CARTESIAN_POINT('Ctrl Pts',(1.97477477835702,0.567312731060949,-5.60778248302471));
#20218=CARTESIAN_POINT('Ctrl Pts',(2.01201382633158,0.472866430429607,-5.67453279408918));
#20219=CARTESIAN_POINT('Ctrl Pts',(2.05457838510613,0.309311014743862,-5.74751544509335));
#20220=CARTESIAN_POINT('Ctrl Pts',(2.06663910190596,0.248843270470049,-5.76728897745186));
#20221=CARTESIAN_POINT('Ctrl Pts',(2.08273777581834,0.1251203935021,-5.79343657211952));
#20222=CARTESIAN_POINT('Ctrl Pts',(2.08688079408944,0.0628253026847131,
-5.8));
#20223=CARTESIAN_POINT('Ctrl Pts',(2.08688079408944,-1.27784594234186E-16,
-5.8));
#20224=CARTESIAN_POINT('',(-1.786057109949,-0.9,-4.9));
#20225=CARTESIAN_POINT('',(-1.78605710994918,0.9,-4.9));
#20226=CARTESIAN_POINT('Ctrl Pts',(-1.78605710994918,-0.9,-4.9));
#20227=CARTESIAN_POINT('Ctrl Pts',(-1.78605710994918,-0.9,-4.90157288708411));
#20228=CARTESIAN_POINT('Ctrl Pts',(-1.78606007091103,-0.899995876722818,
-4.90314607070815));
#20229=CARTESIAN_POINT('Ctrl Pts',(-1.78623446722923,-0.899753015094059,
-4.9494582921019));
#20230=CARTESIAN_POINT('Ctrl Pts',(-1.78880867985365,-0.896191473409595,
-4.99391013963609));
#20231=CARTESIAN_POINT('Ctrl Pts',(-1.80063381565783,-0.879464182449664,
-5.10182083332413));
#20232=CARTESIAN_POINT('Ctrl Pts',(-1.81229274734387,-0.862820879832981,
-5.1637270108056));
#20233=CARTESIAN_POINT('Ctrl Pts',(-1.85616772350585,-0.796015468290225,
-5.33756367316691));
#20234=CARTESIAN_POINT('Ctrl Pts',(-1.89697738935017,-0.729525882843488,
-5.44051832736628));
#20235=CARTESIAN_POINT('Ctrl Pts',(-1.97477477835702,-0.56731273106095,
-5.60778248302471));
#20236=CARTESIAN_POINT('Ctrl Pts',(-2.01201382633158,-0.472866430429608,
-5.67453279408918));
#20237=CARTESIAN_POINT('Ctrl Pts',(-2.05457838510613,-0.309311014743861,
-5.74751544509335));
#20238=CARTESIAN_POINT('Ctrl Pts',(-2.06663910190596,-0.248843270470049,
-5.76728897745186));
#20239=CARTESIAN_POINT('Ctrl Pts',(-2.08273777581834,-0.125120393502098,
-5.79343657211952));
#20240=CARTESIAN_POINT('Ctrl Pts',(-2.08688079408944,-0.0628253026847123,
-5.8));
#20241=CARTESIAN_POINT('Ctrl Pts',(-2.08688079408944,-1.27784594234186E-16,
-5.8));
#20242=CARTESIAN_POINT('Ctrl Pts',(-2.08688079408944,0.101093267950359,
-5.8));
#20243=CARTESIAN_POINT('Ctrl Pts',(-2.07606256936626,0.200116780800451,
-5.78306010664896));
#20244=CARTESIAN_POINT('Ctrl Pts',(-2.03456000012612,0.400564730585057,
-5.7138100508258));
#20245=CARTESIAN_POINT('Ctrl Pts',(-2.00198415673787,0.497484683785944,
-5.65792591947954));
#20246=CARTESIAN_POINT('Ctrl Pts',(-1.92762106375197,0.672219726341378,
-5.5102465790806));
#20247=CARTESIAN_POINT('Ctrl Pts',(-1.88521703073068,0.747655625946073,
-5.41535484251111));
#20248=CARTESIAN_POINT('Ctrl Pts',(-1.82963665913355,0.837307075018195,
-5.23892457904446));
#20249=CARTESIAN_POINT('Ctrl Pts',(-1.81154384378188,0.8637489894802,-5.16502186650822));
#20250=CARTESIAN_POINT('Ctrl Pts',(-1.79307858729398,0.890223641153724,
-5.04065959660886));
#20251=CARTESIAN_POINT('Ctrl Pts',(-1.78858372602066,0.896476659347318,
-4.99305285657899));
#20252=CARTESIAN_POINT('Ctrl Pts',(-1.78632454767185,0.899627884673538,
-4.92989708461551));
#20253=CARTESIAN_POINT('Ctrl Pts',(-1.78605710994918,0.9,-4.91494427305051));
#20254=CARTESIAN_POINT('Ctrl Pts',(-1.78605710994918,0.9,-4.9));
#20255=CARTESIAN_POINT('Ctrl Pts',(-1.78605710994918,0.9,-4.9));
#20256=CARTESIAN_POINT('Ctrl Pts',(-1.78605710994918,0.9,-4.87230304065669));
#20257=CARTESIAN_POINT('Ctrl Pts',(-1.7869769405052,0.89872266648372,-4.84463541023445));
#20258=CARTESIAN_POINT('Ctrl Pts',(-1.79231868802101,0.891241854858107,
-4.76381818537326));
#20259=CARTESIAN_POINT('Ctrl Pts',(-1.79916641606906,0.88163807864837,-4.71160904837684));
#20260=CARTESIAN_POINT('Ctrl Pts',(-1.82686643689218,0.841169124752791,
-4.56481378587192));
#20261=CARTESIAN_POINT('Ctrl Pts',(-1.85446030150783,0.799437867210866,
-4.47550957740264));
#20262=CARTESIAN_POINT('Ctrl Pts',(-1.91932437559004,0.684995961096763,
-4.30636138511347));
#20263=CARTESIAN_POINT('Ctrl Pts',(-1.95740679794227,0.608819659462652,
-4.22838203723553));
#20264=CARTESIAN_POINT('Ctrl Pts',(-2.02485323182035,0.430006700487909,
-4.1016362333799));
#20265=CARTESIAN_POINT('Ctrl Pts',(-2.05383693479979,0.327023915525715,
-4.05368786483531));
#20266=CARTESIAN_POINT('Ctrl Pts',(-2.08565111645498,0.116269187541378,
-4.00170605857396));
#20267=CARTESIAN_POINT('Ctrl Pts',(-2.09048597736785,0.013571707734776,
-3.99421211556224));
#20268=CARTESIAN_POINT('Ctrl Pts',(-2.07776710291235,-0.19148403344073,
-4.01460189690483));
#20269=CARTESIAN_POINT('Ctrl Pts',(-2.06053976427926,-0.289671925625125,
-4.04202503782963));
#20270=CARTESIAN_POINT('Ctrl Pts',(-2.00671918893296,-0.488728582767384,
-4.13487097478375));
#20271=CARTESIAN_POINT('Ctrl Pts',(-1.96758297172864,-0.584443608987603,
-4.20573850098139));
#20272=CARTESIAN_POINT('Ctrl Pts',(-1.88908829229803,-0.743279797016489,
-4.37887910454813));
#20273=CARTESIAN_POINT('Ctrl Pts',(-1.84955679967837,-0.806500365822468,
-4.48238860864025));
#20274=CARTESIAN_POINT('Ctrl Pts',(-1.80880106698392,-0.867867222875829,
-4.65409622882474));
#20275=CARTESIAN_POINT('Ctrl Pts',(-1.79841793711201,-0.882619607672314,
-4.71346892553171));
#20276=CARTESIAN_POINT('Ctrl Pts',(-1.78818429336492,-0.897056276598473,
-4.81607218145843));
#20277=CARTESIAN_POINT('Ctrl Pts',(-1.78605710994918,-0.9,-4.85793001834952));
#20278=CARTESIAN_POINT('Ctrl Pts',(-1.78605710994918,-0.9,-4.9));
#20279=CARTESIAN_POINT('Origin',(0.,0.,-5.));
#20280=CARTESIAN_POINT('',(3.74939945665464E-32,3.06161699786838E-16,0.));
#20281=CARTESIAN_POINT('Origin',(0.,0.,-5.));
#20282=CARTESIAN_POINT('Origin',(-5.,0.,-4.9));
#20283=CARTESIAN_POINT('',(-5.,0.9,-4.9));
#20284=CARTESIAN_POINT('Origin',(-2.1,1.212435565298,-27.8));
#20285=CARTESIAN_POINT('',(0.,2.424871130596,-32.2));
#20286=CARTESIAN_POINT('',(0.,2.424871130596,-27.8));
#20287=CARTESIAN_POINT('',(-2.1,1.212435565298,-32.2));
#20288=CARTESIAN_POINT('',(-2.1,1.212435565298,-32.2));
#20289=CARTESIAN_POINT('',(-2.1,1.212435565298,-27.8));
#20290=CARTESIAN_POINT('Origin',(-2.1,-1.212435565298,-27.8));
#20291=CARTESIAN_POINT('',(-2.1,-1.212435565298,-32.2));
#20292=CARTESIAN_POINT('',(-2.1,-1.212435565298,-32.2));
#20293=CARTESIAN_POINT('',(-2.1,-1.212435565298,-27.8));
#20294=CARTESIAN_POINT('Origin',(0.,-2.424871130596,-27.8));
#20295=CARTESIAN_POINT('',(0.,-2.424871130596,-32.2));
#20296=CARTESIAN_POINT('',(0.,-2.424871130596,-32.2));
#20297=CARTESIAN_POINT('',(0.,-2.424871130596,-27.8));
#20298=CARTESIAN_POINT('Origin',(2.1,-1.212435565298,-27.8));
#20299=CARTESIAN_POINT('',(2.1,-1.212435565298,-32.2));
#20300=CARTESIAN_POINT('',(2.1,-1.212435565298,-32.2));
#20301=CARTESIAN_POINT('',(2.1,-1.212435565298,-27.8));
#20302=CARTESIAN_POINT('Origin',(2.1,1.212435565298,-27.8));
#20303=CARTESIAN_POINT('',(2.1,1.212435565298,-32.2));
#20304=CARTESIAN_POINT('',(2.1,1.212435565298,-32.2));
#20305=CARTESIAN_POINT('',(2.1,1.212435565298,-27.8));
#20306=CARTESIAN_POINT('Origin',(0.,2.424871130596,-27.8));
#20307=CARTESIAN_POINT('',(0.,2.424871130596,-32.2));
#20308=CARTESIAN_POINT('Origin',(0.,0.,-32.2));
#20309=CARTESIAN_POINT('',(-1.37153434820004,-0.607366060714214,-32.2));
#20310=CARTESIAN_POINT('',(-1.37391623627015,-0.601217905938934,-32.2001711891269));
#20311=CARTESIAN_POINT('Ctrl Pts',(-1.37153434820004,-0.607366060714214,
-32.2));
#20312=CARTESIAN_POINT('Ctrl Pts',(-1.37242344863637,-0.605358322932482,
-32.2000570630423));
#20313=CARTESIAN_POINT('Ctrl Pts',(-1.37330814048737,-0.603348632866364,
-32.2001141260846));
#20314=CARTESIAN_POINT('Ctrl Pts',(-1.37418841522194,-0.601337009895288,
-32.2001711891269));
#20315=CARTESIAN_POINT('',(0.,-1.5,-32.2));
#20316=CARTESIAN_POINT('Origin',(0.,0.,-32.2));
#20317=CARTESIAN_POINT('',(-7.68260507571859E-6,-1.33950719362872,-32.1999496734209));
#20318=CARTESIAN_POINT('',(0.,-1.5,-32.2));
#20319=CARTESIAN_POINT('',(1.10953170738974,-0.35934403464,-32.1999624944555));
#20320=CARTESIAN_POINT('Ctrl Pts',(1.10946928894836,-0.359327399770989,
-32.2));
#20321=CARTESIAN_POINT('Ctrl Pts',(1.08903134641224,-0.463981924591757,
-32.2));
#20322=CARTESIAN_POINT('Ctrl Pts',(1.05178007571481,-0.581189099461517,
-32.2));
#20323=CARTESIAN_POINT('Ctrl Pts',(0.922701647259221,-0.812733731151359,
-32.2));
#20324=CARTESIAN_POINT('Ctrl Pts',(0.843132342414831,-0.913259848035649,
-32.2));
#20325=CARTESIAN_POINT('Ctrl Pts',(0.650405694031852,-1.09411325950692,
-32.2));
#20326=CARTESIAN_POINT('Ctrl Pts',(0.534709046647493,-1.17218209995489,
-32.2));
#20327=CARTESIAN_POINT('Ctrl Pts',(0.247987289255217,-1.30354237792863,
-32.2));
#20328=CARTESIAN_POINT('Ctrl Pts',(0.101385973706355,-1.32920597320179,
-32.2));
#20329=CARTESIAN_POINT('Ctrl Pts',(-1.53652101508341E-5,-1.33942086081202,
-32.2));
#20330=CARTESIAN_POINT('',(0.489601837133837,1.05872183713734,-32.2));
#20331=CARTESIAN_POINT('Ctrl Pts',(0.489601837133808,1.05872183713728,-32.2));
#20332=CARTESIAN_POINT('Ctrl Pts',(0.51857496980069,1.04522945410028,-32.2));
#20333=CARTESIAN_POINT('Ctrl Pts',(0.546708450841989,1.03069977102869,-32.2));
#20334=CARTESIAN_POINT('Ctrl Pts',(0.574079162507932,1.01517372385618,-32.2));
#20335=CARTESIAN_POINT('Ctrl Pts',(0.601788573860249,0.999455549150711,
-32.2));
#20336=CARTESIAN_POINT('Ctrl Pts',(0.628716837972728,0.982715812039489,
-32.2));
#20337=CARTESIAN_POINT('Ctrl Pts',(0.654924168246827,0.964947264141742,
-32.2));
#20338=CARTESIAN_POINT('Ctrl Pts',(0.671760176005753,0.953532465032388,
-32.2));
#20339=CARTESIAN_POINT('Ctrl Pts',(0.688298993318717,0.941691519760189,
-32.2));
#20340=CARTESIAN_POINT('Ctrl Pts',(0.704548179537464,0.929414759990573,
-32.2));
#20341=CARTESIAN_POINT('Ctrl Pts',(0.740116410445957,0.90254186799368,-32.2));
#20342=CARTESIAN_POINT('Ctrl Pts',(0.774270727515133,0.873591059770721,
-32.2));
#20343=CARTESIAN_POINT('Ctrl Pts',(0.806653680998004,0.842780534610089,
-32.2));
#20344=CARTESIAN_POINT('Ctrl Pts',(0.829132335967985,0.821393382110362,
-32.2));
#20345=CARTESIAN_POINT('Ctrl Pts',(0.850757926025641,0.799111125103228,
-32.2));
#20346=CARTESIAN_POINT('Ctrl Pts',(0.87142065334157,0.776018028800699,-32.2));
#20347=CARTESIAN_POINT('Ctrl Pts',(0.892050009827519,0.752962228435856,
-32.2));
#20348=CARTESIAN_POINT('Ctrl Pts',(0.911717446523677,0.729103354230809,
-32.2));
#20349=CARTESIAN_POINT('Ctrl Pts',(0.930361395902375,0.704476420442543,
-32.2));
#20350=CARTESIAN_POINT('Ctrl Pts',(0.951973732379004,0.675928521678787,
-32.2));
#20351=CARTESIAN_POINT('Ctrl Pts',(0.97221154496313,0.646348165623794,-32.2));
#20352=CARTESIAN_POINT('Ctrl Pts',(0.991051880052035,0.615842514725783,
-32.2));
#20353=CARTESIAN_POINT('Ctrl Pts',(1.00427160782397,0.594437566327873,-32.2));
#20354=CARTESIAN_POINT('Ctrl Pts',(1.01680423321371,0.572574415000461,-32.2));
#20355=CARTESIAN_POINT('Ctrl Pts',(1.02863277515403,0.550296487726837,-32.2));
#20356=CARTESIAN_POINT('Ctrl Pts',(1.05314560211509,0.504128922944566,-32.2));
#20357=CARTESIAN_POINT('Ctrl Pts',(1.07462078700313,0.456193592852453,-32.2));
#20358=CARTESIAN_POINT('Ctrl Pts',(1.09285040392536,0.407053468476931,-32.2));
#20359=CARTESIAN_POINT('Ctrl Pts',(1.11053719474954,0.359376597119088,-32.2));
#20360=CARTESIAN_POINT('Ctrl Pts',(1.12516803341667,0.310577100774157,-32.2));
#20361=CARTESIAN_POINT('Ctrl Pts',(1.13661646586548,0.261120445276902,-32.2));
#20362=CARTESIAN_POINT('Ctrl Pts',(1.14596056480605,0.220754405270782,-32.2));
#20363=CARTESIAN_POINT('Ctrl Pts',(1.15318470938534,0.179951383476785,-32.2));
#20364=CARTESIAN_POINT('Ctrl Pts',(1.15823093245761,0.138967806309482,-32.2));
#20365=CARTESIAN_POINT('Ctrl Pts',(1.16329511589048,0.0978383616658232,
-32.2));
#20366=CARTESIAN_POINT('Ctrl Pts',(1.16616787746435,0.0565354402705209,
-32.2));
#20367=CARTESIAN_POINT('Ctrl Pts',(1.16679746053248,0.015229310284014,-32.2));
#20368=CARTESIAN_POINT('Ctrl Pts',(1.16714856231426,-0.00780602305134579,
-32.2));
#20369=CARTESIAN_POINT('Ctrl Pts',(1.16680161359773,-0.030842710411849,
-32.2));
#20370=CARTESIAN_POINT('Ctrl Pts',(1.16574410749483,-0.0538519246251241,
-32.2));
#20371=CARTESIAN_POINT('Ctrl Pts',(1.1644894176962,-0.0811514610238715,
-32.2));
#20372=CARTESIAN_POINT('Ctrl Pts',(1.16223449940996,-0.108413071862421,
-32.2));
#20373=CARTESIAN_POINT('Ctrl Pts',(1.15900028857009,-0.135588564761368,
-32.2));
#20374=CARTESIAN_POINT('Ctrl Pts',(1.15502516959396,-0.168989546594902,
-32.2));
#20375=CARTESIAN_POINT('Ctrl Pts',(1.14957369981675,-0.20226703966678,-32.2));
#20376=CARTESIAN_POINT('Ctrl Pts',(1.14263928437902,-0.235446334559117,
-32.2));
#20377=CARTESIAN_POINT('Ctrl Pts',(1.13576030868238,-0.268360365344467,
-32.2));
#20378=CARTESIAN_POINT('Ctrl Pts',(1.12742174417963,-0.301178469756348,
-32.2));
#20379=CARTESIAN_POINT('Ctrl Pts',(1.11756964714795,-0.333907056427342,
-32.2));
#20380=CARTESIAN_POINT('Ctrl Pts',(1.1150161570307,-0.342389729948267,-32.2));
#20381=CARTESIAN_POINT('Ctrl Pts',(1.11236075568906,-0.350866262367389,
-32.2));
#20382=CARTESIAN_POINT('Ctrl Pts',(1.10960200800286,-0.359336469688434,
-32.2));
#20383=CARTESIAN_POINT('Ctrl Pts',(-1.37364723137695,-0.601091548606956,
-32.2));
#20384=CARTESIAN_POINT('Ctrl Pts',(-1.41239809287261,-0.485177618605703,
-32.2));
#20385=CARTESIAN_POINT('Ctrl Pts',(-1.43721913529673,-0.364224462906739,
-32.1999999999997));
#20386=CARTESIAN_POINT('Ctrl Pts',(-1.45443046115612,-0.12184967748929,
-32.1999999999997));
#20387=CARTESIAN_POINT('Ctrl Pts',(-1.44774454028095,-0.00120493111834647,
-32.1999999999997));
#20388=CARTESIAN_POINT('Ctrl Pts',(-1.39523776659632,0.289647590051206,
-32.1999999999997));
#20389=CARTESIAN_POINT('Ctrl Pts',(-1.33259337975644,0.457025994986103,
-32.2000000000004));
#20390=CARTESIAN_POINT('Ctrl Pts',(-1.14669279999604,0.757466021501395,
-32.2000000000004));
#20391=CARTESIAN_POINT('Ctrl Pts',(-1.02281858295675,0.889543113224934,
-32.2));
#20392=CARTESIAN_POINT('Ctrl Pts',(-0.739424758019696,1.09285013074389,
-32.2));
#20393=CARTESIAN_POINT('Ctrl Pts',(-0.585285031395165,1.16397131995923,
-32.1999999999995));
#20394=CARTESIAN_POINT('Ctrl Pts',(-0.259459731178378,1.23784226683936,
-32.1999999999995));
#20395=CARTESIAN_POINT('Ctrl Pts',(-0.0956654035339672,1.24352732441668,
-32.2000000000001));
#20396=CARTESIAN_POINT('Ctrl Pts',(0.258061421686738,1.18582051359148,-32.2000000000001));
#20397=CARTESIAN_POINT('Ctrl Pts',(0.39958824699244,1.11415800436119,-32.2));
#20398=CARTESIAN_POINT('Ctrl Pts',(0.489601837133914,1.05872183713747,-32.2));
#20399=CARTESIAN_POINT('Origin',(0.,0.,-32.2));
#20400=CARTESIAN_POINT('',(1.05931837406391E-5,-1.49970471981709,-32.1077344900145));
#20401=CARTESIAN_POINT('Ctrl Pts',(1.9414191012962E-5,-1.49999999987436,
-32.1079045323221));
#20402=CARTESIAN_POINT('Ctrl Pts',(-0.150756927286492,-1.50000195134149,
-32.1157211989316));
#20403=CARTESIAN_POINT('Ctrl Pts',(-0.300662543778459,-1.47727005913098,
-32.1239427369621));
#20404=CARTESIAN_POINT('Ctrl Pts',(-0.580589173772402,-1.39038854903977,
-32.1398124836169));
#20405=CARTESIAN_POINT('Ctrl Pts',(-0.709851208783395,-1.32905217388155,
-32.1472405420935));
#20406=CARTESIAN_POINT('Ctrl Pts',(-0.88710089333139,-1.21160584570517,
-32.1582276281382));
#20407=CARTESIAN_POINT('Ctrl Pts',(-0.942870535510222,-1.16873057217264,
-32.161844427991));
#20408=CARTESIAN_POINT('Ctrl Pts',(-1.05136504230531,-1.07248447363525,
-32.1695118574188));
#20409=CARTESIAN_POINT('Ctrl Pts',(-1.10351027642,-1.01875172871345,-32.1735838961206));
#20410=CARTESIAN_POINT('Ctrl Pts',(-1.24091513632039,-0.854180765807274,
-32.1852578166437));
#20411=CARTESIAN_POINT('Ctrl Pts',(-1.31499941955155,-0.735031403791276,
-32.1927319272353));
#20412=CARTESIAN_POINT('Ctrl Pts',(-1.37153434820004,-0.607366060714214,
-32.2));
#20413=CARTESIAN_POINT('',(0.,-1.5,-32.1078125));
#20414=CARTESIAN_POINT('Ctrl Pts',(-0.9683606883504,0.5860878712161,-30.56360688769));
#20415=CARTESIAN_POINT('Ctrl Pts',(-0.841941231244,0.7949637727945,-30.58077178948));
#20416=CARTESIAN_POINT('Ctrl Pts',(-0.4496074219719,1.12727586262,-30.61510159306));
#20417=CARTESIAN_POINT('Ctrl Pts',(0.3210196062211,1.170506932088,-30.66659629844));
#20418=CARTESIAN_POINT('Ctrl Pts',(0.9617584207716,0.7403170710639,-30.71809100381));
#20419=CARTESIAN_POINT('Ctrl Pts',(1.213652727685,0.01083402249656,-30.76958570919));
#20420=CARTESIAN_POINT('Ctrl Pts',(0.9748232760455,-0.7230402406274,-30.82108041456));
#20421=CARTESIAN_POINT('Ctrl Pts',(0.3418443908816,-1.164564134257,-30.87257511994));
#20422=CARTESIAN_POINT('Ctrl Pts',(-0.4293532065945,-1.135219537988,-30.92406982531));
#20423=CARTESIAN_POINT('Ctrl Pts',(-1.026949913989,-0.6468704059859,-30.97556453069));
#20424=CARTESIAN_POINT('Ctrl Pts',(-1.20931907835,0.1030283602118,-31.02705923606));
#20425=CARTESIAN_POINT('Ctrl Pts',(-0.9027231702267,0.8112695922203,-31.07855394144));
#20426=CARTESIAN_POINT('Ctrl Pts',(-0.2311283984392,1.191489461132,-31.13004864681));
#20427=CARTESIAN_POINT('Ctrl Pts',(0.5339187258583,1.089953332612,-31.18154335219));
#20428=CARTESIAN_POINT('Ctrl Pts',(1.083086014468,0.5477153988916,-31.23303805756));
#20429=CARTESIAN_POINT('Ctrl Pts',(1.194328167088,-0.2159807914049,-31.28453276294));
#20430=CARTESIAN_POINT('Ctrl Pts',(0.8226665446893,-0.8923492753407,-31.33602746831));
#20431=CARTESIAN_POINT('Ctrl Pts',(0.1183754231753,-1.207913379402,-31.38752217369));
#20432=CARTESIAN_POINT('Ctrl Pts',(-0.6337785389668,-1.035080787425,-31.43901687906));
#20433=CARTESIAN_POINT('Ctrl Pts',(-1.129676258131,-0.4437330557542,-31.49051158444));
#20434=CARTESIAN_POINT('Ctrl Pts',(-1.168810966393,0.3270296588359,-31.54200628981));
#20435=CARTESIAN_POINT('Ctrl Pts',(-0.7353592922662,0.9655641793129,-31.59350099519));
#20436=CARTESIAN_POINT('Ctrl Pts',(-0.004579138184,1.213691272131,-31.64499570056));
#20437=CARTESIAN_POINT('Ctrl Pts',(0.7280525020971,0.9710854892931,-31.69649040594));
#20438=CARTESIAN_POINT('Ctrl Pts',(1.16631002676,0.335839839429,-31.74798511131));
#20439=CARTESIAN_POINT('Ctrl Pts',(1.132992364504,-0.4351962200625,-31.79947981669));
#20440=CARTESIAN_POINT('Ctrl Pts',(0.641570930501,-1.030269050578,-31.85097452206));
#20441=CARTESIAN_POINT('Ctrl Pts',(-0.1092576130587,-1.208772097777,-31.90246922744));
#20442=CARTESIAN_POINT('Ctrl Pts',(-0.8159093239228,-0.8985319049552,-31.95396393281));
#20443=CARTESIAN_POINT('Ctrl Pts',(-1.192665944352,-0.2249850320436,-32.00545863819));
#20444=CARTESIAN_POINT('Ctrl Pts',(-1.087182459866,0.539521014043,-32.05695334356));
#20445=CARTESIAN_POINT('Ctrl Pts',(-0.5421489359955,1.085916477839,-32.10844804894));
#20446=CARTESIAN_POINT('Ctrl Pts',(0.2222093980149,1.193113862031,-32.15994275432));
#20447=CARTESIAN_POINT('Ctrl Pts',(0.6715924913568,0.9432899673364,-32.1942725579));
#20448=CARTESIAN_POINT('Ctrl Pts',(0.83615698899,0.762930472122,-32.21143745969));
#20449=CARTESIAN_POINT('Ctrl Pts',(-1.0833316035,0.6556725411871,-30.64119627189));
#20450=CARTESIAN_POINT('Ctrl Pts',(-0.9419026970726,0.8893477286577,-30.65836117369));
#20451=CARTESIAN_POINT('Ctrl Pts',(-0.5029881275127,1.261114358038,-30.69269097727));
#20452=CARTESIAN_POINT('Ctrl Pts',(0.3591334189276,1.309478138571,-30.74418568264));
#20453=CARTESIAN_POINT('Ctrl Pts',(1.075945466073,0.8282129678975,-30.79568038802));
#20454=CARTESIAN_POINT('Ctrl Pts',(1.35774652089,0.01212031746512,-30.84717509339));
#20455=CARTESIAN_POINT('Ctrl Pts',(1.090561477218,-0.8088849048676,-30.89866979877));
#20456=CARTESIAN_POINT('Ctrl Pts',(0.382430675446,-1.302829767999,-30.95016450414));
#20457=CARTESIAN_POINT('Ctrl Pts',(-0.4803291824663,-1.27000116507,-31.00165920952));
#20458=CARTESIAN_POINT('Ctrl Pts',(-1.148876973652,-0.7236716262895,-31.05315391489));
#20459=CARTESIAN_POINT('Ctrl Pts',(-1.352898348779,0.1152606461796,-31.10464862027));
#20460=CARTESIAN_POINT('Ctrl Pts',(-1.009901115652,0.907589495096,-31.15614332565));
#20461=CARTESIAN_POINT('Ctrl Pts',(-0.2585696647001,1.332951868048,-31.20763803102));
#20462=CARTESIAN_POINT('Ctrl Pts',(0.5973094905453,1.219360622301,-31.2591327364));
#20463=CARTESIAN_POINT('Ctrl Pts',(1.211677965553,0.6127442062457,-31.31062744177));
#20464=CARTESIAN_POINT('Ctrl Pts',(1.336127606089,-0.2416236221613,-31.36212214715));
#20465=CARTESIAN_POINT('Ctrl Pts',(0.9203395777271,-0.9982955555368,-31.41361685252));
#20466=CARTESIAN_POINT('Ctrl Pts',(0.132429825525,-1.351325754896,-31.4651115579));
#20467=CARTESIAN_POINT('Ctrl Pts',(-0.7090253963658,-1.157973204286,-31.51660626327));
#20468=CARTESIAN_POINT('Ctrl Pts',(-1.26379974619,-0.4964163132592,-31.56810096865));
#20469=CARTESIAN_POINT('Ctrl Pts',(-1.307580815334,0.3658570292669,-31.61959567402));
#20470=CARTESIAN_POINT('Ctrl Pts',(-0.8226665650754,1.080203072307,-31.6710903794));
#20471=CARTESIAN_POINT('Ctrl Pts',(-0.005122807205206,1.357789641617,-31.72258508477));
#20472=CARTESIAN_POINT('Ctrl Pts',(0.8144922589459,1.086379912885,-31.77407979015));
#20473=CARTESIAN_POINT('Ctrl Pts',(1.304782945723,0.3757132194075,-31.82557449552));
#20474=CARTESIAN_POINT('Ctrl Pts',(1.267509565142,-0.4868659215406,-31.8770692009));
#20475=CARTESIAN_POINT('Ctrl Pts',(0.7177429580321,-1.15259018259,-31.92856390627));
#20476=CARTESIAN_POINT('Ctrl Pts',(-0.1222294818174,-1.352286426643,-31.98005861165));
#20477=CARTESIAN_POINT('Ctrl Pts',(-0.9127800899286,-1.005212232489,-32.03155331702));
#20478=CARTESIAN_POINT('Ctrl Pts',(-1.334268032024,-0.2516969125858,-32.0830480224));
#20479=CARTESIAN_POINT('Ctrl Pts',(-1.216260771128,0.6035769236572,-32.13454272777));
#20480=CARTESIAN_POINT('Ctrl Pts',(-0.6065168518646,1.214844482388,-32.18603743315));
#20481=CARTESIAN_POINT('Ctrl Pts',(0.2485917348362,1.33476912979,-32.23753213852));
#20482=CARTESIAN_POINT('Ctrl Pts',(0.7513288997713,1.055284301783,-32.27186194211));
#20483=CARTESIAN_POINT('Ctrl Pts',(0.9354317069637,0.8535111985296,-32.2890268439));
#20484=CARTESIAN_POINT('Ctrl Pts',(-1.198302518649,0.7252572111581,-30.7187856561));
#20485=CARTESIAN_POINT('Ctrl Pts',(-1.041864162901,0.9837316845208,-30.73595055789));
#20486=CARTESIAN_POINT('Ctrl Pts',(-0.5563688330535,1.394952853457,-30.77028036148));
#20487=CARTESIAN_POINT('Ctrl Pts',(0.3972472316341,1.448449345054,-30.82177506685));
#20488=CARTESIAN_POINT('Ctrl Pts',(1.190132511375,0.9161088647312,-30.87326977223));
#20489=CARTESIAN_POINT('Ctrl Pts',(1.501840314096,0.01340661243369,-30.9247644776));
#20490=CARTESIAN_POINT('Ctrl Pts',(1.206299678391,-0.8947295691077,-30.97625918298));
#20491=CARTESIAN_POINT('Ctrl Pts',(0.4230169600104,-1.441095401742,-31.02775388835));
#20492=CARTESIAN_POINT('Ctrl Pts',(-0.5313051583381,-1.404782792152,-31.07924859373));
#20493=CARTESIAN_POINT('Ctrl Pts',(-1.270804033315,-0.800472846593,-31.1307432991));
#20494=CARTESIAN_POINT('Ctrl Pts',(-1.496477619208,0.1274929321474,-31.18223800448));
#20495=CARTESIAN_POINT('Ctrl Pts',(-1.117079061076,1.003909397972,-31.23373270985));
#20496=CARTESIAN_POINT('Ctrl Pts',(-0.2860109309609,1.474414274964,-31.28522741523));
#20497=CARTESIAN_POINT('Ctrl Pts',(0.6607002552323,1.34876791199,-31.3367221206));
#20498=CARTESIAN_POINT('Ctrl Pts',(1.340269916638,0.6777730135999,-31.38821682598));
#20499=CARTESIAN_POINT('Ctrl Pts',(1.47792704509,-0.2672664529177,-31.43971153135));
#20500=CARTESIAN_POINT('Ctrl Pts',(1.018012610765,-1.104241835733,-31.49120623673));
#20501=CARTESIAN_POINT('Ctrl Pts',(0.1464842278746,-1.494738130389,-31.5427009421));
#20502=CARTESIAN_POINT('Ctrl Pts',(-0.7842722537648,-1.280865621146,-31.59419564748));
#20503=CARTESIAN_POINT('Ctrl Pts',(-1.397923234248,-0.5490995707643,-31.64569035285));
#20504=CARTESIAN_POINT('Ctrl Pts',(-1.446350664275,0.4046843996979,-31.69718505823));
#20505=CARTESIAN_POINT('Ctrl Pts',(-0.9099738378846,1.1948419653,-31.7486797636));
#20506=CARTESIAN_POINT('Ctrl Pts',(-0.005666476226419,1.501888011103,-31.80017446898));
#20507=CARTESIAN_POINT('Ctrl Pts',(0.9009320157947,1.201674336477,-31.85166917435));
#20508=CARTESIAN_POINT('Ctrl Pts',(1.443255864685,0.415586599386,-31.90316387973));
#20509=CARTESIAN_POINT('Ctrl Pts',(1.40202676578,-0.5385356230187,-31.95465858511));
#20510=CARTESIAN_POINT('Ctrl Pts',(0.7939149855631,-1.274911314603,-32.00615329048));
#20511=CARTESIAN_POINT('Ctrl Pts',(-0.1352013505761,-1.495800755509,-32.05764799586));
#20512=CARTESIAN_POINT('Ctrl Pts',(-1.009650855934,-1.111892560022,-32.10914270123));
#20513=CARTESIAN_POINT('Ctrl Pts',(-1.475870119695,-0.2784087931281,-32.16063740661));
#20514=CARTESIAN_POINT('Ctrl Pts',(-1.345339082391,0.6676328332714,-32.21213211198));
#20515=CARTESIAN_POINT('Ctrl Pts',(-0.6708847677338,1.343772486938,-32.26362681736));
#20516=CARTESIAN_POINT('Ctrl Pts',(0.2749740716576,1.476424397549,-32.31512152273));
#20517=CARTESIAN_POINT('Ctrl Pts',(0.8310653081857,1.16727863623,-32.34945132631));
#20518=CARTESIAN_POINT('Ctrl Pts',(1.034706424937,0.9440919249371,-32.36661622811));
#20519=CARTESIAN_POINT('Ctrl Pts',(-1.313273433799,0.794841881129,-30.79637504031));
#20520=CARTESIAN_POINT('Ctrl Pts',(-1.14182562873,1.078115640384,-30.8135399421));
#20521=CARTESIAN_POINT('Ctrl Pts',(-0.6097495385943,1.528791348876,-30.84786974568));
#20522=CARTESIAN_POINT('Ctrl Pts',(0.4353610443407,1.587420551537,-30.89936445106));
#20523=CARTESIAN_POINT('Ctrl Pts',(1.304319556676,1.004004761565,-30.95085915644));
#20524=CARTESIAN_POINT('Ctrl Pts',(1.645934107302,0.01469290740225,-31.00235386181));
#20525=CARTESIAN_POINT('Ctrl Pts',(1.322037879563,-0.9805742333479,-31.05384856719));
#20526=CARTESIAN_POINT('Ctrl Pts',(0.4636032445749,-1.579361035484,-31.10534327256));
#20527=CARTESIAN_POINT('Ctrl Pts',(-0.5822811342099,-1.539564419234,-31.15683797794));
#20528=CARTESIAN_POINT('Ctrl Pts',(-1.392731092978,-0.8772740668966,-31.20833268331));
#20529=CARTESIAN_POINT('Ctrl Pts',(-1.640056889637,0.1397252181152,-31.25982738869));
#20530=CARTESIAN_POINT('Ctrl Pts',(-1.224257006501,1.100229300847,-31.31132209406));
#20531=CARTESIAN_POINT('Ctrl Pts',(-0.3134521972218,1.615876681881,-31.36281679944));
#20532=CARTESIAN_POINT('Ctrl Pts',(0.7240910199193,1.478175201679,-31.41431150481));
#20533=CARTESIAN_POINT('Ctrl Pts',(1.468861867722,0.742801820954,-31.46580621019));
#20534=CARTESIAN_POINT('Ctrl Pts',(1.619726484091,-0.2929092836741,-31.51730091556));
#20535=CARTESIAN_POINT('Ctrl Pts',(1.115685643803,-1.210188115929,-31.56879562094));
#20536=CARTESIAN_POINT('Ctrl Pts',(0.1605386302243,-1.638150505883,-31.62029032631));
#20537=CARTESIAN_POINT('Ctrl Pts',(-0.8595191111638,-1.403758038006,-31.67178503169));
#20538=CARTESIAN_POINT('Ctrl Pts',(-1.532046722306,-0.6017828282693,-31.72327973706));
#20539=CARTESIAN_POINT('Ctrl Pts',(-1.585120513216,0.4435117701289,-31.77477444244));
#20540=CARTESIAN_POINT('Ctrl Pts',(-0.9972811106938,1.309480858294,-31.82626914781));
#20541=CARTESIAN_POINT('Ctrl Pts',(-0.006210145247626,1.645986380589,-31.87776385319));
#20542=CARTESIAN_POINT('Ctrl Pts',(0.9873717726436,1.316968760069,-31.92925855856));
#20543=CARTESIAN_POINT('Ctrl Pts',(1.581728783648,0.4554599793645,-31.98075326394));
#20544=CARTESIAN_POINT('Ctrl Pts',(1.536543966417,-0.5902053244968,-32.03224796931));
#20545=CARTESIAN_POINT('Ctrl Pts',(0.8700870130942,-1.397232446615,-32.08374267469));
#20546=CARTESIAN_POINT('Ctrl Pts',(-0.1481732193349,-1.639315084374,-32.13523738006));
#20547=CARTESIAN_POINT('Ctrl Pts',(-1.10652162194,-1.218572887555,-32.18673208544));
#20548=CARTESIAN_POINT('Ctrl Pts',(-1.617472207367,-0.3051206736703,-32.23822679081));
#20549=CARTESIAN_POINT('Ctrl Pts',(-1.474417393653,0.7316887428856,-32.28972149619));
#20550=CARTESIAN_POINT('Ctrl Pts',(-0.7352526836029,1.472700491487,-32.34121620156));
#20551=CARTESIAN_POINT('Ctrl Pts',(0.3013564084789,1.618079665308,-32.39271090694));
#20552=CARTESIAN_POINT('Ctrl Pts',(0.9108017166002,1.279272970676,-32.42704071052));
#20553=CARTESIAN_POINT('Ctrl Pts',(1.133981142911,1.034672651345,-32.44420561231));
#20554=CARTESIAN_POINT('',(-0.685937500187104,0.944111968542343,-30.6155198486503));
#20555=CARTESIAN_POINT('Ctrl Pts',(-0.685549818356495,0.943589307941825,
-30.6154432565738));
#20556=CARTESIAN_POINT('Ctrl Pts',(-0.58064605296268,1.02007511987387,-30.6243229170041));
#20557=CARTESIAN_POINT('Ctrl Pts',(-0.444206516756635,1.09392715892444,
-30.6348232653003));
#20558=CARTESIAN_POINT('Ctrl Pts',(-0.123013026528223,1.16966346430087,
-30.6572180841587));
#20559=CARTESIAN_POINT('Ctrl Pts',(0.0323543525080591,1.1755099489028,-30.6674551876461));
#20560=CARTESIAN_POINT('Ctrl Pts',(0.272129692413745,1.13820198274907,-30.6841062976065));
#20561=CARTESIAN_POINT('Ctrl Pts',(0.35976297016591,1.11401115078793,-30.6904574701318));
#20562=CARTESIAN_POINT('Ctrl Pts',(0.515514067421646,1.04955883562299,-30.7020015367485));
#20563=CARTESIAN_POINT('Ctrl Pts',(0.583848005518145,1.01277911064057,-30.7071896615724));
#20564=CARTESIAN_POINT('Ctrl Pts',(0.724546181506395,0.918370978969335,
-30.7185554543531));
#20565=CARTESIAN_POINT('Ctrl Pts',(0.795191272615342,0.858032542126043,
-30.7247396075133));
#20566=CARTESIAN_POINT('Ctrl Pts',(0.962172388622911,0.677781105774433,
-30.7415978089187));
#20567=CARTESIAN_POINT('Ctrl Pts',(1.04182541894227,0.547667974612751,-30.7522459281879));
#20568=CARTESIAN_POINT('Ctrl Pts',(1.12323761388946,0.324738122282939,-30.7680872244194));
#20569=CARTESIAN_POINT('Ctrl Pts',(1.14355889053653,0.243126408867936,-30.7736158882269));
#20570=CARTESIAN_POINT('Ctrl Pts',(1.16583991182123,0.0841465040768233,
-30.7844711483562));
#20571=CARTESIAN_POINT('Ctrl Pts',(1.16913809492736,0.00689646112748725,
-30.7898296388345));
#20572=CARTESIAN_POINT('Ctrl Pts',(1.16222537935487,-0.113540683276614,
-30.7983737162774));
#20573=CARTESIAN_POINT('Ctrl Pts',(1.15723001531888,-0.157076089779638,
-30.8014697176085));
#20574=CARTESIAN_POINT('Ctrl Pts',(1.13490702072137,-0.284498729207274,
-30.8103909766174));
#20575=CARTESIAN_POINT('Ctrl Pts',(1.11060620210311,-0.36691443612988,-30.8160317748216));
#20576=CARTESIAN_POINT('Ctrl Pts',(1.04510048542586,-0.524311586158876,
-30.827298666073));
#20577=CARTESIAN_POINT('Ctrl Pts',(1.00394780872658,-0.599371546138324,
-30.8329348435321));
#20578=CARTESIAN_POINT('Ctrl Pts',(0.921020285080622,-0.718350217423981,
-30.8429575993004));
#20579=CARTESIAN_POINT('Ctrl Pts',(0.882990259693012,-0.76494679049744,
-30.8472534440817));
#20580=CARTESIAN_POINT('Ctrl Pts',(0.815751820700548,-0.835292827709003,
-30.8541625266585));
#20581=CARTESIAN_POINT('Ctrl Pts',(0.788600249269866,-0.861057780772529,
-30.8567974562499));
#20582=CARTESIAN_POINT('Ctrl Pts',(0.704840482900919,-0.932860902847456,
-30.8643865651111));
#20583=CARTESIAN_POINT('Ctrl Pts',(0.644987568932664,-0.974856777009102,
-30.8691842871257));
#20584=CARTESIAN_POINT('Ctrl Pts',(0.516425892376748,-1.04837375477001,
-30.8789144838574));
#20585=CARTESIAN_POINT('Ctrl Pts',(0.4474710934552,-1.07950036803969,-30.8838515782429));
#20586=CARTESIAN_POINT('Ctrl Pts',(0.322697231458926,-1.12218677030221,
-30.8928435994936));
#20587=CARTESIAN_POINT('Ctrl Pts',(0.267843862426517,-1.13669200069658,
-30.896846619438));
#20588=CARTESIAN_POINT('Ctrl Pts',(0.168539599695823,-1.15537506229575,
-30.9040510091863));
#20589=CARTESIAN_POINT('Ctrl Pts',(0.12437129358316,-1.16109940910304,-30.9072314578863));
#20590=CARTESIAN_POINT('Ctrl Pts',(0.04002917364263,-1.16701286980662,-30.9131523317177));
#20591=CARTESIAN_POINT('Ctrl Pts',(0.00014785501451689,-1.16766543747708,
-30.9158750267731));
#20592=CARTESIAN_POINT('Ctrl Pts',(-0.120399774363236,-1.16329491837156,
-30.9239498325746));
#20593=CARTESIAN_POINT('Ctrl Pts',(-0.200704815239112,-1.151826505131,-30.9291490667603));
#20594=CARTESIAN_POINT('Ctrl Pts',(-0.315214160338411,-1.12341563756021,
-30.9369298719994));
#20595=CARTESIAN_POINT('Ctrl Pts',(-0.350995565090333,-1.11273069881691,
-30.9394161098036));
#20596=CARTESIAN_POINT('Ctrl Pts',(-0.457319408159109,-1.07547579278067,
-30.9470914368855));
#20597=CARTESIAN_POINT('Ctrl Pts',(-0.526092532709015,-1.043814098234,-30.9525024051635));
#20598=CARTESIAN_POINT('Ctrl Pts',(-0.637601397105962,-0.978724537033635,
-30.9617031731051));
#20599=CARTESIAN_POINT('Ctrl Pts',(-0.682226149753855,-0.948353027567811,
-30.9655138607647));
#20600=CARTESIAN_POINT('Ctrl Pts',(-0.776257227460013,-0.873838007781977,
-30.9736876405209));
#20601=CARTESIAN_POINT('Ctrl Pts',(-0.824357288478918,-0.828279102352816,
-30.9779858533615));
#20602=CARTESIAN_POINT('Ctrl Pts',(-0.910617501933913,-0.731559492611122,
-30.9864321791417));
#20603=CARTESIAN_POINT('Ctrl Pts',(-0.949079289481939,-0.680674445423622,
-30.9905825954745));
#20604=CARTESIAN_POINT('Ctrl Pts',(-1.02513338266168,-0.56138353942896,
-31.000216709631));
#20605=CARTESIAN_POINT('Ctrl Pts',(-1.06060237636569,-0.49155930001184,
-31.0058072822228));
#20606=CARTESIAN_POINT('Ctrl Pts',(-1.10962744691463,-0.365287132932502,
-31.0154453787039));
#20607=CARTESIAN_POINT('Ctrl Pts',(-1.12649192979211,-0.310091614787038,
-31.0195135341267));
#20608=CARTESIAN_POINT('Ctrl Pts',(-1.15268125864006,-0.192731992657596,
-31.0276959783734));
#20609=CARTESIAN_POINT('Ctrl Pts',(-1.16115789218137,-0.13051886757346,
-31.0317727346732));
#20610=CARTESIAN_POINT('Ctrl Pts',(-1.16791178975008,-0.00868033034464753,
-31.0397150790911));
#20611=CARTESIAN_POINT('Ctrl Pts',(-1.1666680633032,0.0509752084799933,
-31.0435873391708));
#20612=CARTESIAN_POINT('Ctrl Pts',(-1.15467348304469,0.17617947896303,-31.0521400991318));
#20613=CARTESIAN_POINT('Ctrl Pts',(-1.14284908742083,0.241656664267984,
-31.0568344967498));
#20614=CARTESIAN_POINT('Ctrl Pts',(-1.10763145439615,0.372687281057628,
-31.0664668348878));
#20615=CARTESIAN_POINT('Ctrl Pts',(-1.08370537416884,0.438139495945055,
-31.0714053450789));
#20616=CARTESIAN_POINT('Ctrl Pts',(-1.02026614664799,0.572107606135475,
-31.0815641621441));
#20617=CARTESIAN_POINT('Ctrl Pts',(-0.979287244981931,0.639164520306697,
-31.0866104510614));
#20618=CARTESIAN_POINT('Ctrl Pts',(-0.910536559022417,0.729969026199407,
-31.0940487006932));
#20619=CARTESIAN_POINT('Ctrl Pts',(-0.887588763253689,0.757550902676565,
-31.0964059553973));
#20620=CARTESIAN_POINT('Ctrl Pts',(-0.79318341488161,0.861115385835129,
-31.105836469407));
#20621=CARTESIAN_POINT('Ctrl Pts',(-0.712708892211407,0.929007678350079,
-31.1133048282032));
#20622=CARTESIAN_POINT('Ctrl Pts',(-0.586676199099358,1.00947261785909,
-31.1238366894391));
#20623=CARTESIAN_POINT('Ctrl Pts',(-0.54711709638151,1.03161773821077,-31.1270017225964));
#20624=CARTESIAN_POINT('Ctrl Pts',(-0.447880028777928,1.07963910147511,
-31.1345515613862));
#20625=CARTESIAN_POINT('Ctrl Pts',(-0.387510472693664,1.10260994906124,
-31.1387701787857));
#20626=CARTESIAN_POINT('Ctrl Pts',(-0.284851937819151,1.13211115662808,
-31.1457492890684));
#20627=CARTESIAN_POINT('Ctrl Pts',(-0.243599465079629,1.14155657530597,
-31.1485177707169));
#20628=CARTESIAN_POINT('Ctrl Pts',(-0.128297940424894,1.16153184398187,
-31.1563826813405));
#20629=CARTESIAN_POINT('Ctrl Pts',(-0.05339768760864,1.16731338199176,-31.1616009318968));
#20630=CARTESIAN_POINT('Ctrl Pts',(0.0892765697898679,1.1649149779081,-31.1716159041541));
#20631=CARTESIAN_POINT('Ctrl Pts',(0.15714162457393,1.15795513700009,-31.1764096565917));
#20632=CARTESIAN_POINT('Ctrl Pts',(0.278664991070919,1.13454883807076,-31.1849605518862));
#20633=CARTESIAN_POINT('Ctrl Pts',(0.332653037305334,1.12002949667963,-31.1887346689173));
#20634=CARTESIAN_POINT('Ctrl Pts',(0.433816672891627,1.0844438029925,-31.1958147743426));
#20635=CARTESIAN_POINT('Ctrl Pts',(0.480820518649546,1.06424943532574,-31.1991383315904));
#20636=CARTESIAN_POINT('Ctrl Pts',(0.64177924230017,0.982275042229206,-31.2112090255195));
#20637=CARTESIAN_POINT('Ctrl Pts',(0.747625313053594,0.904251732343868,
-31.2203661560253));
#20638=CARTESIAN_POINT('Ctrl Pts',(0.880907974589085,0.767383596728147,
-31.2336520510528));
#20639=CARTESIAN_POINT('Ctrl Pts',(0.920355842015236,0.719964895099076,
-31.2378964628582));
#20640=CARTESIAN_POINT('Ctrl Pts',(0.994030870573145,0.615094816078788,
-31.2465511819434));
#20641=CARTESIAN_POINT('Ctrl Pts',(1.02719182235098,0.557521893428536,-31.2508737135115));
#20642=CARTESIAN_POINT('Ctrl Pts',(1.11651848045971,0.36662271234126,-31.2650086372261));
#20643=CARTESIAN_POINT('Ctrl Pts',(1.15347382627016,0.22401192173484,-31.2751414931434));
#20644=CARTESIAN_POINT('Ctrl Pts',(1.1744576386023,-0.0697605175983266,
-31.2954708383108));
#20645=CARTESIAN_POINT('Ctrl Pts',(1.15618399361287,-0.217343368572523,
-31.3051565938156));
#20646=CARTESIAN_POINT('Ctrl Pts',(1.06334090087441,-0.501175404200165,
-31.3254700203755));
#20647=CARTESIAN_POINT('Ctrl Pts',(0.990072860789148,-0.634244960097407,
-31.3357877022529));
#20648=CARTESIAN_POINT('Ctrl Pts',(0.779939960671839,-0.886826667173546,
-31.3582916167791));
#20649=CARTESIAN_POINT('Ctrl Pts',(0.651195811249931,-0.976393206170076,
-31.3686325822348));
#20650=CARTESIAN_POINT('Ctrl Pts',(0.40465076484607,-1.10348922038188,-31.3874884713758));
#20651=CARTESIAN_POINT('Ctrl Pts',(0.26067210257786,-1.14683252718141,-31.3975848541239));
#20652=CARTESIAN_POINT('Ctrl Pts',(0.0414129321920925,-1.1685833647203,
-31.4127775461669));
#20653=CARTESIAN_POINT('Ctrl Pts',(-0.0311611824591641,-1.16863904701939,
-31.4177144778021));
#20654=CARTESIAN_POINT('Ctrl Pts',(-0.250957175467129,-1.14849060721418,
-31.4326611289385));
#20655=CARTESIAN_POINT('Ctrl Pts',(-0.396566537627489,-1.10667316158768,
-31.44261757239));
#20656=CARTESIAN_POINT('Ctrl Pts',(-0.638350257118472,-0.98452433640704,
-31.461266651544));
#20657=CARTESIAN_POINT('Ctrl Pts',(-0.736541623239782,-0.913407391716465,
-31.4696968846861));
#20658=CARTESIAN_POINT('Ctrl Pts',(-0.923384755992755,-0.726303779689699,
-31.4875096033724));
#20659=CARTESIAN_POINT('Ctrl Pts',(-1.0055723746581,-0.607329676628576,
-31.4968989787272));
#20660=CARTESIAN_POINT('Ctrl Pts',(-1.0936762524601,-0.412696282653138,
-31.5116737635136));
#20661=CARTESIAN_POINT('Ctrl Pts',(-1.11727838553113,-0.344659613610039,
-31.5168039971177));
#20662=CARTESIAN_POINT('Ctrl Pts',(-1.14616299763878,-0.225186641674113,
-31.5253254635316));
#20663=CARTESIAN_POINT('Ctrl Pts',(-1.15476615560226,-0.174808565363235,
-31.5287817978504));
#20664=CARTESIAN_POINT('Ctrl Pts',(-1.16753840461434,-0.0518871225375712,
-31.5370652043289));
#20665=CARTESIAN_POINT('Ctrl Pts',(-1.16829471715105,0.0210179048571228,
-31.5418549401139));
#20666=CARTESIAN_POINT('Ctrl Pts',(-1.15703286837474,0.160510799516341,
-31.5511950587481));
#20667=CARTESIAN_POINT('Ctrl Pts',(-1.14592336273605,0.227225796083613,
-31.5557428617876));
#20668=CARTESIAN_POINT('Ctrl Pts',(-1.11662488052543,0.3416742850202,-31.5639576111054));
#20669=CARTESIAN_POINT('Ctrl Pts',(-1.10084925783999,0.390046111141884,
-31.567582314457));
#20670=CARTESIAN_POINT('Ctrl Pts',(-1.06334533384066,0.483414957899083,
-31.5747012168093));
#20671=CARTESIAN_POINT('Ctrl Pts',(-1.04188770919863,0.528059829950944,
-31.5781420352983));
#20672=CARTESIAN_POINT('Ctrl Pts',(-0.991356486728722,0.617571049953205,
-31.5851109376138));
#20673=CARTESIAN_POINT('Ctrl Pts',(-0.96211461432135,0.661875222634075,
-31.5886220053224));
#20674=CARTESIAN_POINT('Ctrl Pts',(-0.875015979693796,0.776286059444753,
-31.5981155690734));
#20675=CARTESIAN_POINT('Ctrl Pts',(-0.811616460796327,0.842239001467981,
-31.6040805899385));
#20676=CARTESIAN_POINT('Ctrl Pts',(-0.707260818464706,0.928555454565463,
-31.6133843286188));
#20677=CARTESIAN_POINT('Ctrl Pts',(-0.671285275966235,0.955051098604024,
-31.6165309479633));
#20678=CARTESIAN_POINT('Ctrl Pts',(-0.576842243397548,1.01658449168296,
-31.6245495281119));
#20679=CARTESIAN_POINT('Ctrl Pts',(-0.516407878498177,1.04883047882692,
-31.6294318125191));
#20680=CARTESIAN_POINT('Ctrl Pts',(-0.386933712951129,1.1031863842945,-31.6390086889994));
#20681=CARTESIAN_POINT('Ctrl Pts',(-0.318197534791427,1.12464209428096,
-31.6437060028805));
#20682=CARTESIAN_POINT('Ctrl Pts',(-0.176551057827588,1.15509542084064,
-31.6532098441827));
#20683=CARTESIAN_POINT('Ctrl Pts',(-0.103562879627239,1.16383625984169,
-31.6580222417704));
#20684=CARTESIAN_POINT('Ctrl Pts',(0.00757975185125543,1.16688101758023,
-31.6656505014464));
#20685=CARTESIAN_POINT('Ctrl Pts',(0.0456383690066451,1.16610227706485,
-31.6683241575286));
#20686=CARTESIAN_POINT('Ctrl Pts',(0.166807315161587,1.15774406385772,-31.6769512638621));
#20687=CARTESIAN_POINT('Ctrl Pts',(0.249701555193096,1.1431299277067,-31.6829994302105));
#20688=CARTESIAN_POINT('Ctrl Pts',(0.365039122436339,1.10896345331728,-31.6911740597271));
#20689=CARTESIAN_POINT('Ctrl Pts',(0.399178429731245,1.09703892879711,-31.6935755172703));
#20690=CARTESIAN_POINT('Ctrl Pts',(0.507266581111613,1.05351244564662,-31.701245116546));
#20691=CARTESIAN_POINT('Ctrl Pts',(0.578724955642715,1.01570900434554,-31.7064229068078));
#20692=CARTESIAN_POINT('Ctrl Pts',(0.679519651351591,0.94862017495968,-31.7145405625731));
#20693=CARTESIAN_POINT('Ctrl Pts',(0.712237917566348,0.92434310659105,-31.7173323014913));
#20694=CARTESIAN_POINT('Ctrl Pts',(0.782828297502978,0.866126524336308,
-31.7237497581707));
#20695=CARTESIAN_POINT('Ctrl Pts',(0.819965848295058,0.831275602275542,
-31.7273928733489));
#20696=CARTESIAN_POINT('Ctrl Pts',(0.889879014567416,0.75648662679121,-31.7346851589437));
#20697=CARTESIAN_POINT('Ctrl Pts',(0.922584047073668,0.716479193628441,
-31.738332751243));
#20698=CARTESIAN_POINT('Ctrl Pts',(0.988121125294871,0.623950581583141,
-31.7460816214656));
#20699=CARTESIAN_POINT('Ctrl Pts',(1.01962351039126,0.570598821904264,-31.7501180542607));
#20700=CARTESIAN_POINT('Ctrl Pts',(1.07676956878579,0.453589499983911,-31.7586015879158));
#20701=CARTESIAN_POINT('Ctrl Pts',(1.10141647309642,0.389406426700824,-31.7630519669856));
#20702=CARTESIAN_POINT('Ctrl Pts',(1.13884447385869,0.259660537621559,-31.7722465089549));
#20703=CARTESIAN_POINT('Ctrl Pts',(1.15194897150424,0.194139742766789,-31.7769860960563));
#20704=CARTESIAN_POINT('Ctrl Pts',(1.1672103135223,0.0594154514047917,-31.786637421575));
#20705=CARTESIAN_POINT('Ctrl Pts',(1.16894378165254,-0.00986571973121408,
-31.7915476746924));
#20706=CARTESIAN_POINT('Ctrl Pts',(1.1604583412024,-0.136354678584791,-31.8001907605822));
#20707=CARTESIAN_POINT('Ctrl Pts',(1.15213820383205,-0.193450951917024,
-31.8039493203448));
#20708=CARTESIAN_POINT('Ctrl Pts',(1.12539423050888,-0.313872074658607,
-31.8119794187064));
#20709=CARTESIAN_POINT('Ctrl Pts',(1.10563389783109,-0.377002239706556,
-31.816262647434));
#20710=CARTESIAN_POINT('Ctrl Pts',(1.06699224135733,-0.472075357193685,
-31.8232522134308));
#20711=CARTESIAN_POINT('Ctrl Pts',(1.05159611665665,-0.505451744236681,
-31.8258065160752));
#20712=CARTESIAN_POINT('Ctrl Pts',(0.997697504751317,-0.609396293443471,
-31.8340351723212));
#20713=CARTESIAN_POINT('Ctrl Pts',(0.953462279858224,-0.677039455355891,
-31.8398087470032));
#20714=CARTESIAN_POINT('Ctrl Pts',(0.875876982117829,-0.772264684904525,
-31.8483668447474));
#20715=CARTESIAN_POINT('Ctrl Pts',(0.847212776712624,-0.803722565967738,
-31.8512769224679));
#20716=CARTESIAN_POINT('Ctrl Pts',(0.787009152503631,-0.86261132692273,
-31.8568875280796));
#20717=CARTESIAN_POINT('Ctrl Pts',(0.755717262167963,-0.890004801972639,
-31.8595912763478));
#20718=CARTESIAN_POINT('Ctrl Pts',(0.678733697678142,-0.950425163636487,
-31.8659695744294));
#20719=CARTESIAN_POINT('Ctrl Pts',(0.63189677977743,-0.981973859333561,
-31.8696567319898));
#20720=CARTESIAN_POINT('Ctrl Pts',(0.519801354509735,-1.04643731668189,
-31.8784459259654));
#20721=CARTESIAN_POINT('Ctrl Pts',(0.453159318095688,-1.07701398350054,
-31.8835937097214));
#20722=CARTESIAN_POINT('Ctrl Pts',(0.30912384004286,-1.12765457696487,-31.8943670714784));
#20723=CARTESIAN_POINT('Ctrl Pts',(0.231242788441453,-1.14650870172707,
-31.8999922894932));
#20724=CARTESIAN_POINT('Ctrl Pts',(0.110773568709514,-1.16249701372248,
-31.9082282615955));
#20725=CARTESIAN_POINT('Ctrl Pts',(0.0692623325449389,-1.1656493189394,
-31.9109710701201));
#20726=CARTESIAN_POINT('Ctrl Pts',(-0.0454268327301759,-1.16809589961942,
-31.9184840634544));
#20727=CARTESIAN_POINT('Ctrl Pts',(-0.118656559476324,-1.16265865935421,
-31.9232749526452));
#20728=CARTESIAN_POINT('Ctrl Pts',(-0.247313507871422,-1.14109367538233,
-31.9321948832158));
#20729=CARTESIAN_POINT('Ctrl Pts',(-0.303190714654443,-1.12752207428608,
-31.9361993591496));
#20730=CARTESIAN_POINT('Ctrl Pts',(-0.452865660521723,-1.07951943878788,
-31.9472141775491));
#20731=CARTESIAN_POINT('Ctrl Pts',(-0.544157689964662,-1.03704794058161,
-31.9542499483904));
#20732=CARTESIAN_POINT('Ctrl Pts',(-0.669499700364756,-0.957123845705213,
-31.9642691289062));
#20733=CARTESIAN_POINT('Ctrl Pts',(-0.708700366708839,-0.928341028069589,
-31.9674498951241));
#20734=CARTESIAN_POINT('Ctrl Pts',(-0.798156607010517,-0.853557790951347,
-31.9751348354495));
#20735=CARTESIAN_POINT('Ctrl Pts',(-0.846532795135961,-0.805251056003578,
-31.9797251625568));
#20736=CARTESIAN_POINT('Ctrl Pts',(-0.950464210935684,-0.681991701886756,
-31.9908063714599));
#20737=CARTESIAN_POINT('Ctrl Pts',(-1.002191263051,-0.603682661018503,-31.997345447302));
#20738=CARTESIAN_POINT('Ctrl Pts',(-1.11304275244878,-0.382944202377441,
-32.0144690651066));
#20739=CARTESIAN_POINT('Ctrl Pts',(-1.15302090381803,-0.2355416839742,-32.0242610185895));
#20740=CARTESIAN_POINT('Ctrl Pts',(-1.17121369822542,0.0302875605874619,
-32.0424073410858));
#20741=CARTESIAN_POINT('Ctrl Pts',(-1.16270608476529,0.144486904507698,
-32.0502868606288));
#20742=CARTESIAN_POINT('Ctrl Pts',(-1.10479117593712,0.406453358131091,
-32.0687819686291));
#20743=CARTESIAN_POINT('Ctrl Pts',(-1.04222804244462,0.547067618273399,
-32.0788474634008));
#20744=CARTESIAN_POINT('Ctrl Pts',(-0.863884158737958,0.797961159360694,
-32.0997864489639));
#20745=CARTESIAN_POINT('Ctrl Pts',(-0.750781838165988,0.905665773067937,
-32.1103406369112));
#20746=CARTESIAN_POINT('Ctrl Pts',(-0.474269706082626,1.08072592818931,
-32.1327633981003));
#20747=CARTESIAN_POINT('Ctrl Pts',(-0.328649337640334,1.12621628952164,
-32.1428790802087));
#20748=CARTESIAN_POINT('Ctrl Pts',(-0.0880045267715734,1.16876081259411,
-32.159463210428));
#20749=CARTESIAN_POINT('Ctrl Pts',(0.0317130996195926,1.17202486743615,
-32.1675214898663));
#20750=CARTESIAN_POINT('Ctrl Pts',(0.207541202474937,1.14986260680352,-32.1797221634427));
#20751=CARTESIAN_POINT('Ctrl Pts',(0.265225746622224,1.13804061104461,-32.1838016068475));
#20752=CARTESIAN_POINT('Ctrl Pts',(0.379471890339568,1.1050092507888,-32.191937678746));
#20753=CARTESIAN_POINT('Ctrl Pts',(0.43549315896196,1.08391949249316,-32.1959752132237));
#20754=CARTESIAN_POINT('Ctrl Pts',(0.489601837133815,1.05872183713728,-32.1999999999999));
#20755=CARTESIAN_POINT('',(-0.881447090972499,1.21320766888878,-30.8075882712147));
#20756=CARTESIAN_POINT('',(-0.6859379234404,0.9441125563889,-30.61554752692));
#20757=CARTESIAN_POINT('Ctrl Pts',(-0.881406518429929,1.21312559025058,
-30.8078849673971));
#20758=CARTESIAN_POINT('Ctrl Pts',(-0.79008662599039,1.27933557882102,-30.8137160152781));
#20759=CARTESIAN_POINT('Ctrl Pts',(-0.691313381309575,1.33525609171038,
-30.8194533024385));
#20760=CARTESIAN_POINT('Ctrl Pts',(-0.489918252130208,1.42100767299626,
-30.8309935829052));
#20761=CARTESIAN_POINT('Ctrl Pts',(-0.388091655782742,1.45203456811973,
-30.8367977370922));
#20762=CARTESIAN_POINT('Ctrl Pts',(-0.172122595797077,1.49390562222026,
-30.8488414701131));
#20763=CARTESIAN_POINT('Ctrl Pts',(-0.0573076259882289,1.502956892091,-30.8550591698905));
#20764=CARTESIAN_POINT('Ctrl Pts',(0.141659514305707,1.49529218732152,-30.8654107218449));
#20765=CARTESIAN_POINT('Ctrl Pts',(0.225375475387054,1.48492949413823,-30.8696854414375));
#20766=CARTESIAN_POINT('Ctrl Pts',(0.461660801982068,1.43520771759958,-30.882150950471));
#20767=CARTESIAN_POINT('Ctrl Pts',(0.609566018273736,1.37841704093802,-30.8906597091753));
#20768=CARTESIAN_POINT('Ctrl Pts',(0.824725152900814,1.2554745072927,-30.9041453796565));
#20769=CARTESIAN_POINT('Ctrl Pts',(0.900182963410078,1.2028217148482,-30.909115708631));
#20770=CARTESIAN_POINT('Ctrl Pts',(1.08476327734415,1.04671912984802,-30.9218791144841));
#20771=CARTESIAN_POINT('Ctrl Pts',(1.18336234755058,0.933435969686118,-30.9293613811484));
#20772=CARTESIAN_POINT('Ctrl Pts',(1.3172285738265,0.722591374806512,-30.9426119478136));
#20773=CARTESIAN_POINT('Ctrl Pts',(1.36220261914603,0.633428070916348,-30.9479777546079));
#20774=CARTESIAN_POINT('Ctrl Pts',(1.4428429516675,0.425550449776397,-30.960018791922));
#20775=CARTESIAN_POINT('Ctrl Pts',(1.4735988539753,0.304792351095012,-30.9666968186304));
#20776=CARTESIAN_POINT('Ctrl Pts',(1.50058334541614,0.0867624271108834,
-30.9782427494017));
#20777=CARTESIAN_POINT('Ctrl Pts',(1.50289470475243,-0.0090133054095964,
-30.9831649796411));
#20778=CARTESIAN_POINT('Ctrl Pts',(1.48179490039278,-0.298466953504106,
-30.9984396551502));
#20779=CARTESIAN_POINT('Ctrl Pts',(1.42987621490152,-0.489656997555912,
-31.0088880132697));
#20780=CARTESIAN_POINT('Ctrl Pts',(1.2386012241916,-0.879835871463111,-31.0321233695193));
#20781=CARTESIAN_POINT('Ctrl Pts',(1.10314579046395,-1.02748310901842,-31.0424184303893));
#20782=CARTESIAN_POINT('Ctrl Pts',(0.841355375644668,-1.25518308736778,
-31.0607060142992));
#20783=CARTESIAN_POINT('Ctrl Pts',(0.671706708060022,-1.35419411522653,
-31.0708950113284));
#20784=CARTESIAN_POINT('Ctrl Pts',(0.399238767357063,-1.44907881193649,
-31.0863851114838));
#20785=CARTESIAN_POINT('Ctrl Pts',(0.306591001400567,-1.47143123103278,
-31.0915269749786));
#20786=CARTESIAN_POINT('Ctrl Pts',(0.113353143272575,-1.49850340174426,
-31.1018748998098));
#20787=CARTESIAN_POINT('Ctrl Pts',(0.0135762553281146,-1.50239730172588,
-31.1070662013325));
#20788=CARTESIAN_POINT('Ctrl Pts',(-0.25279976086019,-1.48689363127454,
-31.1210066620724));
#20789=CARTESIAN_POINT('Ctrl Pts',(-0.440327599977758,-1.4485730974684,
-31.1308870078316));
#20790=CARTESIAN_POINT('Ctrl Pts',(-0.824338933496522,-1.27143949898088,
-31.1539432665113));
#20791=CARTESIAN_POINT('Ctrl Pts',(-0.97390169357174,-1.15076855336848,
-31.1636864658054));
#20792=CARTESIAN_POINT('Ctrl Pts',(-1.14942639738023,-0.96710241579273,
-31.1768629096307));
#20793=CARTESIAN_POINT('Ctrl Pts',(-1.20864987162695,-0.892267291039145,
-31.1818226921469));
#20794=CARTESIAN_POINT('Ctrl Pts',(-1.31153191079653,-0.733178090589835,
-31.1919988181629));
#20795=CARTESIAN_POINT('Ctrl Pts',(-1.35510592769048,-0.649243111987365,
-31.1972110998056));
#20796=CARTESIAN_POINT('Ctrl Pts',(-1.4430303095048,-0.431803877659614,
-31.2099919419473));
#20797=CARTESIAN_POINT('Ctrl Pts',(-1.47664096128969,-0.295262535485362,
-31.2172154468669));
#20798=CARTESIAN_POINT('Ctrl Pts',(-1.50411912757575,-0.0322778863762428,
-31.230824171605));
#20799=CARTESIAN_POINT('Ctrl Pts',(-1.50169331600658,0.0937759591765203,
-31.2373099128508));
#20800=CARTESIAN_POINT('Ctrl Pts',(-1.45877594130903,0.385873451166313,
-31.2533154840002));
#20801=CARTESIAN_POINT('Ctrl Pts',(-1.40192168754619,0.576773620324711,
-31.2641906913579));
#20802=CARTESIAN_POINT('Ctrl Pts',(-1.24228484519573,0.844679607623427,
-31.2802472652015));
#20803=CARTESIAN_POINT('Ctrl Pts',(-1.18883912584601,0.918303367222,-31.284861711137));
#20804=CARTESIAN_POINT('Ctrl Pts',(-1.06362541041061,1.06141058899406,-31.2948277191295));
#20805=CARTESIAN_POINT('Ctrl Pts',(-0.990653681906926,1.12962368854039,
-31.3002226847462));
#20806=CARTESIAN_POINT('Ctrl Pts',(-0.834479275518156,1.24938156325568,
-31.3109555592689));
#20807=CARTESIAN_POINT('Ctrl Pts',(-0.751318553615352,1.30131156952722,
-31.3162982013493));
#20808=CARTESIAN_POINT('Ctrl Pts',(-0.552552652402147,1.39983681676189,
-31.3281230810791));
#20809=CARTESIAN_POINT('Ctrl Pts',(-0.435630188981496,1.44041399534726,
-31.3343404047184));
#20810=CARTESIAN_POINT('Ctrl Pts',(-0.132937870119536,1.50496257801301,
-31.3504040525313));
#20811=CARTESIAN_POINT('Ctrl Pts',(0.0559719993075142,1.50928152959898,
-31.3605875743258));
#20812=CARTESIAN_POINT('Ctrl Pts',(0.416632678179987,1.45186566078964,-31.3802907470301));
#20813=CARTESIAN_POINT('Ctrl Pts',(0.586857963378165,1.39229352268651,-31.3893980346239));
#20814=CARTESIAN_POINT('Ctrl Pts',(0.910640740006506,1.20620019271066,-31.4090381303016));
#20815=CARTESIAN_POINT('Ctrl Pts',(1.05917804790911,1.07788949844651,-31.41946583828));
#20816=CARTESIAN_POINT('Ctrl Pts',(1.32423117837389,0.742889010787418,-31.4423282514141));
#20817=CARTESIAN_POINT('Ctrl Pts',(1.40073910986579,0.558632045022755,-31.452494098352));
#20818=CARTESIAN_POINT('Ctrl Pts',(1.49626125117303,0.215384419002758,-31.4713146187414));
#20819=CARTESIAN_POINT('Ctrl Pts',(1.51221196691776,0.014491680411974,-31.4818312421332));
#20820=CARTESIAN_POINT('Ctrl Pts',(1.47740899534278,-0.276788453865656,
-31.4975402963852));
#20821=CARTESIAN_POINT('Ctrl Pts',(1.45682220235215,-0.369786974767944,
-31.5026323980835));
#20822=CARTESIAN_POINT('Ctrl Pts',(1.36806601562231,-0.642230151416177,
-31.517791599168));
#20823=CARTESIAN_POINT('Ctrl Pts',(1.27387636212263,-0.812521573844567,
-31.5277066552976));
#20824=CARTESIAN_POINT('Ctrl Pts',(1.02814167442595,-1.10901835949839,-31.548154594587));
#20825=CARTESIAN_POINT('Ctrl Pts',(0.878131014092237,-1.23143645550272,
-31.5586713008323));
#20826=CARTESIAN_POINT('Ctrl Pts',(0.542797830598519,-1.40952383585759,
-31.578579337433));
#20827=CARTESIAN_POINT('Ctrl Pts',(0.363013394480282,-1.46628866348356,
-31.5880421456073));
#20828=CARTESIAN_POINT('Ctrl Pts',(0.0743620682596745,-1.50154155002754,
-31.6036596732713));
#20829=CARTESIAN_POINT('Ctrl Pts',(-0.0311382941941019,-1.50311766402509,
-31.6094853829751));
#20830=CARTESIAN_POINT('Ctrl Pts',(-0.246326110710298,-1.48346206537663,
-31.6211736713795));
#20831=CARTESIAN_POINT('Ctrl Pts',(-0.355213869364278,-1.46090073589857,
-31.6269166443787));
#20832=CARTESIAN_POINT('Ctrl Pts',(-0.53321731237527,-1.40330380008982,
-31.6365687084528));
#20833=CARTESIAN_POINT('Ctrl Pts',(-0.604429361722516,-1.37413765579584,
-31.6405141016791));
#20834=CARTESIAN_POINT('Ctrl Pts',(-0.79410328740295,-1.27901266898536,
-31.6516104404927));
#20835=CARTESIAN_POINT('Ctrl Pts',(-0.905494966010469,-1.20273423832872,
-31.6589593501426));
#20836=CARTESIAN_POINT('Ctrl Pts',(-1.166901453977,-0.966788599054434,-31.678226063038));
#20837=CARTESIAN_POINT('Ctrl Pts',(-1.2772148206795,-0.803691622859537,
-31.6880116044744));
#20838=CARTESIAN_POINT('Ctrl Pts',(-1.3849448199296,-0.579839538881978,
-31.7008813038447));
#20839=CARTESIAN_POINT('Ctrl Pts',(-1.41329287853837,-0.506704748463012,
-31.7050201908034));
#20840=CARTESIAN_POINT('Ctrl Pts',(-1.47287881374097,-0.308138417722713,
-31.7162293998432));
#20841=CARTESIAN_POINT('Ctrl Pts',(-1.49412227426975,-0.179965409458075,
-31.7233765017813));
#20842=CARTESIAN_POINT('Ctrl Pts',(-1.50233949805111,0.0512896747237151,
-31.7357797099441));
#20843=CARTESIAN_POINT('Ctrl Pts',(-1.49536294654877,0.153084621763814,
-31.7410012173628));
#20844=CARTESIAN_POINT('Ctrl Pts',(-1.46151200506474,0.349489472780055,
-31.7512417022782));
#20845=CARTESIAN_POINT('Ctrl Pts',(-1.43574274826947,0.443079292656519,
-31.7562649972009));
#20846=CARTESIAN_POINT('Ctrl Pts',(-1.35324376147598,0.65860320719556,-31.7686134586091));
#20847=CARTESIAN_POINT('Ctrl Pts',(-1.28894921214917,0.77707047456878,-31.7759524714491));
#20848=CARTESIAN_POINT('Ctrl Pts',(-1.09859692931211,1.03858451421536,-31.7933795730877));
#20849=CARTESIAN_POINT('Ctrl Pts',(-0.960074498189745,1.16789073189457,
-31.8027834654643));
#20850=CARTESIAN_POINT('Ctrl Pts',(-0.656121551014658,1.35824435926684,
-31.8217597197663));
#20851=CARTESIAN_POINT('Ctrl Pts',(-0.498064699137248,1.42381470626568,
-31.8309331232312));
#20852=CARTESIAN_POINT('Ctrl Pts',(-0.14094115511042,1.50641662107625,-31.8505768131683));
#20853=CARTESIAN_POINT('Ctrl Pts',(0.0557338468603843,1.51165229967551,
-31.8605541249687));
#20854=CARTESIAN_POINT('Ctrl Pts',(0.444388507881338,1.4448535910386,-31.8814228607825));
#20855=CARTESIAN_POINT('Ctrl Pts',(0.632485824724102,1.37356746613444,-31.8919926370937));
#20856=CARTESIAN_POINT('Ctrl Pts',(0.98895705395808,1.15025371807177,-31.9144543658979));
#20857=CARTESIAN_POINT('Ctrl Pts',(1.1221288035876,1.00707400476522,-31.924529693045));
#20858=CARTESIAN_POINT('Ctrl Pts',(1.27392369897089,0.796101204632409,-31.9382013838022));
#20859=CARTESIAN_POINT('Ctrl Pts',(1.32421243107241,0.709581560557193,-31.9434492774636));
#20860=CARTESIAN_POINT('Ctrl Pts',(1.4466469402899,0.441345485206039,-31.959132347925));
#20861=CARTESIAN_POINT('Ctrl Pts',(1.49142361622571,0.252182015772013,-31.9695969023453));
#20862=CARTESIAN_POINT('Ctrl Pts',(1.5050330411194,-0.131895182047114,-31.9897595738826));
#20863=CARTESIAN_POINT('Ctrl Pts',(1.47628922826956,-0.322084931689001,
-31.9994735551462));
#20864=CARTESIAN_POINT('Ctrl Pts',(1.38141864067906,-0.5919315821454,-32.0148547383256));
#20865=CARTESIAN_POINT('Ctrl Pts',(1.34040367527535,-0.679847013725666,
-32.0201949304321));
#20866=CARTESIAN_POINT('Ctrl Pts',(1.23541296291457,-0.857179707721256,
-32.031322308911));
#20867=CARTESIAN_POINT('Ctrl Pts',(1.16939049170082,-0.944710215970665,
-32.0369916517565));
#20868=CARTESIAN_POINT('Ctrl Pts',(0.995624032465529,-1.13005097410711,
-32.0501197742209));
#20869=CARTESIAN_POINT('Ctrl Pts',(0.863278653887601,-1.24099037191773,
-32.0588622674964));
#20870=CARTESIAN_POINT('Ctrl Pts',(0.591571910837053,-1.38260099293634,
-32.0756184397751));
#20871=CARTESIAN_POINT('Ctrl Pts',(0.484976021203013,-1.42366132742166,
-32.081906458484));
#20872=CARTESIAN_POINT('Ctrl Pts',(0.252444912482356,-1.48352548355856,
-32.0946122106501));
#20873=CARTESIAN_POINT('Ctrl Pts',(0.126228242511555,-1.49940828336764,
-32.1010172840953));
#20874=CARTESIAN_POINT('Ctrl Pts',(1.77217646831623E-6,-1.49940943975982,
-32.1075644477068));
#20875=CARTESIAN_POINT('Ctrl Pts',(-1.354384777031,0.7225666776598,-30.25156091023));
#20876=CARTESIAN_POINT('Ctrl Pts',(-1.177323984063,1.054450848381,-30.27106091023));
#20877=CARTESIAN_POINT('Ctrl Pts',(-0.569111203504,1.580105774587,-30.31006091023));
#20878=CARTESIAN_POINT('Ctrl Pts',(0.6379428881994,1.553898857047,-30.36856091023));
#20879=CARTESIAN_POINT('Ctrl Pts',(1.515280082606,0.7246860501608,-30.42706091023));
#20880=CARTESIAN_POINT('Ctrl Pts',(1.610006155319,-0.4787341075376,-30.48556091023));
#20881=CARTESIAN_POINT('Ctrl Pts',(0.8731225586908,-1.434908334168,-30.54406091023));
#20882=CARTESIAN_POINT('Ctrl Pts',(-0.3147391875509,-1.649921262663,-30.60256091023));
#20883=CARTESIAN_POINT('Ctrl Pts',(-1.340034041364,-1.012724728735,-30.66106091023));
#20884=CARTESIAN_POINT('Ctrl Pts',(-1.673178974659,0.1475613323174,-30.71956091023));
#20885=CARTESIAN_POINT('Ctrl Pts',(-1.142099513493,1.231629392261,-30.77806091023));
#20886=CARTESIAN_POINT('Ctrl Pts',(-0.0211068401903,1.679540644058,-30.83656091023));
#20887=CARTESIAN_POINT('Ctrl Pts',(1.110787857823,1.259941506756,-30.89506091023));
#20888=CARTESIAN_POINT('Ctrl Pts',(1.668942351274,0.1895618522656,-30.95356091023));
#20889=CARTESIAN_POINT('Ctrl Pts',(1.365060658244,-0.9787296188165,-31.01206091023));
#20890=CARTESIAN_POINT('Ctrl Pts',(0.3561026739166,-1.641491137051,-31.07056091023));
#20891=CARTESIAN_POINT('Ctrl Pts',(-0.8367882010172,-1.456395473099,-31.12906091023));
#20892=CARTESIAN_POINT('Ctrl Pts',(-1.597464201167,-0.519047582986,-31.18756091023));
#20893=CARTESIAN_POINT('Ctrl Pts',(-1.533023655909,0.686396924418,-31.24606091023));
#20894=CARTESIAN_POINT('Ctrl Pts',(-0.6767511671866,1.53730612602,-31.30456091023));
#20895=CARTESIAN_POINT('Ctrl Pts',(0.52907443495,1.594171417921,-31.36306091023));
#20896=CARTESIAN_POINT('Ctrl Pts',(1.461624385972,0.8276209410372,-31.42156091023));
#20897=CARTESIAN_POINT('Ctrl Pts',(1.639221290546,-0.3664093696299,-31.48006091023));
#20898=CARTESIAN_POINT('Ctrl Pts',(0.9701334287918,-1.371183213173,-31.53856091023));
#20899=CARTESIAN_POINT('Ctrl Pts',(-0.2000443226221,-1.667718359793,-31.59706091023));
#20900=CARTESIAN_POINT('Ctrl Pts',(-1.266895850185,-1.102849551308,-31.65556091023));
#20901=CARTESIAN_POINT('Ctrl Pts',(-1.679374972687,0.03165926908636,-31.71406091023));
#20902=CARTESIAN_POINT('Ctrl Pts',(-1.224428737161,1.149815288114,-31.77256091023));
#20903=CARTESIAN_POINT('Ctrl Pts',(-0.1370469690625,1.674073791154,-31.83106091023));
#20904=CARTESIAN_POINT('Ctrl Pts',(1.021129492522,1.333641902982,-31.88956091023));
#20905=CARTESIAN_POINT('Ctrl Pts',(1.651847110893,0.3043759554816,-31.94806091023));
#20906=CARTESIAN_POINT('Ctrl Pts',(1.42946546972,-0.8821571614021,-32.00656091023));
#20907=CARTESIAN_POINT('Ctrl Pts',(0.4683422360403,-1.612847596885,-32.06506091023));
#20908=CARTESIAN_POINT('Ctrl Pts',(-0.3326844530463,-1.545082331076,-32.10406091023));
#20909=CARTESIAN_POINT('Ctrl Pts',(-0.6710062646147,-1.380656119664,-32.12356091023));
#20910=CARTESIAN_POINT('Ctrl Pts',(-1.235814757055,0.6593093619714,-30.32915029444));
#20911=CARTESIAN_POINT('Ctrl Pts',(-1.07425480411,0.9621386338044,-30.34865029444));
#20912=CARTESIAN_POINT('Ctrl Pts',(-0.5192881931508,1.441774942437,-30.38765029444));
#20913=CARTESIAN_POINT('Ctrl Pts',(0.5820939874436,1.417862317323,-30.44615029444));
#20914=CARTESIAN_POINT('Ctrl Pts',(1.38262443503,0.6612431933735,-30.50465029444));
#20915=CARTESIAN_POINT('Ctrl Pts',(1.469057685405,-0.4368231870542,-30.56315029444));
#20916=CARTESIAN_POINT('Ctrl Pts',(0.7966847834135,-1.309288855323,-30.62165029444));
#20917=CARTESIAN_POINT('Ctrl Pts',(-0.2871852513371,-1.50547841275,-30.68015029444));
#20918=CARTESIAN_POINT('Ctrl Pts',(-1.22272036083,-0.9240654397699,-30.73865029444));
#20919=CARTESIAN_POINT('Ctrl Pts',(-1.5267000214,0.1346430313904,-30.79715029444));
#20920=CARTESIAN_POINT('Ctrl Pts',(-1.042114070341,1.123806029122,-30.85565029444));
#20921=CARTESIAN_POINT('Ctrl Pts',(-0.01925903555941,1.532504756551,-30.91415029444));
#20922=CARTESIAN_POINT('Ctrl Pts',(1.013543602922,1.149639551094,-30.97265029444));
#20923=CARTESIAN_POINT('Ctrl Pts',(1.522834294475,0.1729666032706,-31.03115029444));
#20924=CARTESIAN_POINT('Ctrl Pts',(1.245556015057,-0.8930464419066,-31.08965029444));
#20925=CARTESIAN_POINT('Ctrl Pts',(0.3249275589301,-1.497786305004,-31.14815029444));
#20926=CARTESIAN_POINT('Ctrl Pts',(-0.7635313279386,-1.328894896257,-31.20665029444));
#20927=CARTESIAN_POINT('Ctrl Pts',(-1.457613720376,-0.4736074072494,-31.26515029444));
#20928=CARTESIAN_POINT('Ctrl Pts',(-1.398814641906,0.6263061005841,-31.32365029444));
#20929=CARTESIAN_POINT('Ctrl Pts',(-0.6175047840515,1.402722201892,-31.38215029444));
#20930=CARTESIAN_POINT('Ctrl Pts',(0.4827564554623,1.454609204823,-31.44065029444));
#20931=CARTESIAN_POINT('Ctrl Pts',(1.333666042389,0.7551666184726,-31.49915029444));
#20932=CARTESIAN_POINT('Ctrl Pts',(1.495715172889,-0.3343319518877,-31.55765029444));
#20933=CARTESIAN_POINT('Ctrl Pts',(0.8852028079061,-1.251142569086,-31.61615029444));
#20934=CARTESIAN_POINT('Ctrl Pts',(-0.1825313826277,-1.521717457694,-31.67465029444));
#20935=CARTESIAN_POINT('Ctrl Pts',(-1.15598507445,-1.006300257822,-31.73315029444));
#20936=CARTESIAN_POINT('Ctrl Pts',(-1.53235358893,0.02888764891485,-31.79165029444));
#20937=CARTESIAN_POINT('Ctrl Pts',(-1.117235757524,1.049154365167,-31.85015029444));
#20938=CARTESIAN_POINT('Ctrl Pts',(-0.1250491512082,1.527516500918,-31.90865029444));
#20939=CARTESIAN_POINT('Ctrl Pts',(0.9317344059998,1.216887824112,-31.96715029444));
#20940=CARTESIAN_POINT('Ctrl Pts',(1.507235662021,0.2777292715157,-32.02565029444));
#20941=CARTESIAN_POINT('Ctrl Pts',(1.304322488069,-0.804928449131,-32.08415029444));
#20942=CARTESIAN_POINT('Ctrl Pts',(0.4273410750521,-1.471650372119,-32.14265029444));
#20943=CARTESIAN_POINT('Ctrl Pts',(-0.303559493203,-1.409817636753,-32.18165029444));
#20944=CARTESIAN_POINT('Ctrl Pts',(-0.6122628206918,-1.259786167148,-32.20115029444));
#20945=CARTESIAN_POINT('Ctrl Pts',(-1.117244737079,0.5960520462829,-30.40673967864));
#20946=CARTESIAN_POINT('Ctrl Pts',(-0.9711856241576,0.8698264192279,-30.42623967864));
#20947=CARTESIAN_POINT('Ctrl Pts',(-0.4694651827977,1.303444110288,-30.46523967864));
#20948=CARTESIAN_POINT('Ctrl Pts',(0.5262450866879,1.2818257776,-30.52373967864));
#20949=CARTESIAN_POINT('Ctrl Pts',(1.249968787454,0.5978003365862,-30.58223967864));
#20950=CARTESIAN_POINT('Ctrl Pts',(1.32810921549,-0.3949122665708,-30.64073967864));
#20951=CARTESIAN_POINT('Ctrl Pts',(0.7202470081362,-1.183669376478,-30.69923967864));
#20952=CARTESIAN_POINT('Ctrl Pts',(-0.2596313151233,-1.361035562837,-30.75773967864));
#20953=CARTESIAN_POINT('Ctrl Pts',(-1.105406680295,-0.8354061508049,-30.81623967864));
#20954=CARTESIAN_POINT('Ctrl Pts',(-1.380221068141,0.1217247304635,-30.87473967864));
#20955=CARTESIAN_POINT('Ctrl Pts',(-0.9421286271891,1.015982665983,-30.93323967864));
#20956=CARTESIAN_POINT('Ctrl Pts',(-0.01741123092852,1.385468869044,-30.99173967864));
#20957=CARTESIAN_POINT('Ctrl Pts',(0.9162993480212,1.039337595432,-31.05023967864));
#20958=CARTESIAN_POINT('Ctrl Pts',(1.376726237677,0.1563713542756,-31.10873967864));
#20959=CARTESIAN_POINT('Ctrl Pts',(1.12605137187,-0.8073632649967,-31.16723967864));
#20960=CARTESIAN_POINT('Ctrl Pts',(0.2937524439436,-1.354081472956,-31.22573967864));
#20961=CARTESIAN_POINT('Ctrl Pts',(-0.6902744548601,-1.201394319414,-31.28423967864));
#20962=CARTESIAN_POINT('Ctrl Pts',(-1.317763239585,-0.4281672315128,-31.34273967864));
#20963=CARTESIAN_POINT('Ctrl Pts',(-1.264605627904,0.5662152767502,-31.40123967864));
#20964=CARTESIAN_POINT('Ctrl Pts',(-0.5582584009165,1.268138277765,-31.45973967864));
#20965=CARTESIAN_POINT('Ctrl Pts',(0.4364384759746,1.315046991725,-31.51823967864));
#20966=CARTESIAN_POINT('Ctrl Pts',(1.205707698806,0.682712295908,-31.57673967864));
#20967=CARTESIAN_POINT('Ctrl Pts',(1.352209055232,-0.3022545341455,-31.63523967864));
#20968=CARTESIAN_POINT('Ctrl Pts',(0.8002721870203,-1.131101924998,-31.69373967864));
#20969=CARTESIAN_POINT('Ctrl Pts',(-0.1650184426333,-1.375716555595,-31.75223967864));
#20970=CARTESIAN_POINT('Ctrl Pts',(-1.045074298715,-0.9097509643373,-31.81073967864));
#20971=CARTESIAN_POINT('Ctrl Pts',(-1.385332205172,0.02611602874334,-31.86923967864));
#20972=CARTESIAN_POINT('Ctrl Pts',(-1.010042777888,0.9484934422207,-31.92773967864));
#20973=CARTESIAN_POINT('Ctrl Pts',(-0.1130513333539,1.380959210682,-31.98623967864));
#20974=CARTESIAN_POINT('Ctrl Pts',(0.8423393194779,1.100133745242,-32.04473967864));
#20975=CARTESIAN_POINT('Ctrl Pts',(1.362624213149,0.2510825875499,-32.10323967864));
#20976=CARTESIAN_POINT('Ctrl Pts',(1.179179506419,-0.72769973686,-32.16173967864));
#20977=CARTESIAN_POINT('Ctrl Pts',(0.3863399140639,-1.330453147354,-32.22023967864));
#20978=CARTESIAN_POINT('Ctrl Pts',(-0.2744345333596,-1.27455294243,-32.25923967864));
#20979=CARTESIAN_POINT('Ctrl Pts',(-0.5535193767689,-1.138916214631,-32.27873967864));
#20980=CARTESIAN_POINT('Ctrl Pts',(-0.9986747171026,0.5327947305945,-30.48432906285));
#20981=CARTESIAN_POINT('Ctrl Pts',(-0.868116444205,0.7775142046513,-30.50382906285));
#20982=CARTESIAN_POINT('Ctrl Pts',(-0.4196421724445,1.165113278138,-30.54282906285));
#20983=CARTESIAN_POINT('Ctrl Pts',(0.4703961859321,1.145789237877,-30.60132906285));
#20984=CARTESIAN_POINT('Ctrl Pts',(1.117313139878,0.5343574797989,-30.65982906285));
#20985=CARTESIAN_POINT('Ctrl Pts',(1.187160745576,-0.3530013460875,-30.71832906285));
#20986=CARTESIAN_POINT('Ctrl Pts',(0.6438092328589,-1.058049897633,-30.77682906285));
#20987=CARTESIAN_POINT('Ctrl Pts',(-0.2320773789096,-1.216592712924,-30.83532906285));
#20988=CARTESIAN_POINT('Ctrl Pts',(-0.9880929997609,-0.74674686184,-30.89382906285));
#20989=CARTESIAN_POINT('Ctrl Pts',(-1.233742114882,0.1088064295365,-30.95232906285));
#20990=CARTESIAN_POINT('Ctrl Pts',(-0.8421431840371,0.9081593028442,-31.01082906285));
#20991=CARTESIAN_POINT('Ctrl Pts',(-0.01556342629764,1.238432981537,-31.06932906285));
#20992=CARTESIAN_POINT('Ctrl Pts',(0.8190550931203,0.9290356397707,-31.12782906285));
#20993=CARTESIAN_POINT('Ctrl Pts',(1.230618180878,0.1397761052806,-31.18632906285));
#20994=CARTESIAN_POINT('Ctrl Pts',(1.006546728684,-0.7216800880868,-31.24482906285));
#20995=CARTESIAN_POINT('Ctrl Pts',(0.2625773289571,-1.210376640909,-31.30332906285));
#20996=CARTESIAN_POINT('Ctrl Pts',(-0.6170175817815,-1.073893742571,-31.36182906285));
#20997=CARTESIAN_POINT('Ctrl Pts',(-1.177912758794,-0.3827270557762,-31.42032906285));
#20998=CARTESIAN_POINT('Ctrl Pts',(-1.130396613902,0.5061244529163,-31.47882906285));
#20999=CARTESIAN_POINT('Ctrl Pts',(-0.4990120177814,1.133554353637,-31.53732906285));
#21000=CARTESIAN_POINT('Ctrl Pts',(0.390120496487,1.175484778628,-31.59582906285));
#21001=CARTESIAN_POINT('Ctrl Pts',(1.077749355224,0.6102579733435,-31.65432906285));
#21002=CARTESIAN_POINT('Ctrl Pts',(1.208702937575,-0.2701771164033,-31.71282906285));
#21003=CARTESIAN_POINT('Ctrl Pts',(0.7153415661346,-1.011061280911,-31.77132906285));
#21004=CARTESIAN_POINT('Ctrl Pts',(-0.147505502639,-1.229715653496,-31.82982906285));
#21005=CARTESIAN_POINT('Ctrl Pts',(-0.9341635229797,-0.8132016708522,-31.88832906285));
#21006=CARTESIAN_POINT('Ctrl Pts',(-1.238310821415,0.02334440857183,-31.94682906285));
#21007=CARTESIAN_POINT('Ctrl Pts',(-0.9028497982508,0.8478325192742,-32.00532906285));
#21008=CARTESIAN_POINT('Ctrl Pts',(-0.1010535154996,1.234401920446,-32.06382906285));
#21009=CARTESIAN_POINT('Ctrl Pts',(0.752944232956,0.9833796663719,-32.12232906285));
#21010=CARTESIAN_POINT('Ctrl Pts',(1.218012764277,0.224435903584,-32.18082906285));
#21011=CARTESIAN_POINT('Ctrl Pts',(1.054036524768,-0.6504710245889,-32.23932906285));
#21012=CARTESIAN_POINT('Ctrl Pts',(0.3453387530757,-1.189255922589,-32.29782906285));
#21013=CARTESIAN_POINT('Ctrl Pts',(-0.2453095735162,-1.139288248107,-32.33682906285));
#21014=CARTESIAN_POINT('Ctrl Pts',(-0.494775932846,-1.018046262115,-32.35632906285));
#21015=CARTESIAN_POINT('Ctrl Pts',(1.58448099658799E-15,-1.4996457514538,
-32.1074280088343));
#21016=CARTESIAN_POINT('Ctrl Pts',(-4.02777456180757E-14,-1.47307126155369,
-32.1227816138083));
#21017=CARTESIAN_POINT('Ctrl Pts',(-4.08797690373025E-12,-1.44649677165354,
-32.1381352187823));
#21018=CARTESIAN_POINT('Ctrl Pts',(-4.08797690373025E-12,-1.39314602998405,
-32.1689589981181));
#21019=CARTESIAN_POINT('Ctrl Pts',(-6.03115543055E-16,-1.36636977821469,
-32.1844291724799));
#21020=CARTESIAN_POINT('Ctrl Pts',(-6.03115543055E-16,-1.33959352644542,
-32.1998993468418));
#21021=CARTESIAN_POINT('',(-0.881417612943866,1.21316727086597,-30.3080680843044));
#21022=CARTESIAN_POINT('Ctrl Pts',(-0.881271937662713,1.21292436187718,
-30.8080241838854));
#21023=CARTESIAN_POINT('Ctrl Pts',(-1.00850257770077,1.12100015634677,-30.7997573214021));
#21024=CARTESIAN_POINT('Ctrl Pts',(-1.11962151110689,1.01045334070276,-30.791142048369));
#21025=CARTESIAN_POINT('Ctrl Pts',(-1.29782368007299,0.764709539444589,
-30.7748536411824));
#21026=CARTESIAN_POINT('Ctrl Pts',(-1.36620783948847,0.633308215427597,
-30.7672924655404));
#21027=CARTESIAN_POINT('Ctrl Pts',(-1.44791553044954,0.400408010499091,
-30.7544822326199));
#21028=CARTESIAN_POINT('Ctrl Pts',(-1.47183072254183,0.302461831188457,
-30.7492472683227));
#21029=CARTESIAN_POINT('Ctrl Pts',(-1.49870865055451,0.109629087763779,
-30.738824650982));
#21030=CARTESIAN_POINT('Ctrl Pts',(-1.50269192751912,0.0158391051916832,
-30.7336538650198));
#21031=CARTESIAN_POINT('Ctrl Pts',(-1.48844953100768,-0.251855598929125,
-30.7190433780395));
#21032=CARTESIAN_POINT('Ctrl Pts',(-1.44806891166574,-0.423480947216793,
-30.7100681728756));
#21033=CARTESIAN_POINT('Ctrl Pts',(-1.34175315864756,-0.675773645942979,
-30.6958599534907));
#21034=CARTESIAN_POINT('Ctrl Pts',(-1.29359321344248,-0.764564369839684,
-30.690618628421));
#21035=CARTESIAN_POINT('Ctrl Pts',(-1.18513459159227,-0.923705254367759,
-30.6803156958803));
#21036=CARTESIAN_POINT('Ctrl Pts',(-1.12669270096378,-0.994231687201124,
-30.6752783061748));
#21037=CARTESIAN_POINT('Ctrl Pts',(-0.938545859850394,-1.18244444707684,
-30.6607782140534));
#21038=CARTESIAN_POINT('Ctrl Pts',(-0.793522725874811,-1.2832066969144,
-30.6517845335157));
#21039=CARTESIAN_POINT('Ctrl Pts',(-0.545053607980234,-1.39997528592721,
-30.6375367089199));
#21040=CARTESIAN_POINT('Ctrl Pts',(-0.449356628346627,-1.43389985036606,
-30.6322690691834));
#21041=CARTESIAN_POINT('Ctrl Pts',(-0.256824866392193,-1.48080608022622,
-30.6216685621478));
#21042=CARTESIAN_POINT('Ctrl Pts',(-0.161142963600495,-1.4942981699223,
-30.6163461134762));
#21043=CARTESIAN_POINT('Ctrl Pts',(0.0965437044720375,-1.50505707981076,
-30.6023150548004));
#21044=CARTESIAN_POINT('Ctrl Pts',(0.258322541556046,-1.48506645149598,
-30.593976335957));
#21045=CARTESIAN_POINT('Ctrl Pts',(0.513375728501787,-1.41211330395416,
-30.5802170579591));
#21046=CARTESIAN_POINT('Ctrl Pts',(0.611090204635858,-1.37300329719874,
-30.5747725770304));
#21047=CARTESIAN_POINT('Ctrl Pts',(0.795293760309478,-1.27574114267746,
-30.5636573804259));
#21048=CARTESIAN_POINT('Ctrl Pts',(0.880864790932003,-1.21831318979652,
-30.5579831919676));
#21049=CARTESIAN_POINT('Ctrl Pts',(1.05086496760408,-1.07627017131234,-30.5459381412953));
#21050=CARTESIAN_POINT('Ctrl Pts',(1.13229476874188,-0.989462653585845,
-30.5397306838153));
#21051=CARTESIAN_POINT('Ctrl Pts',(1.31267063557654,-0.746322614434621,
-30.52399325693));
#21052=CARTESIAN_POINT('Ctrl Pts',(1.39617883260761,-0.577543248151898,
-30.5144741851185));
#21053=CARTESIAN_POINT('Ctrl Pts',(1.47191857527949,-0.304326950315721,
-30.4990435204291));
#21054=CARTESIAN_POINT('Ctrl Pts',(1.48855505534371,-0.207802407227979,
-30.4936519971964));
#21055=CARTESIAN_POINT('Ctrl Pts',(1.50286798890886,-0.00518476754475829,
-30.4827983456252));
#21056=CARTESIAN_POINT('Ctrl Pts',(1.49922046596233,0.0999638418623623,
-30.4773509267098));
#21057=CARTESIAN_POINT('Ctrl Pts',(1.46369104273209,0.358095280148811,-30.4638339471291));
#21058=CARTESIAN_POINT('Ctrl Pts',(1.41636832436588,0.528094531696217,-30.4548661060413));
#21059=CARTESIAN_POINT('Ctrl Pts',(1.28560465947371,0.777895524399192,-30.4394761899898));
#21060=CARTESIAN_POINT('Ctrl Pts',(1.23584650838838,0.854597008610237,-30.4344616337474));
#21061=CARTESIAN_POINT('Ctrl Pts',(1.11320543282276,1.00976823521111,-30.4239068184296));
#21062=CARTESIAN_POINT('Ctrl Pts',(1.03870092469521,1.08581595462586,-30.4184021257723));
#21063=CARTESIAN_POINT('Ctrl Pts',(0.833653311054535,1.25586254468988,-30.4045866429208));
#21064=CARTESIAN_POINT('Ctrl Pts',(0.69364232957928,1.33917766672989,-30.3962483611893));
#21065=CARTESIAN_POINT('Ctrl Pts',(0.452710415206934,1.4332053036504,-30.3821661482874));
#21066=CARTESIAN_POINT('Ctrl Pts',(0.358915569212309,1.45945723586656,-30.3767980732763));
#21067=CARTESIAN_POINT('Ctrl Pts',(0.160658085760966,1.4941602769485,-30.3660297074887));
#21068=CARTESIAN_POINT('Ctrl Pts',(0.057009913787783,1.50135840423208,-30.3606431606162));
#21069=CARTESIAN_POINT('Ctrl Pts',(-0.19053515909408,1.49356059421536,-30.3477934729808));
#21070=CARTESIAN_POINT('Ctrl Pts',(-0.334268697842853,1.46862044317557,
-30.3403361053898));
#21071=CARTESIAN_POINT('Ctrl Pts',(-0.618615280175414,1.37522068205069,
-30.3242597935662));
#21072=CARTESIAN_POINT('Ctrl Pts',(-0.756125381298191,1.30435623160632,
-30.3157610121053));
#21073=CARTESIAN_POINT('Ctrl Pts',(-0.8812312603029,1.21295391713908,-30.3076008391023));
#21074=CARTESIAN_POINT('',(-0.685937814923959,0.944112407119636,-30.5000774675642));
#21075=CARTESIAN_POINT('',(-0.8816778784387,1.213525491562,-30.3078125));
#21076=CARTESIAN_POINT('Ctrl Pts',(-0.685548708199919,0.943590117361044,
-30.4999580574627));
#21077=CARTESIAN_POINT('Ctrl Pts',(-0.620658503056946,0.990901745737687,
-30.5054493275448));
#21078=CARTESIAN_POINT('Ctrl Pts',(-0.550959823264162,1.03163702953013,
-30.5109566740961));
#21079=CARTESIAN_POINT('Ctrl Pts',(-0.403872488361834,1.09795612075019,
-30.5220381978001));
#21080=CARTESIAN_POINT('Ctrl Pts',(-0.327257154251574,1.12290648436756,
-30.5275399734823));
#21081=CARTESIAN_POINT('Ctrl Pts',(-0.100873402982573,1.17156187918893,
-30.5432675541518));
#21082=CARTESIAN_POINT('Ctrl Pts',(0.053399591797408,1.17465261587528,-30.553424700155));
#21083=CARTESIAN_POINT('Ctrl Pts',(0.391521872713888,1.11617340314988,-30.5768753375799));
#21084=CARTESIAN_POINT('Ctrl Pts',(0.53180965214093,1.04428570792321,-30.5876876224664));
#21085=CARTESIAN_POINT('Ctrl Pts',(0.72553131493444,0.920594607136468,-30.6032043458073));
#21086=CARTESIAN_POINT('Ctrl Pts',(0.816159816510971,0.841517554690681,
-30.611101164653));
#21087=CARTESIAN_POINT('Ctrl Pts',(0.960946221710973,0.670376878708893,
-30.6263353830646));
#21088=CARTESIAN_POINT('Ctrl Pts',(1.01723879274502,0.581765626143624,-30.6337115693417));
#21089=CARTESIAN_POINT('Ctrl Pts',(1.10425141536702,0.390087082012562,-30.64834528083));
#21090=CARTESIAN_POINT('Ctrl Pts',(1.13460050240139,0.288910726357807,-30.6553271203898));
#21091=CARTESIAN_POINT('Ctrl Pts',(1.16338805497993,0.111296031839137,-30.6672934493909));
#21092=CARTESIAN_POINT('Ctrl Pts',(1.16840076223968,0.0358059784192352,
-30.6722986874147));
#21093=CARTESIAN_POINT('Ctrl Pts',(1.1640118352481,-0.106156990343197,-30.6819567814185));
#21094=CARTESIAN_POINT('Ctrl Pts',(1.15618689001219,-0.172475808382573,
-30.686599600179));
#21095=CARTESIAN_POINT('Ctrl Pts',(1.1324952743554,-0.285021426899435,-30.6947702271497));
#21096=CARTESIAN_POINT('Ctrl Pts',(1.11969541457319,-0.331193090783143,
-30.6981669611072));
#21097=CARTESIAN_POINT('Ctrl Pts',(1.06524415949267,-0.489387920864526,
-30.7097201100341));
#21098=CARTESIAN_POINT('Ctrl Pts',(1.00906889671204,-0.596548724884538,
-30.7175157393668));
#21099=CARTESIAN_POINT('Ctrl Pts',(0.907478030436901,-0.734901646249509,
-30.7288918619303));
#21100=CARTESIAN_POINT('Ctrl Pts',(0.873819215807472,-0.774897823605277,
-30.7323768988926));
#21101=CARTESIAN_POINT('Ctrl Pts',(0.804048748951575,-0.847167206515101,
-30.7392409545507));
#21102=CARTESIAN_POINT('Ctrl Pts',(0.768469068537212,-0.879620246660906,
-30.7426065220351));
#21103=CARTESIAN_POINT('Ctrl Pts',(0.695440347491846,-0.938054764308324,
-30.7492738276346));
#21104=CARTESIAN_POINT('Ctrl Pts',(0.658559073910089,-0.964127226949575,
-30.7525210802118));
#21105=CARTESIAN_POINT('Ctrl Pts',(0.582208819688217,-1.01174476378742,
-30.7588592772385));
#21106=CARTESIAN_POINT('Ctrl Pts',(0.542749389348318,-1.03331199398362,
-30.7619381584573));
#21107=CARTESIAN_POINT('Ctrl Pts',(0.416276876357301,-1.09342586330311,
-30.7713609849539));
#21108=CARTESIAN_POINT('Ctrl Pts',(0.325380070116385,-1.12400298222979,
-30.7775132584775));
#21109=CARTESIAN_POINT('Ctrl Pts',(0.190071498834436,-1.15190522952279,
-30.7866412473092));
#21110=CARTESIAN_POINT('Ctrl Pts',(0.147470992919353,-1.15827142163799,
-30.7895119494768));
#21111=CARTESIAN_POINT('Ctrl Pts',(0.0195633985643735,-1.17004221305817,
-30.7982779098936));
#21112=CARTESIAN_POINT('Ctrl Pts',(-0.0653833390363976,-1.16807622863429,
-30.8044159856939));
#21113=CARTESIAN_POINT('Ctrl Pts',(-0.191666563688748,-1.15140566703514,
-30.8135099611217));
#21114=CARTESIAN_POINT('Ctrl Pts',(-0.233832913002153,-1.14346534826818,
-30.816515879701));
#21115=CARTESIAN_POINT('Ctrl Pts',(-0.366314577040543,-1.11102808203377,
-30.8258099429263));
#21116=CARTESIAN_POINT('Ctrl Pts',(-0.4546293910922,-1.07804391131431,-30.8318420499684));
#21117=CARTESIAN_POINT('Ctrl Pts',(-0.576506740473783,-1.01517446868446,
-30.8408040974894));
#21118=CARTESIAN_POINT('Ctrl Pts',(-0.614124897463469,-0.993041057591312,
-30.8436721997507));
#21119=CARTESIAN_POINT('Ctrl Pts',(-0.681414838461067,-0.948091679732547,
-30.8491193011929));
#21120=CARTESIAN_POINT('Ctrl Pts',(-0.711441123643893,-0.925834257978619,
-30.8516833011831));
#21121=CARTESIAN_POINT('Ctrl Pts',(-0.79022740139402,-0.861034604049957,
-30.8588671848167));
#21122=CARTESIAN_POINT('Ctrl Pts',(-0.836508566353444,-0.815801487855969,
-30.8635724603074));
#21123=CARTESIAN_POINT('Ctrl Pts',(-0.905208129760981,-0.736646372968856,
-30.8710613864576));
#21124=CARTESIAN_POINT('Ctrl Pts',(-0.930070295231557,-0.704839956840183,
-30.8738968769317));
#21125=CARTESIAN_POINT('Ctrl Pts',(-0.982286842236417,-0.630564553449005,
-30.8800889328438));
#21126=CARTESIAN_POINT('Ctrl Pts',(-1.00869765789631,-0.587422341858284,
-30.883418330516));
#21127=CARTESIAN_POINT('Ctrl Pts',(-1.06170501340571,-0.48702278699212,
-30.8908180465144));
#21128=CARTESIAN_POINT('Ctrl Pts',(-1.08671765906662,-0.428906450045411,
-30.8948688018013));
#21129=CARTESIAN_POINT('Ctrl Pts',(-1.12002448009141,-0.329971499936298,
-30.9017422583765));
#21130=CARTESIAN_POINT('Ctrl Pts',(-1.1311068495569,-0.29009808489723,-30.9045072036108));
#21131=CARTESIAN_POINT('Ctrl Pts',(-1.15123618562205,-0.198246548887531,
-30.9109945668488));
#21132=CARTESIAN_POINT('Ctrl Pts',(-1.15886629216208,-0.146014505077338,
-30.9147706560545));
#21133=CARTESIAN_POINT('Ctrl Pts',(-1.16642753965937,-0.0483358449972948,
-30.921828495974));
#21134=CARTESIAN_POINT('Ctrl Pts',(-1.16728315965028,-0.00293675892899701,
-30.9251063416237));
#21135=CARTESIAN_POINT('Ctrl Pts',(-1.16423412848984,0.0764793241860627,
-30.9307261307089));
#21136=CARTESIAN_POINT('Ctrl Pts',(-1.16145205542447,0.110545851708783,
-30.9330939648108));
#21137=CARTESIAN_POINT('Ctrl Pts',(-1.1507630119261,0.196040296314932,-30.9389159856546));
#21138=CARTESIAN_POINT('Ctrl Pts',(-1.14093638520118,0.247240011612176,
-30.9423091552743));
#21139=CARTESIAN_POINT('Ctrl Pts',(-1.11415509775947,0.349773164106084,
-30.9491663254526));
#21140=CARTESIAN_POINT('Ctrl Pts',(-1.09694525695557,0.401049399726515,
-30.9526299660782));
#21141=CARTESIAN_POINT('Ctrl Pts',(-1.06191971430983,0.485244558921056,
-30.9586301629196));
#21142=CARTESIAN_POINT('Ctrl Pts',(-1.04592843859889,0.518966246414727,
-30.9611252077559));
#21143=CARTESIAN_POINT('Ctrl Pts',(-1.00667850457887,0.592004102249595,
-30.9668413737592));
#21144=CARTESIAN_POINT('Ctrl Pts',(-0.982690543030822,0.630789580669632,
-30.9700809744543));
#21145=CARTESIAN_POINT('Ctrl Pts',(-0.92577731115898,0.711764805256299,
-30.9771871833879));
#21146=CARTESIAN_POINT('Ctrl Pts',(-0.892021085752503,0.753375714006476,
-30.9810643272464));
#21147=CARTESIAN_POINT('Ctrl Pts',(-0.831157513826872,0.81885589047688,
-30.9874031052895));
#21148=CARTESIAN_POINT('Ctrl Pts',(-0.805487538846159,0.844079160218681,
-30.9899110954614));
#21149=CARTESIAN_POINT('Ctrl Pts',(-0.741884245488248,0.901166354308377,
-30.995701440776));
#21150=CARTESIAN_POINT('Ctrl Pts',(-0.702972232118756,0.931952904362451,
-30.9989337662652));
#21151=CARTESIAN_POINT('Ctrl Pts',(-0.618514271893681,0.990541324608438,
-31.0055765993046));
#21152=CARTESIAN_POINT('Ctrl Pts',(-0.572684700748231,1.01794232834898,
-31.0089834107297));
#21153=CARTESIAN_POINT('Ctrl Pts',(-0.49255597576707,1.05855280552911,-31.0148746919682));
#21154=CARTESIAN_POINT('Ctrl Pts',(-0.459157642464918,1.07351338031607,
-31.0173157459797));
#21155=CARTESIAN_POINT('Ctrl Pts',(-0.362257512762512,1.11129644287772,
-31.0244646695162));
#21156=CARTESIAN_POINT('Ctrl Pts',(-0.297410848298703,1.13011301102836,
-31.0292997106953));
#21157=CARTESIAN_POINT('Ctrl Pts',(-0.187124706409844,1.15211935516333,
-31.0373816939126));
#21158=CARTESIAN_POINT('Ctrl Pts',(-0.142289990560102,1.15841330716532,
-31.0406284239081));
#21159=CARTESIAN_POINT('Ctrl Pts',(-0.063176738898904,1.16497102653747,
-31.046208231521));
#21160=CARTESIAN_POINT('Ctrl Pts',(-0.0289746663040221,1.16633112542234,
-31.0485702431819));
#21161=CARTESIAN_POINT('Ctrl Pts',(0.0593084551231717,1.16604144539294,
-31.0545031810733));
#21162=CARTESIAN_POINT('Ctrl Pts',(0.113395661910786,1.16218189970294,-31.0579956853853));
#21163=CARTESIAN_POINT('Ctrl Pts',(0.224842541394679,1.14641006745828,-31.0652428658355));
#21164=CARTESIAN_POINT('Ctrl Pts',(0.282100957497795,1.1338736788578,-31.0689971062012));
#21165=CARTESIAN_POINT('Ctrl Pts',(0.374052171032848,1.10606227821236,-31.0754427222994));
#21166=CARTESIAN_POINT('Ctrl Pts',(0.409453520323982,1.09337035163398,-31.0780348427351));
#21167=CARTESIAN_POINT('Ctrl Pts',(0.517476805264023,1.04857455727421,-31.0862385359748));
#21168=CARTESIAN_POINT('Ctrl Pts',(0.587682831432323,1.01055892366634,-31.0920033516305));
#21169=CARTESIAN_POINT('Ctrl Pts',(0.690824163490302,0.940622392373098,
-31.1008475785035));
#21170=CARTESIAN_POINT('Ctrl Pts',(0.72681028023883,0.913113517205756,-31.1040148988039));
#21171=CARTESIAN_POINT('Ctrl Pts',(0.817984776836416,0.834813237889736,
-31.1121663288315));
#21172=CARTESIAN_POINT('Ctrl Pts',(0.870253412544716,0.780594317299417,
-31.1169396107474));
#21173=CARTESIAN_POINT('Ctrl Pts',(0.937220513377292,0.695987892557664,
-31.1239148245526));
#21174=CARTESIAN_POINT('Ctrl Pts',(0.956547942992973,0.669287829234583,
-31.1260589017073));
#21175=CARTESIAN_POINT('Ctrl Pts',(0.996400989999189,0.60878603062681,-31.1308845701165));
#21176=CARTESIAN_POINT('Ctrl Pts',(1.01635907202192,0.574675644168678,-31.1335875623297));
#21177=CARTESIAN_POINT('Ctrl Pts',(1.07408883199262,0.46327759563795,-31.1423270895464));
#21178=CARTESIAN_POINT('Ctrl Pts',(1.1051196110236,0.382453701872699,-31.1485422957239));
#21179=CARTESIAN_POINT('Ctrl Pts',(1.13988537104464,0.251184830520502,-31.1581469742182));
#21180=CARTESIAN_POINT('Ctrl Pts',(1.14962127517682,0.202259736242942,-31.1616242141299));
#21181=CARTESIAN_POINT('Ctrl Pts',(1.16481115260415,0.0892323089346831,
-31.1693363582519));
#21182=CARTESIAN_POINT('Ctrl Pts',(1.16819757460234,0.0248471507560758,
-31.173462210906));
#21183=CARTESIAN_POINT('Ctrl Pts',(1.16505492615128,-0.0755507344237222,
-31.1799619715207));
#21184=CARTESIAN_POINT('Ctrl Pts',(1.16221017433194,-0.111704713006625,
-31.182319041523));
#21185=CARTESIAN_POINT('Ctrl Pts',(1.15158005006472,-0.194696702061016,
-31.1879013545843));
#21186=CARTESIAN_POINT('Ctrl Pts',(1.14259382155944,-0.241266739154483,
-31.1911518502856));
#21187=CARTESIAN_POINT('Ctrl Pts',(1.10912772555809,-0.371437981360074,
-31.2005258451499));
#21188=CARTESIAN_POINT('Ctrl Pts',(1.07796884465094,-0.453349820889493,
-31.2067744058992));
#21189=CARTESIAN_POINT('Ctrl Pts',(1.01993868550944,-0.566914805651578,
-31.2157311300408));
#21190=CARTESIAN_POINT('Ctrl Pts',(0.999685483652604,-0.602026275118691,
-31.2185454180568));
#21191=CARTESIAN_POINT('Ctrl Pts',(0.943447679441216,-0.688917601007358,
-31.2255910197575));
#21192=CARTESIAN_POINT('Ctrl Pts',(0.904986255469571,-0.739088189196026,
-31.2296842482066));
#21193=CARTESIAN_POINT('Ctrl Pts',(0.83239505206359,-0.819144896900878,
-31.2367052600699));
#21194=CARTESIAN_POINT('Ctrl Pts',(0.800287439985633,-0.850591997282813,
-31.2396426579672));
#21195=CARTESIAN_POINT('Ctrl Pts',(0.677247083649768,-0.957343264563837,
-31.2506083772752));
#21196=CARTESIAN_POINT('Ctrl Pts',(0.576361367480104,-1.02061902569622,
-31.2589908100937));
#21197=CARTESIAN_POINT('Ctrl Pts',(0.421633955074437,-1.08851278412317,
-31.2708526489429));
#21198=CARTESIAN_POINT('Ctrl Pts',(0.373333306378296,-1.1060982468434,-31.274429506583));
#21199=CARTESIAN_POINT('Ctrl Pts',(0.268024200900743,-1.13685382344944,
-31.2819219010863));
#21200=CARTESIAN_POINT('Ctrl Pts',(0.210733858165044,-1.14907162017185,
-31.2857759753666));
#21201=CARTESIAN_POINT('Ctrl Pts',(0.0850061683590383,-1.16595350028459,
-31.2940714011991));
#21202=CARTESIAN_POINT('Ctrl Pts',(0.0171193143066746,-1.16881571421432,
-31.2985589381589));
#21203=CARTESIAN_POINT('Ctrl Pts',(-0.170348216791286,-1.16010129180361,
-31.3113707279674));
#21204=CARTESIAN_POINT('Ctrl Pts',(-0.289034321660633,-1.13599694319867,
-31.3198463246205));
#21205=CARTESIAN_POINT('Ctrl Pts',(-0.468120182557069,-1.07066515186562,
-31.3330824400782));
#21206=CARTESIAN_POINT('Ctrl Pts',(-0.532693517969684,-1.04033994702365,
-31.3379530166625));
#21207=CARTESIAN_POINT('Ctrl Pts',(-0.625391610677575,-0.985851723054238,
-31.3450977313131));
#21208=CARTESIAN_POINT('Ctrl Pts',(-0.655959765253003,-0.965871197408253,
-31.3474902215926));
#21209=CARTESIAN_POINT('Ctrl Pts',(-0.777879976153246,-0.877380172770267,
-31.357486367411));
#21210=CARTESIAN_POINT('Ctrl Pts',(-0.859912618212914,-0.796237594718653,
-31.3653439434294));
#21211=CARTESIAN_POINT('Ctrl Pts',(-0.975254435297355,-0.643948339349487,
-31.3785854260959));
#21212=CARTESIAN_POINT('Ctrl Pts',(-1.01577210878922,-0.578125335361136,
-31.3839392354365));
#21213=CARTESIAN_POINT('Ctrl Pts',(-1.10899380208953,-0.387246913439551,
-31.3985453285889));
#21214=CARTESIAN_POINT('Ctrl Pts',(-1.14344335550353,-0.264663157205293,
-31.4068122887934));
#21215=CARTESIAN_POINT('Ctrl Pts',(-1.17590076084456,0.00819027975376396,
-31.4254655864227));
#21216=CARTESIAN_POINT('Ctrl Pts',(-1.16463926395832,0.161289680328769,
-31.4359077152906));
#21217=CARTESIAN_POINT('Ctrl Pts',(-1.08535270579174,0.45572979035119,-31.4568415946505));
#21218=CARTESIAN_POINT('Ctrl Pts',(-1.01670874950091,0.592794756408663,
-31.466956769279));
#21219=CARTESIAN_POINT('Ctrl Pts',(-0.827849909053765,0.83538314803652,
-31.487852646732));
#21220=CARTESIAN_POINT('Ctrl Pts',(-0.709617583089645,0.93843676949597,
-31.4983682348508));
#21221=CARTESIAN_POINT('Ctrl Pts',(-0.511147348714834,1.05180989497623,
-31.5140645531066));
#21222=CARTESIAN_POINT('Ctrl Pts',(-0.443272565048419,1.08210604098259,
-31.5191611936776));
#21223=CARTESIAN_POINT('Ctrl Pts',(-0.230901793688486,1.15296249320239,
-31.5344190291072));
#21224=CARTESIAN_POINT('Ctrl Pts',(-0.0801266960605881,1.17280484436255,
-31.5444358079042));
#21225=CARTESIAN_POINT('Ctrl Pts',(0.221971670579917,1.15577877094791,-31.5650280299048));
#21226=CARTESIAN_POINT('Ctrl Pts',(0.369673902437772,1.11746614756773,-31.575591324995));
#21227=CARTESIAN_POINT('Ctrl Pts',(0.622160525775805,0.994452459531914,
-31.5946539956718));
#21228=CARTESIAN_POINT('Ctrl Pts',(0.727539007713757,0.920189142633611,
-31.6030889670126));
#21229=CARTESIAN_POINT('Ctrl Pts',(0.916982964614389,0.73477608994851,-31.6210410579286));
#21230=CARTESIAN_POINT('Ctrl Pts',(0.996272708142201,0.623142279337944,
-31.6307046019878));
#21231=CARTESIAN_POINT('Ctrl Pts',(1.08433698239759,0.435193202490311,-31.6449148687832));
#21232=CARTESIAN_POINT('Ctrl Pts',(1.10822642430814,0.369663308560383,-31.6495634464446));
#21233=CARTESIAN_POINT('Ctrl Pts',(1.15766448812734,0.185711327184666,-31.6622430262217));
#21234=CARTESIAN_POINT('Ctrl Pts',(1.17132519379187,0.0639675994095021,
-31.6702435733044));
#21235=CARTESIAN_POINT('Ctrl Pts',(1.16300828851598,-0.110853971756192,
-31.6824209503072));
#21236=CARTESIAN_POINT('Ctrl Pts',(1.15655334679051,-0.164270613099354,
-31.6862649953204));
#21237=CARTESIAN_POINT('Ctrl Pts',(1.13596513152833,-0.271414406573397,
-31.6939847321905));
#21238=CARTESIAN_POINT('Ctrl Pts',(1.1215795497405,-0.325113706990364,-31.6978144376222));
#21239=CARTESIAN_POINT('Ctrl Pts',(1.08263550331581,-0.438176204048292,
-31.7058935031972));
#21240=CARTESIAN_POINT('Ctrl Pts',(1.05682806402532,-0.497140478928953,
-31.7101306170283));
#21241=CARTESIAN_POINT('Ctrl Pts',(0.98300300796349,-0.63449965815748,-31.7204223140629));
#21242=CARTESIAN_POINT('Ctrl Pts',(0.930173045980556,-0.710361834246211,
-31.7264812348101));
#21243=CARTESIAN_POINT('Ctrl Pts',(0.838930525074047,-0.812502698043108,
-31.7359377792509));
#21244=CARTESIAN_POINT('Ctrl Pts',(0.807039546152215,-0.844135571885244,
-31.7391179237103));
#21245=CARTESIAN_POINT('Ctrl Pts',(0.726353665209184,-0.91520566837048,
-31.746804006435));
#21246=CARTESIAN_POINT('Ctrl Pts',(0.676066014753284,-0.952672061924379,
-31.7512732634903));
#21247=CARTESIAN_POINT('Ctrl Pts',(0.586597396153142,-1.00892317739801,
-31.7585101855706));
#21248=CARTESIAN_POINT('Ctrl Pts',(0.548805759549127,-1.02989821143397,
-31.7614003698864));
#21249=CARTESIAN_POINT('Ctrl Pts',(0.431409242179501,-1.08697182239586,
-31.7700425151364));
#21250=CARTESIAN_POINT('Ctrl Pts',(0.348579506835605,-1.11657141359353,
-31.7756961700068));
#21251=CARTESIAN_POINT('Ctrl Pts',(0.217677855472974,-1.14733111137362,
-31.7846649392895));
#21252=CARTESIAN_POINT('Ctrl Pts',(0.171191373914171,-1.15531031302035,
-31.7878568696945));
#21253=CARTESIAN_POINT('Ctrl Pts',(0.0895549583645699,-1.16408050808528,
-31.7935895247711));
#21254=CARTESIAN_POINT('Ctrl Pts',(0.054609741640134,-1.16617767881962,
-31.796086555492));
#21255=CARTESIAN_POINT('Ctrl Pts',(-0.0467913736064708,-1.16763349643548,
-31.8033629679176));
#21256=CARTESIAN_POINT('Ctrl Pts',(-0.113337928350958,-1.16281548208516,
-31.8081612838819));
#21257=CARTESIAN_POINT('Ctrl Pts',(-0.235278263563502,-1.14362810067056,
-31.8166300151622));
#21258=CARTESIAN_POINT('Ctrl Pts',(-0.290908321981227,-1.13073008081567,
-31.8204024646212));
#21259=CARTESIAN_POINT('Ctrl Pts',(-0.444812112979426,-1.08322628172866,
-31.830945564078));
#21260=CARTESIAN_POINT('Ctrl Pts',(-0.540311217364741,-1.03946587487301,
-31.837621805171));
#21261=CARTESIAN_POINT('Ctrl Pts',(-0.673100283251339,-0.954845681333125,
-31.8484417282243));
#21262=CARTESIAN_POINT('Ctrl Pts',(-0.715792773943846,-0.923107745328805,
-31.8522365879894));
#21263=CARTESIAN_POINT('Ctrl Pts',(-0.803852241302621,-0.847752091635972,
-31.8605787399954));
#21264=CARTESIAN_POINT('Ctrl Pts',(-0.848313210756834,-0.802950806528635,
-31.8651310439244));
#21265=CARTESIAN_POINT('Ctrl Pts',(-0.916115433980169,-0.722848737228883,
-31.8723664669261));
#21266=CARTESIAN_POINT('Ctrl Pts',(-0.941571571027832,-0.689329219815559,
-31.8751785748015));
#21267=CARTESIAN_POINT('Ctrl Pts',(-0.99975857647731,-0.603675302149774,
-31.8819956493985));
#21268=CARTESIAN_POINT('Ctrl Pts',(-1.03040277506431,-0.550095551789753,
-31.88595080696));
#21269=CARTESIAN_POINT('Ctrl Pts',(-1.07866822297917,-0.447757935699058,
-31.8933197268893));
#21270=CARTESIAN_POINT('Ctrl Pts',(-1.09758968721411,-0.399614243566427,
-31.8967191126898));
#21271=CARTESIAN_POINT('Ctrl Pts',(-1.12524986139922,-0.312005362231876,
-31.9029894599813));
#21272=CARTESIAN_POINT('Ctrl Pts',(-1.13524081419106,-0.273143485089577,
-31.9058100800701));
#21273=CARTESIAN_POINT('Ctrl Pts',(-1.15655793595677,-0.167633623548991,
-31.9134992139986));
#21274=CARTESIAN_POINT('Ctrl Pts',(-1.16408685545047,-0.100190605984288,
-31.9184390059287));
#21275=CARTESIAN_POINT('Ctrl Pts',(-1.16671949918186,0.000995598857348756,
-31.9255822026249));
#21276=CARTESIAN_POINT('Ctrl Pts',(-1.16616740721873,0.0346408626275563,
-31.927906725977));
#21277=CARTESIAN_POINT('Ctrl Pts',(-1.16225049598424,0.101363110558704,
-31.9324145875288));
#21278=CARTESIAN_POINT('Ctrl Pts',(-1.15891999235791,0.134442845400991,
-31.9346064296027));
#21279=CARTESIAN_POINT('Ctrl Pts',(-1.14378268241922,0.240159071561426,
-31.9415747696343));
#21280=CARTESIAN_POINT('Ctrl Pts',(-1.12659062347451,0.312042548769722,
-31.9462565676558));
#21281=CARTESIAN_POINT('Ctrl Pts',(-1.09092949322726,0.415884557053626,
-31.9534961242054));
#21282=CARTESIAN_POINT('Ctrl Pts',(-1.07752966429866,0.449614269739891,
-31.9559292779484));
#21283=CARTESIAN_POINT('Ctrl Pts',(-1.0374731109826,0.537627087276782,-31.9626076401286));
#21284=CARTESIAN_POINT('Ctrl Pts',(-1.00807686224237,0.590494188094113,
-31.9669474270401));
#21285=CARTESIAN_POINT('Ctrl Pts',(-0.939126696925382,0.694708303515753,
-31.9759472815253));
#21286=CARTESIAN_POINT('Ctrl Pts',(-0.898980851929762,0.745692992216044,
-31.9806067047616));
#21287=CARTESIAN_POINT('Ctrl Pts',(-0.830179916132025,0.819829954206266,
-31.987550978645));
#21288=CARTESIAN_POINT('Ctrl Pts',(-0.804137417975539,0.845434094234728,
-31.9899822639371));
#21289=CARTESIAN_POINT('Ctrl Pts',(-0.737655511072942,0.905038542932737,
-31.9958345678478));
#21290=CARTESIAN_POINT('Ctrl Pts',(-0.695981335925813,0.937675454780674,
-31.9992128271908));
#21291=CARTESIAN_POINT('Ctrl Pts',(-0.612847639332127,0.994093419831662,
-32.0057054755517));
#21292=CARTESIAN_POINT('Ctrl Pts',(-0.571771963705075,1.01842145541926,
-32.0088137038318));
#21293=CARTESIAN_POINT('Ctrl Pts',(-0.495496118829579,1.05726047115192,
-32.0146036163438));
#21294=CARTESIAN_POINT('Ctrl Pts',(-0.460858658671628,1.07272788565039,
-32.0172423593459));
#21295=CARTESIAN_POINT('Ctrl Pts',(-0.375133633164121,1.10604743893886,
-32.0237480290935));
#21296=CARTESIAN_POINT('Ctrl Pts',(-0.323309374888746,1.12209275398005,
-32.0276600588066));
#21297=CARTESIAN_POINT('Ctrl Pts',(-0.221635181656419,1.14609414865391,
-32.035151397609));
#21298=CARTESIAN_POINT('Ctrl Pts',(-0.171876293416826,1.15454058196787,
-32.0387355372415));
#21299=CARTESIAN_POINT('Ctrl Pts',(-0.0877502387182354,1.16340157106644,
-32.0445526251554));
#21300=CARTESIAN_POINT('Ctrl Pts',(-0.0535558392802562,1.16552299988754,
-32.0468426510691));
#21301=CARTESIAN_POINT('Ctrl Pts',(0.0270083813386109,1.16703043450772,
-32.0521342104412));
#21302=CARTESIAN_POINT('Ctrl Pts',(0.0734045328626228,1.16518204041798,
-32.0551059263961));
#21303=CARTESIAN_POINT('Ctrl Pts',(0.171858372962463,1.15533764184338,-32.0614809553558));
#21304=CARTESIAN_POINT('Ctrl Pts',(0.223908914150883,1.14653962663329,-32.064894866051));
#21305=CARTESIAN_POINT('Ctrl Pts',(0.316431900889636,1.12404973179581,-32.0713318545482));
#21306=CARTESIAN_POINT('Ctrl Pts',(0.357074873436082,1.11169392879419,-32.0742859596744));
#21307=CARTESIAN_POINT('Ctrl Pts',(0.456782879970018,1.07529717055788,-32.0817878254199));
#21308=CARTESIAN_POINT('Ctrl Pts',(0.514847053636697,1.04850353644109,-32.0863907615577));
#21309=CARTESIAN_POINT('Ctrl Pts',(0.609764637786685,0.995107450904462,
-32.0941404178487));
#21310=CARTESIAN_POINT('Ctrl Pts',(0.64789339688654,0.970707018317168,-32.0973219442031));
#21311=CARTESIAN_POINT('Ctrl Pts',(0.715151547512504,0.922068492094722,
-32.1029949487002));
#21312=CARTESIAN_POINT('Ctrl Pts',(0.744736439003466,0.898452960557686,
-32.1055032684934));
#21313=CARTESIAN_POINT('Ctrl Pts',(0.818267481323139,0.83372917772617,-32.1118913711226));
#21314=CARTESIAN_POINT('Ctrl Pts',(0.860368514566787,0.790533037148104,
-32.1157159401581));
#21315=CARTESIAN_POINT('Ctrl Pts',(0.923449901262993,0.71458664340485,-32.1221795037161));
#21316=CARTESIAN_POINT('Ctrl Pts',(0.94642154334661,0.68384088381028,-32.1247457808902));
#21317=CARTESIAN_POINT('Ctrl Pts',(1.00557045651288,0.59563248486742,-32.1320332235485));
#21318=CARTESIAN_POINT('Ctrl Pts',(1.03824014728665,0.536068984602925,-32.1368509098396));
#21319=CARTESIAN_POINT('Ctrl Pts',(1.09664652215412,0.403931737157978,-32.1471559960423));
#21320=CARTESIAN_POINT('Ctrl Pts',(1.12088236127104,0.330622819452228,-32.152646886106));
#21321=CARTESIAN_POINT('Ctrl Pts',(1.14658333970841,0.217189487467516,-32.1605896802752));
#21322=CARTESIAN_POINT('Ctrl Pts',(1.15339342276266,0.178237339655661,-32.1632099946067));
#21323=CARTESIAN_POINT('Ctrl Pts',(1.16657974788419,0.0711945325339807,
-32.1702374938604));
#21324=CARTESIAN_POINT('Ctrl Pts',(1.16901560357053,0.00250273317850058,
-32.1745827432116));
#21325=CARTESIAN_POINT('Ctrl Pts',(1.16242719852251,-0.113341789505422,
-32.1823079664126));
#21326=CARTESIAN_POINT('Ctrl Pts',(1.15674237783295,-0.160460199536454,
-32.1855532645071));
#21327=CARTESIAN_POINT('Ctrl Pts',(1.13876044634579,-0.258614577418294,
-32.1925001731439));
#21328=CARTESIAN_POINT('Ctrl Pts',(1.12582551001773,-0.309528934911987,
-32.1962128878324));
#21329=CARTESIAN_POINT('Ctrl Pts',(1.10959412583112,-0.35936066950901,-32.1999249889109));
#21330=CARTESIAN_POINT('Ctrl Pts',(-1.015482192511,0.5750263216907,-30.425575843));
#21331=CARTESIAN_POINT('Ctrl Pts',(-0.8824095367636,0.8100293243789,-30.44399167037));
#21332=CARTESIAN_POINT('Ctrl Pts',(-0.4470880869402,1.18276829068,-30.48082332512));
#21333=CARTESIAN_POINT('Ctrl Pts',(0.4133389835427,1.195144688561,-30.53607080725));
#21334=CARTESIAN_POINT('Ctrl Pts',(1.082287319525,0.6540128508907,-30.59131828937));
#21335=CARTESIAN_POINT('Ctrl Pts',(1.250228977982,-0.189832146326,-30.6465657715));
#21336=CARTESIAN_POINT('Ctrl Pts',(0.8393735447346,-0.945811051386,-30.70181325362));
#21337=CARTESIAN_POINT('Ctrl Pts',(0.03993616735796,-1.263926564634,-30.75706073575));
#21338=CARTESIAN_POINT('Ctrl Pts',(-0.7779901316111,-0.9969138795045,-30.81230821787));
#21339=CARTESIAN_POINT('Ctrl Pts',(-1.235749089843,-0.2683839185767,-30.8675557));
#21340=CARTESIAN_POINT('Ctrl Pts',(-1.121423396098,0.5843931352325,-30.92280318212));
#21341=CARTESIAN_POINT('Ctrl Pts',(-0.4879395772335,1.166627935668,-30.97805066425));
#21342=CARTESIAN_POINT('Ctrl Pts',(0.3714337559552,1.208777371376,-31.03329814637));
#21343=CARTESIAN_POINT('Ctrl Pts',(1.058853438626,0.691328550783,-31.0885456285));
#21344=CARTESIAN_POINT('Ctrl Pts',(1.256081499646,-0.1461678338278,-31.14379311062));
#21345=CARTESIAN_POINT('Ctrl Pts',(0.8718120611923,-0.9159964516181,-31.19904059275));
#21346=CARTESIAN_POINT('Ctrl Pts',(0.08394099831018,-1.261768472513,-31.25428807487));
#21347=CARTESIAN_POINT('Ctrl Pts',(-0.7427901868119,-1.023410234361,-31.309535557));
#21348=CARTESIAN_POINT('Ctrl Pts',(-1.225649866438,-0.3112686529751,-31.36478303912));
#21349=CARTESIAN_POINT('Ctrl Pts',(-1.141100239542,0.5449734055297,-31.42003052125));
#21350=CARTESIAN_POINT('Ctrl Pts',(-0.5282831903702,1.148922382135,-31.47527800337));
#21351=CARTESIAN_POINT('Ctrl Pts',(0.3291002778155,1.220982709444,-31.5305254855));
#21352=CARTESIAN_POINT('Ctrl Pts',(1.034128194939,0.7277943700298,-31.58577296762));
#21353=CARTESIAN_POINT('Ctrl Pts',(1.260410936535,-0.1023232250025,-31.64102044975));
#21354=CARTESIAN_POINT('Ctrl Pts',(0.9031918799483,-0.8850707304042,-31.69626793187));
#21355=CARTESIAN_POINT('Ctrl Pts',(0.1278440645328,-1.258078549202,-31.751515414));
#21356=CARTESIAN_POINT('Ctrl Pts',(-0.7066886712758,-1.048664412443,-31.80676289612));
#21357=CARTESIAN_POINT('Ctrl Pts',(-1.214062705292,-0.3537753607434,-31.86201037825));
#21358=CARTESIAN_POINT('Ctrl Pts',(-1.159392542789,0.5048914975012,-31.91725786037));
#21359=CARTESIAN_POINT('Ctrl Pts',(-0.5679833167426,1.129824629341,-31.9725053425));
#21360=CARTESIAN_POINT('Ctrl Pts',(0.2863590197545,1.23169686325,-32.02775282462));
#21361=CARTESIAN_POINT('Ctrl Pts',(1.008178628936,0.7634106326662,-32.08300030675));
#21362=CARTESIAN_POINT('Ctrl Pts',(1.263094839915,-0.05848087125908,-32.13824778887));
#21363=CARTESIAN_POINT('Ctrl Pts',(1.043636050887,-0.5878927540068,-32.17507944362));
#21364=CARTESIAN_POINT('Ctrl Pts',(0.8614506246688,-0.7872497540188,-32.193495271));
#21365=CARTESIAN_POINT('Ctrl Pts',(-1.015482192511,0.5750263216907,-30.49106798064));
#21366=CARTESIAN_POINT('Ctrl Pts',(-0.8824095367636,0.8100293243789,-30.50948380802));
#21367=CARTESIAN_POINT('Ctrl Pts',(-0.4470880869402,1.18276829068,-30.54631546277));
#21368=CARTESIAN_POINT('Ctrl Pts',(0.4133389835427,1.195144688561,-30.60156294489));
#21369=CARTESIAN_POINT('Ctrl Pts',(1.082287319525,0.6540128508907,-30.65681042702));
#21370=CARTESIAN_POINT('Ctrl Pts',(1.250228977982,-0.189832146326,-30.71205790914));
#21371=CARTESIAN_POINT('Ctrl Pts',(0.8393735447346,-0.945811051386,-30.76730539127));
#21372=CARTESIAN_POINT('Ctrl Pts',(0.03993616735796,-1.263926564634,-30.82255287339));
#21373=CARTESIAN_POINT('Ctrl Pts',(-0.7779901316111,-0.9969138795045,-30.87780035552));
#21374=CARTESIAN_POINT('Ctrl Pts',(-1.235749089843,-0.2683839185767,-30.93304783764));
#21375=CARTESIAN_POINT('Ctrl Pts',(-1.121423396098,0.5843931352325,-30.98829531976));
#21376=CARTESIAN_POINT('Ctrl Pts',(-0.4879395772335,1.166627935668,-31.04354280189));
#21377=CARTESIAN_POINT('Ctrl Pts',(0.3714337559552,1.208777371376,-31.09879028401));
#21378=CARTESIAN_POINT('Ctrl Pts',(1.058853438626,0.691328550783,-31.15403776614));
#21379=CARTESIAN_POINT('Ctrl Pts',(1.256081499646,-0.1461678338278,-31.20928524826));
#21380=CARTESIAN_POINT('Ctrl Pts',(0.8718120611923,-0.9159964516181,-31.26453273039));
#21381=CARTESIAN_POINT('Ctrl Pts',(0.08394099831018,-1.261768472513,-31.31978021251));
#21382=CARTESIAN_POINT('Ctrl Pts',(-0.7427901868119,-1.023410234361,-31.37502769464));
#21383=CARTESIAN_POINT('Ctrl Pts',(-1.225649866438,-0.3112686529751,-31.43027517676));
#21384=CARTESIAN_POINT('Ctrl Pts',(-1.141100239542,0.5449734055297,-31.48552265889));
#21385=CARTESIAN_POINT('Ctrl Pts',(-0.5282831903702,1.148922382135,-31.54077014101));
#21386=CARTESIAN_POINT('Ctrl Pts',(0.3291002778155,1.220982709444,-31.59601762314));
#21387=CARTESIAN_POINT('Ctrl Pts',(1.034128194939,0.7277943700298,-31.65126510526));
#21388=CARTESIAN_POINT('Ctrl Pts',(1.260410936535,-0.1023232250025,-31.70651258739));
#21389=CARTESIAN_POINT('Ctrl Pts',(0.9031918799483,-0.8850707304042,-31.76176006951));
#21390=CARTESIAN_POINT('Ctrl Pts',(0.1278440645328,-1.258078549202,-31.81700755164));
#21391=CARTESIAN_POINT('Ctrl Pts',(-0.7066886712758,-1.048664412443,-31.87225503376));
#21392=CARTESIAN_POINT('Ctrl Pts',(-1.214062705292,-0.3537753607434,-31.92750251589));
#21393=CARTESIAN_POINT('Ctrl Pts',(-1.159392542789,0.5048914975012,-31.98274999801));
#21394=CARTESIAN_POINT('Ctrl Pts',(-0.5679833167426,1.129824629341,-32.03799748014));
#21395=CARTESIAN_POINT('Ctrl Pts',(0.2863590197545,1.23169686325,-32.09324496226));
#21396=CARTESIAN_POINT('Ctrl Pts',(1.008178628936,0.7634106326662,-32.14849244439));
#21397=CARTESIAN_POINT('Ctrl Pts',(1.263094839915,-0.05848087125908,-32.20373992651));
#21398=CARTESIAN_POINT('Ctrl Pts',(1.043636050887,-0.5878927540068,-32.24057158126));
#21399=CARTESIAN_POINT('Ctrl Pts',(0.8614506246688,-0.7872497540188,-32.25898740864));
#21400=CARTESIAN_POINT('Ctrl Pts',(-1.015482192511,0.5750263216907,-30.55656011828));
#21401=CARTESIAN_POINT('Ctrl Pts',(-0.8824095367636,0.8100293243789,-30.57497594566));
#21402=CARTESIAN_POINT('Ctrl Pts',(-0.4470880869402,1.18276829068,-30.61180760041));
#21403=CARTESIAN_POINT('Ctrl Pts',(0.4133389835427,1.195144688561,-30.66705508253));
#21404=CARTESIAN_POINT('Ctrl Pts',(1.082287319525,0.6540128508907,-30.72230256466));
#21405=CARTESIAN_POINT('Ctrl Pts',(1.250228977982,-0.189832146326,-30.77755004678));
#21406=CARTESIAN_POINT('Ctrl Pts',(0.8393735447346,-0.945811051386,-30.83279752891));
#21407=CARTESIAN_POINT('Ctrl Pts',(0.03993616735796,-1.263926564634,-30.88804501103));
#21408=CARTESIAN_POINT('Ctrl Pts',(-0.7779901316111,-0.9969138795045,-30.94329249316));
#21409=CARTESIAN_POINT('Ctrl Pts',(-1.235749089843,-0.2683839185767,-30.99853997528));
#21410=CARTESIAN_POINT('Ctrl Pts',(-1.121423396098,0.5843931352325,-31.05378745741));
#21411=CARTESIAN_POINT('Ctrl Pts',(-0.4879395772335,1.166627935668,-31.10903493953));
#21412=CARTESIAN_POINT('Ctrl Pts',(0.3714337559552,1.208777371376,-31.16428242166));
#21413=CARTESIAN_POINT('Ctrl Pts',(1.058853438626,0.691328550783,-31.21952990378));
#21414=CARTESIAN_POINT('Ctrl Pts',(1.256081499646,-0.1461678338278,-31.27477738591));
#21415=CARTESIAN_POINT('Ctrl Pts',(0.8718120611923,-0.9159964516181,-31.33002486803));
#21416=CARTESIAN_POINT('Ctrl Pts',(0.08394099831018,-1.261768472513,-31.38527235016));
#21417=CARTESIAN_POINT('Ctrl Pts',(-0.7427901868119,-1.023410234361,-31.44051983228));
#21418=CARTESIAN_POINT('Ctrl Pts',(-1.225649866438,-0.3112686529751,-31.4957673144));
#21419=CARTESIAN_POINT('Ctrl Pts',(-1.141100239542,0.5449734055297,-31.55101479653));
#21420=CARTESIAN_POINT('Ctrl Pts',(-0.5282831903702,1.148922382135,-31.60626227865));
#21421=CARTESIAN_POINT('Ctrl Pts',(0.3291002778155,1.220982709444,-31.66150976078));
#21422=CARTESIAN_POINT('Ctrl Pts',(1.034128194939,0.7277943700298,-31.7167572429));
#21423=CARTESIAN_POINT('Ctrl Pts',(1.260410936535,-0.1023232250025,-31.77200472503));
#21424=CARTESIAN_POINT('Ctrl Pts',(0.9031918799483,-0.8850707304042,-31.82725220715));
#21425=CARTESIAN_POINT('Ctrl Pts',(0.1278440645328,-1.258078549202,-31.88249968928));
#21426=CARTESIAN_POINT('Ctrl Pts',(-0.7066886712758,-1.048664412443,-31.9377471714));
#21427=CARTESIAN_POINT('Ctrl Pts',(-1.214062705292,-0.3537753607434,-31.99299465353));
#21428=CARTESIAN_POINT('Ctrl Pts',(-1.159392542789,0.5048914975012,-32.04824213565));
#21429=CARTESIAN_POINT('Ctrl Pts',(-0.5679833167426,1.129824629341,-32.10348961778));
#21430=CARTESIAN_POINT('Ctrl Pts',(0.2863590197545,1.23169686325,-32.1587370999));
#21431=CARTESIAN_POINT('Ctrl Pts',(1.008178628936,0.7634106326662,-32.21398458203));
#21432=CARTESIAN_POINT('Ctrl Pts',(1.263094839915,-0.05848087125908,-32.26923206415));
#21433=CARTESIAN_POINT('Ctrl Pts',(1.043636050887,-0.5878927540068,-32.3060637189));
#21434=CARTESIAN_POINT('Ctrl Pts',(0.8614506246688,-0.7872497540188,-32.32447954628));
#21435=CARTESIAN_POINT('Ctrl Pts',(-1.015482192511,0.5750263216907,-30.62205225592));
#21436=CARTESIAN_POINT('Ctrl Pts',(-0.8824095367636,0.8100293243789,-30.6404680833));
#21437=CARTESIAN_POINT('Ctrl Pts',(-0.4470880869402,1.18276829068,-30.67729973805));
#21438=CARTESIAN_POINT('Ctrl Pts',(0.4133389835427,1.195144688561,-30.73254722017));
#21439=CARTESIAN_POINT('Ctrl Pts',(1.082287319525,0.6540128508907,-30.7877947023));
#21440=CARTESIAN_POINT('Ctrl Pts',(1.250228977982,-0.189832146326,-30.84304218442));
#21441=CARTESIAN_POINT('Ctrl Pts',(0.8393735447346,-0.945811051386,-30.89828966655));
#21442=CARTESIAN_POINT('Ctrl Pts',(0.03993616735796,-1.263926564634,-30.95353714867));
#21443=CARTESIAN_POINT('Ctrl Pts',(-0.7779901316111,-0.9969138795045,-31.0087846308));
#21444=CARTESIAN_POINT('Ctrl Pts',(-1.235749089843,-0.2683839185767,-31.06403211292));
#21445=CARTESIAN_POINT('Ctrl Pts',(-1.121423396098,0.5843931352325,-31.11927959505));
#21446=CARTESIAN_POINT('Ctrl Pts',(-0.4879395772335,1.166627935668,-31.17452707717));
#21447=CARTESIAN_POINT('Ctrl Pts',(0.3714337559552,1.208777371376,-31.2297745593));
#21448=CARTESIAN_POINT('Ctrl Pts',(1.058853438626,0.691328550783,-31.28502204142));
#21449=CARTESIAN_POINT('Ctrl Pts',(1.256081499646,-0.1461678338278,-31.34026952355));
#21450=CARTESIAN_POINT('Ctrl Pts',(0.8718120611923,-0.9159964516181,-31.39551700567));
#21451=CARTESIAN_POINT('Ctrl Pts',(0.08394099831018,-1.261768472513,-31.4507644878));
#21452=CARTESIAN_POINT('Ctrl Pts',(-0.7427901868119,-1.023410234361,-31.50601196992));
#21453=CARTESIAN_POINT('Ctrl Pts',(-1.225649866438,-0.3112686529751,-31.56125945205));
#21454=CARTESIAN_POINT('Ctrl Pts',(-1.141100239542,0.5449734055297,-31.61650693417));
#21455=CARTESIAN_POINT('Ctrl Pts',(-0.5282831903702,1.148922382135,-31.6717544163));
#21456=CARTESIAN_POINT('Ctrl Pts',(0.3291002778155,1.220982709444,-31.72700189842));
#21457=CARTESIAN_POINT('Ctrl Pts',(1.034128194939,0.7277943700298,-31.78224938055));
#21458=CARTESIAN_POINT('Ctrl Pts',(1.260410936535,-0.1023232250025,-31.83749686267));
#21459=CARTESIAN_POINT('Ctrl Pts',(0.9031918799483,-0.8850707304042,-31.8927443448));
#21460=CARTESIAN_POINT('Ctrl Pts',(0.1278440645328,-1.258078549202,-31.94799182692));
#21461=CARTESIAN_POINT('Ctrl Pts',(-0.7066886712758,-1.048664412443,-32.00323930904));
#21462=CARTESIAN_POINT('Ctrl Pts',(-1.214062705292,-0.3537753607434,-32.05848679117));
#21463=CARTESIAN_POINT('Ctrl Pts',(-1.159392542789,0.5048914975012,-32.11373427329));
#21464=CARTESIAN_POINT('Ctrl Pts',(-0.5679833167426,1.129824629341,-32.16898175542));
#21465=CARTESIAN_POINT('Ctrl Pts',(0.2863590197545,1.23169686325,-32.22422923754));
#21466=CARTESIAN_POINT('Ctrl Pts',(1.008178628936,0.7634106326662,-32.27947671967));
#21467=CARTESIAN_POINT('Ctrl Pts',(1.263094839915,-0.05848087125908,-32.33472420179));
#21468=CARTESIAN_POINT('Ctrl Pts',(1.043636050887,-0.5878927540068,-32.37155585654));
#21469=CARTESIAN_POINT('Ctrl Pts',(0.8614506246688,-0.7872497540188,-32.38997168392));
#21470=CARTESIAN_POINT('',(-0.6859379234404,0.9441125563889,-30.50007747308));
#21471=CARTESIAN_POINT('Ctrl Pts',(1.155855903054,0.1607995190315,-28.62357429354));
#21472=CARTESIAN_POINT('Ctrl Pts',(1.195258896894,-0.1224362972325,-28.64307429354));
#21473=CARTESIAN_POINT('Ctrl Pts',(1.056077145856,-0.7175033572827,-28.68207429354));
#21474=CARTESIAN_POINT('Ctrl Pts',(0.3019967923042,-1.240748778247,-28.74057429354));
#21475=CARTESIAN_POINT('Ctrl Pts',(-0.6081163618214,-1.122792874227,-28.79907429354));
#21476=CARTESIAN_POINT('Ctrl Pts',(-1.204114952344,-0.4249855149138,-28.85757429354));
#21477=CARTESIAN_POINT('Ctrl Pts',(-1.178171694542,0.49235784776,-28.91607429354));
#21478=CARTESIAN_POINT('Ctrl Pts',(-0.5436824759227,1.155383851922,-28.97457429354));
#21479=CARTESIAN_POINT('Ctrl Pts',(0.3716274479098,1.221636807823,-29.03307429354));
#21480=CARTESIAN_POINT('Ctrl Pts',(1.094985744155,0.6568937894785,-29.09157429354));
#21481=CARTESIAN_POINT('Ctrl Pts',(1.252765868871,-0.2471455563325,-29.15007429354));
#21482=CARTESIAN_POINT('Ctrl Pts',(0.7634718132616,-1.023530188774,-29.20857429354));
#21483=CARTESIAN_POINT('Ctrl Pts',(-0.1201679976972,-1.271244628134,-29.26707429354));
#21484=CARTESIAN_POINT('Ctrl Pts',(-0.9417390602074,-0.8623403017182,-29.32557429354));
#21485=CARTESIAN_POINT('Ctrl Pts',(-1.276886402343,-0.008023019429936,-29.38407429354));
#21486=CARTESIAN_POINT('Ctrl Pts',(-0.9525009070881,0.850438284238,-29.44257429354));
#21487=CARTESIAN_POINT('Ctrl Pts',(-0.1361330203811,1.269634220587,-29.50107429354));
#21488=CARTESIAN_POINT('Ctrl Pts',(0.7505498113574,1.033043190765,-29.55957429354));
#21489=CARTESIAN_POINT('Ctrl Pts',(1.249561315594,0.262868354685,-29.61807429354));
#21490=CARTESIAN_POINT('Ctrl Pts',(1.103153839379,-0.6430823119665,-29.67657429354));
#21491=CARTESIAN_POINT('Ctrl Pts',(0.3869492533009,-1.216870382867,-29.73507429354));
#21492=CARTESIAN_POINT('Ctrl Pts',(-0.5291209893422,-1.162124878025,-29.79357429354));
#21493=CARTESIAN_POINT('Ctrl Pts',(-1.171891533923,-0.5071227513611,-29.85207429354));
#21494=CARTESIAN_POINT('Ctrl Pts',(-1.209360820682,0.4098166204233,-29.91057429354));
#21495=CARTESIAN_POINT('Ctrl Pts',(-0.6221753352776,1.115078965991,-29.96907429354));
#21496=CARTESIAN_POINT('Ctrl Pts',(0.2863739154552,1.244384671677,-30.02757429354));
#21497=CARTESIAN_POINT('Ctrl Pts',(1.047006449646,0.7309452405402,-30.08607429354));
#21498=CARTESIAN_POINT('Ctrl Pts',(1.266842465797,-0.1600395162514,-30.14457429354));
#21499=CARTESIAN_POINT('Ctrl Pts',(0.8323352153661,-0.9683609251365,-30.20307429354));
#21500=CARTESIAN_POINT('Ctrl Pts',(-0.03209325983472,-1.276509118266,-30.26157429354));
#21501=CARTESIAN_POINT('Ctrl Pts',(-0.8799211891228,-0.9253151078751,-30.32007429354));
#21502=CARTESIAN_POINT('Ctrl Pts',(-1.273344351706,-0.09619644100725,-30.37857429354));
#21503=CARTESIAN_POINT('Ctrl Pts',(-1.008732028848,0.7826683203553,-30.43707429354));
#21504=CARTESIAN_POINT('Ctrl Pts',(-0.485799150132,1.098923865977,-30.47607429354));
#21505=CARTESIAN_POINT('Ctrl Pts',(-0.2042496867001,1.148974072566,-30.49557429354));
#21506=CARTESIAN_POINT('Ctrl Pts',(1.155855903054,0.1607995190315,-28.68906643118));
#21507=CARTESIAN_POINT('Ctrl Pts',(1.195258896894,-0.1224362972325,-28.70856643118));
#21508=CARTESIAN_POINT('Ctrl Pts',(1.056077145856,-0.7175033572827,-28.74756643118));
#21509=CARTESIAN_POINT('Ctrl Pts',(0.3019967923042,-1.240748778247,-28.80606643118));
#21510=CARTESIAN_POINT('Ctrl Pts',(-0.6081163618214,-1.122792874227,-28.86456643118));
#21511=CARTESIAN_POINT('Ctrl Pts',(-1.204114952344,-0.4249855149138,-28.92306643118));
#21512=CARTESIAN_POINT('Ctrl Pts',(-1.178171694542,0.49235784776,-28.98156643118));
#21513=CARTESIAN_POINT('Ctrl Pts',(-0.5436824759227,1.155383851922,-29.04006643118));
#21514=CARTESIAN_POINT('Ctrl Pts',(0.3716274479098,1.221636807823,-29.09856643118));
#21515=CARTESIAN_POINT('Ctrl Pts',(1.094985744155,0.6568937894785,-29.15706643118));
#21516=CARTESIAN_POINT('Ctrl Pts',(1.252765868871,-0.2471455563325,-29.21556643118));
#21517=CARTESIAN_POINT('Ctrl Pts',(0.7634718132616,-1.023530188774,-29.27406643118));
#21518=CARTESIAN_POINT('Ctrl Pts',(-0.1201679976972,-1.271244628134,-29.33256643118));
#21519=CARTESIAN_POINT('Ctrl Pts',(-0.9417390602074,-0.8623403017182,-29.39106643118));
#21520=CARTESIAN_POINT('Ctrl Pts',(-1.276886402343,-0.008023019429936,-29.44956643118));
#21521=CARTESIAN_POINT('Ctrl Pts',(-0.9525009070881,0.850438284238,-29.50806643118));
#21522=CARTESIAN_POINT('Ctrl Pts',(-0.1361330203811,1.269634220587,-29.56656643118));
#21523=CARTESIAN_POINT('Ctrl Pts',(0.7505498113574,1.033043190765,-29.62506643118));
#21524=CARTESIAN_POINT('Ctrl Pts',(1.249561315594,0.262868354685,-29.68356643118));
#21525=CARTESIAN_POINT('Ctrl Pts',(1.103153839379,-0.6430823119665,-29.74206643118));
#21526=CARTESIAN_POINT('Ctrl Pts',(0.3869492533009,-1.216870382867,-29.80056643118));
#21527=CARTESIAN_POINT('Ctrl Pts',(-0.5291209893422,-1.162124878025,-29.85906643118));
#21528=CARTESIAN_POINT('Ctrl Pts',(-1.171891533923,-0.5071227513611,-29.91756643118));
#21529=CARTESIAN_POINT('Ctrl Pts',(-1.209360820682,0.4098166204233,-29.97606643118));
#21530=CARTESIAN_POINT('Ctrl Pts',(-0.6221753352776,1.115078965991,-30.03456643118));
#21531=CARTESIAN_POINT('Ctrl Pts',(0.2863739154552,1.244384671677,-30.09306643118));
#21532=CARTESIAN_POINT('Ctrl Pts',(1.047006449646,0.7309452405402,-30.15156643118));
#21533=CARTESIAN_POINT('Ctrl Pts',(1.266842465797,-0.1600395162514,-30.21006643118));
#21534=CARTESIAN_POINT('Ctrl Pts',(0.8323352153661,-0.9683609251365,-30.26856643118));
#21535=CARTESIAN_POINT('Ctrl Pts',(-0.03209325983472,-1.276509118266,-30.32706643118));
#21536=CARTESIAN_POINT('Ctrl Pts',(-0.8799211891228,-0.9253151078751,-30.38556643118));
#21537=CARTESIAN_POINT('Ctrl Pts',(-1.273344351706,-0.09619644100725,-30.44406643118));
#21538=CARTESIAN_POINT('Ctrl Pts',(-1.008732028848,0.7826683203553,-30.50256643118));
#21539=CARTESIAN_POINT('Ctrl Pts',(-0.485799150132,1.098923865977,-30.54156643118));
#21540=CARTESIAN_POINT('Ctrl Pts',(-0.2042496867001,1.148974072566,-30.56106643118));
#21541=CARTESIAN_POINT('Ctrl Pts',(1.155855903054,0.1607995190315,-28.75455856882));
#21542=CARTESIAN_POINT('Ctrl Pts',(1.195258896894,-0.1224362972325,-28.77405856882));
#21543=CARTESIAN_POINT('Ctrl Pts',(1.056077145856,-0.7175033572827,-28.81305856882));
#21544=CARTESIAN_POINT('Ctrl Pts',(0.3019967923042,-1.240748778247,-28.87155856882));
#21545=CARTESIAN_POINT('Ctrl Pts',(-0.6081163618214,-1.122792874227,-28.93005856882));
#21546=CARTESIAN_POINT('Ctrl Pts',(-1.204114952344,-0.4249855149138,-28.98855856882));
#21547=CARTESIAN_POINT('Ctrl Pts',(-1.178171694542,0.49235784776,-29.04705856882));
#21548=CARTESIAN_POINT('Ctrl Pts',(-0.5436824759227,1.155383851922,-29.10555856882));
#21549=CARTESIAN_POINT('Ctrl Pts',(0.3716274479098,1.221636807823,-29.16405856882));
#21550=CARTESIAN_POINT('Ctrl Pts',(1.094985744155,0.6568937894785,-29.22255856882));
#21551=CARTESIAN_POINT('Ctrl Pts',(1.252765868871,-0.2471455563325,-29.28105856882));
#21552=CARTESIAN_POINT('Ctrl Pts',(0.7634718132616,-1.023530188774,-29.33955856882));
#21553=CARTESIAN_POINT('Ctrl Pts',(-0.1201679976972,-1.271244628134,-29.39805856882));
#21554=CARTESIAN_POINT('Ctrl Pts',(-0.9417390602074,-0.8623403017182,-29.45655856882));
#21555=CARTESIAN_POINT('Ctrl Pts',(-1.276886402343,-0.008023019429936,-29.51505856882));
#21556=CARTESIAN_POINT('Ctrl Pts',(-0.9525009070881,0.850438284238,-29.57355856882));
#21557=CARTESIAN_POINT('Ctrl Pts',(-0.1361330203811,1.269634220587,-29.63205856882));
#21558=CARTESIAN_POINT('Ctrl Pts',(0.7505498113574,1.033043190765,-29.69055856882));
#21559=CARTESIAN_POINT('Ctrl Pts',(1.249561315594,0.262868354685,-29.74905856882));
#21560=CARTESIAN_POINT('Ctrl Pts',(1.103153839379,-0.6430823119665,-29.80755856882));
#21561=CARTESIAN_POINT('Ctrl Pts',(0.3869492533009,-1.216870382867,-29.86605856882));
#21562=CARTESIAN_POINT('Ctrl Pts',(-0.5291209893422,-1.162124878025,-29.92455856882));
#21563=CARTESIAN_POINT('Ctrl Pts',(-1.171891533923,-0.5071227513611,-29.98305856882));
#21564=CARTESIAN_POINT('Ctrl Pts',(-1.209360820682,0.4098166204233,-30.04155856882));
#21565=CARTESIAN_POINT('Ctrl Pts',(-0.6221753352776,1.115078965991,-30.10005856882));
#21566=CARTESIAN_POINT('Ctrl Pts',(0.2863739154552,1.244384671677,-30.15855856882));
#21567=CARTESIAN_POINT('Ctrl Pts',(1.047006449646,0.7309452405402,-30.21705856882));
#21568=CARTESIAN_POINT('Ctrl Pts',(1.266842465797,-0.1600395162514,-30.27555856882));
#21569=CARTESIAN_POINT('Ctrl Pts',(0.8323352153661,-0.9683609251365,-30.33405856882));
#21570=CARTESIAN_POINT('Ctrl Pts',(-0.03209325983472,-1.276509118266,-30.39255856882));
#21571=CARTESIAN_POINT('Ctrl Pts',(-0.8799211891228,-0.9253151078751,-30.45105856882));
#21572=CARTESIAN_POINT('Ctrl Pts',(-1.273344351706,-0.09619644100725,-30.50955856882));
#21573=CARTESIAN_POINT('Ctrl Pts',(-1.008732028848,0.7826683203553,-30.56805856882));
#21574=CARTESIAN_POINT('Ctrl Pts',(-0.485799150132,1.098923865977,-30.60705856882));
#21575=CARTESIAN_POINT('Ctrl Pts',(-0.2042496867001,1.148974072566,-30.62655856882));
#21576=CARTESIAN_POINT('Ctrl Pts',(1.155855903054,0.1607995190315,-28.82005070646));
#21577=CARTESIAN_POINT('Ctrl Pts',(1.195258896894,-0.1224362972325,-28.83955070646));
#21578=CARTESIAN_POINT('Ctrl Pts',(1.056077145856,-0.7175033572827,-28.87855070646));
#21579=CARTESIAN_POINT('Ctrl Pts',(0.3019967923042,-1.240748778247,-28.93705070646));
#21580=CARTESIAN_POINT('Ctrl Pts',(-0.6081163618214,-1.122792874227,-28.99555070646));
#21581=CARTESIAN_POINT('Ctrl Pts',(-1.204114952344,-0.4249855149138,-29.05405070646));
#21582=CARTESIAN_POINT('Ctrl Pts',(-1.178171694542,0.49235784776,-29.11255070646));
#21583=CARTESIAN_POINT('Ctrl Pts',(-0.5436824759227,1.155383851922,-29.17105070646));
#21584=CARTESIAN_POINT('Ctrl Pts',(0.3716274479098,1.221636807823,-29.22955070646));
#21585=CARTESIAN_POINT('Ctrl Pts',(1.094985744155,0.6568937894785,-29.28805070646));
#21586=CARTESIAN_POINT('Ctrl Pts',(1.252765868871,-0.2471455563325,-29.34655070646));
#21587=CARTESIAN_POINT('Ctrl Pts',(0.7634718132616,-1.023530188774,-29.40505070646));
#21588=CARTESIAN_POINT('Ctrl Pts',(-0.1201679976972,-1.271244628134,-29.46355070646));
#21589=CARTESIAN_POINT('Ctrl Pts',(-0.9417390602074,-0.8623403017182,-29.52205070646));
#21590=CARTESIAN_POINT('Ctrl Pts',(-1.276886402343,-0.008023019429936,-29.58055070646));
#21591=CARTESIAN_POINT('Ctrl Pts',(-0.9525009070881,0.850438284238,-29.63905070646));
#21592=CARTESIAN_POINT('Ctrl Pts',(-0.1361330203811,1.269634220587,-29.69755070646));
#21593=CARTESIAN_POINT('Ctrl Pts',(0.7505498113574,1.033043190765,-29.75605070646));
#21594=CARTESIAN_POINT('Ctrl Pts',(1.249561315594,0.262868354685,-29.81455070646));
#21595=CARTESIAN_POINT('Ctrl Pts',(1.103153839379,-0.6430823119665,-29.87305070646));
#21596=CARTESIAN_POINT('Ctrl Pts',(0.3869492533009,-1.216870382867,-29.93155070646));
#21597=CARTESIAN_POINT('Ctrl Pts',(-0.5291209893422,-1.162124878025,-29.99005070646));
#21598=CARTESIAN_POINT('Ctrl Pts',(-1.171891533923,-0.5071227513611,-30.04855070646));
#21599=CARTESIAN_POINT('Ctrl Pts',(-1.209360820682,0.4098166204233,-30.10705070646));
#21600=CARTESIAN_POINT('Ctrl Pts',(-0.6221753352776,1.115078965991,-30.16555070646));
#21601=CARTESIAN_POINT('Ctrl Pts',(0.2863739154552,1.244384671677,-30.22405070646));
#21602=CARTESIAN_POINT('Ctrl Pts',(1.047006449646,0.7309452405402,-30.28255070646));
#21603=CARTESIAN_POINT('Ctrl Pts',(1.266842465797,-0.1600395162514,-30.34105070646));
#21604=CARTESIAN_POINT('Ctrl Pts',(0.8323352153661,-0.9683609251365,-30.39955070646));
#21605=CARTESIAN_POINT('Ctrl Pts',(-0.03209325983472,-1.276509118266,-30.45805070646));
#21606=CARTESIAN_POINT('Ctrl Pts',(-0.8799211891228,-0.9253151078751,-30.51655070646));
#21607=CARTESIAN_POINT('Ctrl Pts',(-1.273344351706,-0.09619644100725,-30.57505070646));
#21608=CARTESIAN_POINT('Ctrl Pts',(-1.008732028848,0.7826683203553,-30.63355070646));
#21609=CARTESIAN_POINT('Ctrl Pts',(-0.485799150132,1.098923865977,-30.67255070646));
#21610=CARTESIAN_POINT('Ctrl Pts',(-0.2042496867001,1.148974072566,-30.69205070646));
#21611=CARTESIAN_POINT('',(1.10987074412979,-0.360618865453563,-28.7000774755696));
#21612=CARTESIAN_POINT('',(1.10987074420186,-0.360618865445946,-28.8155475173803));
#21613=CARTESIAN_POINT('',(1.109870874299,-0.360618907335,-28.70007747308));
#21614=CARTESIAN_POINT('Ctrl Pts',(1.10908833794556,-0.360366944018243,
-28.8155263221856));
#21615=CARTESIAN_POINT('Ctrl Pts',(1.08313436609586,-0.440796138886377,
-28.821289639903));
#21616=CARTESIAN_POINT('Ctrl Pts',(1.04860768641626,-0.518475529758915,
-28.8270583193288));
#21617=CARTESIAN_POINT('Ctrl Pts',(0.962822718320563,-0.665102822246014,
-28.8386648185783));
#21618=CARTESIAN_POINT('Ctrl Pts',(0.911877589687252,-0.732889579139993,
-28.8444246367459));
#21619=CARTESIAN_POINT('Ctrl Pts',(0.749526335843727,-0.906069987879671,
-28.8606247655878));
#21620=CARTESIAN_POINT('Ctrl Pts',(0.622881803069167,-0.997235485886477,
-28.8710522198585));
#21621=CARTESIAN_POINT('Ctrl Pts',(0.343528450555899,-1.12590745534022,
-28.8920310449809));
#21622=CARTESIAN_POINT('Ctrl Pts',(0.194312135562372,-1.16089704614948,
-28.902302863744));
#21623=CARTESIAN_POINT('Ctrl Pts',(-0.111156106659192,-1.17034442347986,
-28.9231468506276));
#21624=CARTESIAN_POINT('Ctrl Pts',(-0.26351142328336,-1.14592402246402,
-28.9334627805694));
#21625=CARTESIAN_POINT('Ctrl Pts',(-0.549326063249744,-1.04113475309189,
-28.9542375650596));
#21626=CARTESIAN_POINT('Ctrl Pts',(-0.677727411883004,-0.962092897939803,
-28.9643397811051));
#21627=CARTESIAN_POINT('Ctrl Pts',(-0.900820166818602,-0.754917089196826,
-28.9850966850868));
#21628=CARTESIAN_POINT('Ctrl Pts',(-0.991430863061421,-0.632184918383142,
-28.9953023673024));
#21629=CARTESIAN_POINT('Ctrl Pts',(-1.13130517516952,-0.337598251088518,
-29.0175666426254));
#21630=CARTESIAN_POINT('Ctrl Pts',(-1.15872514586492,-0.185091355530231,
-29.0279248529793));
#21631=CARTESIAN_POINT('Ctrl Pts',(-1.17156099735629,0.0915106406107147,
-29.0467982047518));
#21632=CARTESIAN_POINT('Ctrl Pts',(-1.15094021376635,0.240868634693148,
-29.0568916601283));
#21633=CARTESIAN_POINT('Ctrl Pts',(-1.04462445846178,0.551227615411852,
-29.079295860188));
#21634=CARTESIAN_POINT('Ctrl Pts',(-0.955273189774736,0.680414508389834,
-29.0897825979082));
#21635=CARTESIAN_POINT('Ctrl Pts',(-0.774838363480179,0.883314838060978,
-29.1082867322753));
#21636=CARTESIAN_POINT('Ctrl Pts',(-0.657401586964177,0.974985736585898,
-29.1182677916964));
#21637=CARTESIAN_POINT('Ctrl Pts',(-0.368344830676665,1.12174076584231,
-29.1404107238409));
#21638=CARTESIAN_POINT('Ctrl Pts',(-0.212531118107411,1.1535440042497,-29.1510273049902));
#21639=CARTESIAN_POINT('Ctrl Pts',(0.0594720124148806,1.17343886176816,
-29.1696126930078));
#21640=CARTESIAN_POINT('Ctrl Pts',(0.206305151023307,1.15779145978757,-29.1795125735436));
#21641=CARTESIAN_POINT('Ctrl Pts',(0.493566643319564,1.06879852693626,-29.2000550606956));
#21642=CARTESIAN_POINT('Ctrl Pts',(0.632274348520006,0.991765068167543,
-29.2106622296585));
#21643=CARTESIAN_POINT('Ctrl Pts',(0.843248468532097,0.814363861741664,
-29.2294473277748));
#21644=CARTESIAN_POINT('Ctrl Pts',(0.946872694845534,0.704265996517519,
-29.2395560462993));
#21645=CARTESIAN_POINT('Ctrl Pts',(1.10143556399852,0.414582166282669,-29.2619812077135));
#21646=CARTESIAN_POINT('Ctrl Pts',(1.14628465443798,0.262803931594675,-29.272558053066));
#21647=CARTESIAN_POINT('Ctrl Pts',(1.17306196823584,-0.0177920846726822,
-29.2917705495727));
#21648=CARTESIAN_POINT('Ctrl Pts',(1.16777374859159,-0.169443851360727,
-29.301923080837));
#21649=CARTESIAN_POINT('Ctrl Pts',(1.07311149596804,-0.482141027412294,
-29.324229282871));
#21650=CARTESIAN_POINT('Ctrl Pts',(0.998645675280905,-0.620862503467565,
-29.3347495650282));
#21651=CARTESIAN_POINT('Ctrl Pts',(0.802434704990753,-0.861103744062571,
-29.3558983763231));
#21652=CARTESIAN_POINT('Ctrl Pts',(0.686156399960789,-0.956092045564658,
-29.3659604824618));
#21653=CARTESIAN_POINT('Ctrl Pts',(0.418179775124533,-1.09915266243817,
-29.3866904752757));
#21654=CARTESIAN_POINT('Ctrl Pts',(0.268798826463745,-1.14470235742467,
-29.3971268139701));
#21655=CARTESIAN_POINT('Ctrl Pts',(-0.0370622684688421,-1.17652270127989,
-29.4181021416964));
#21656=CARTESIAN_POINT('Ctrl Pts',(-0.189446380573865,-1.16172356518029,
-29.4283633413594));
#21657=CARTESIAN_POINT('Ctrl Pts',(-0.48191823722687,-1.07231208588559,
-29.4492232952251));
#21658=CARTESIAN_POINT('Ctrl Pts',(-0.618455614369153,-1.00003027230851,
-29.4595514605357));
#21659=CARTESIAN_POINT('Ctrl Pts',(-0.854289106561804,-0.809574565893422,
-29.4802380394371));
#21660=CARTESIAN_POINT('Ctrl Pts',(-0.950818687642285,-0.693822895932136,
-29.4903371103176));
#21661=CARTESIAN_POINT('Ctrl Pts',(-1.09602778432127,-0.424466988073746,
-29.5112005351714));
#21662=CARTESIAN_POINT('Ctrl Pts',(-1.14228730776674,-0.278868611711132,
-29.5214196096766));
#21663=CARTESIAN_POINT('Ctrl Pts',(-1.17969101994448,0.0449548978083805,
-29.5436737563468));
#21664=CARTESIAN_POINT('Ctrl Pts',(-1.15666344894799,0.197955069125265,
-29.5540179844193));
#21665=CARTESIAN_POINT('Ctrl Pts',(-1.07946856224424,0.464460329139435,
-29.5729300210825));
#21666=CARTESIAN_POINT('Ctrl Pts',(-1.01165109460015,0.599360219704604,
-29.5830368577589));
#21667=CARTESIAN_POINT('Ctrl Pts',(-0.811053751559631,0.858554997261858,
-29.6054191523544));
#21668=CARTESIAN_POINT('Ctrl Pts',(-0.685118451514117,0.951996193221799,
-29.6158902244773));
#21669=CARTESIAN_POINT('Ctrl Pts',(-0.448246304615079,1.08615128492057,
-29.6344423045363));
#21670=CARTESIAN_POINT('Ctrl Pts',(-0.307294849336651,1.1350476484419,-29.6444366233427));
#21671=CARTESIAN_POINT('Ctrl Pts',(0.0292016419244714,1.18278509811256,
-29.667650805626));
#21672=CARTESIAN_POINT('Ctrl Pts',(0.189862921386255,1.15554169754149,-29.6784973022942));
#21673=CARTESIAN_POINT('Ctrl Pts',(0.435078569175385,1.09139610098499,-29.6957700105568));
#21674=CARTESIAN_POINT('Ctrl Pts',(0.568753885931893,1.02925174324196,-29.7056531858431));
#21675=CARTESIAN_POINT('Ctrl Pts',(0.8031219609487,0.858973369535551,-29.7254418679969));
#21676=CARTESIAN_POINT('Ctrl Pts',(0.903532701937408,0.751044251113621,
-29.7353250432866));
#21677=CARTESIAN_POINT('Ctrl Pts',(1.04031459198797,0.53765239083601,-29.7525977515492));
#21678=CARTESIAN_POINT('Ctrl Pts',(1.11587167131851,0.393273107848723,-29.7634442482175));
#21679=CARTESIAN_POINT('Ctrl Pts',(1.17445379308505,0.0584942439088353,
-29.7866584305008));
#21680=CARTESIAN_POINT('Ctrl Pts',(1.17150698299789,-0.090668363406152,
-29.7966527493071));
#21681=CARTESIAN_POINT('Ctrl Pts',(1.11711542772956,-0.357403365460144,
-29.8152048293661));
#21682=CARTESIAN_POINT('Ctrl Pts',(1.06716371732723,-0.506049870726462,
-29.8256759014888));
#21683=CARTESIAN_POINT('Ctrl Pts',(0.882642823167696,-0.776924872095253,
-29.8480581960844));
#21684=CARTESIAN_POINT('Ctrl Pts',(0.77530215321567,-0.883109475340823,
-29.858165032761));
#21685=CARTESIAN_POINT('Ctrl Pts',(0.545695120922613,-1.03888082979983,
-29.8770770694243));
#21686=CARTESIAN_POINT('Ctrl Pts',(0.407299221774572,-1.10806100432971,
-29.8874212974969));
#21687=CARTESIAN_POINT('Ctrl Pts',(0.0877663802010376,-1.17255492774913,
-29.9096754441671));
#21688=CARTESIAN_POINT('Ctrl Pts',(-0.0650008832968393,-1.17355187918509,
-29.9198945186722));
#21689=CARTESIAN_POINT('Ctrl Pts',(-0.366045653279394,-1.1186853746269,
-29.9407579435258));
#21690=CARTESIAN_POINT('Ctrl Pts',(-0.505961314281852,-1.06264952067055,
-29.9508570144062));
#21691=CARTESIAN_POINT('Ctrl Pts',(-0.75997201186392,-0.897212591118086,
-29.9715435933075));
#21692=CARTESIAN_POINT('Ctrl Pts',(-0.870908471580324,-0.78969413764874,
-29.9818717586181));
#21693=CARTESIAN_POINT('Ctrl Pts',(-1.04632261567737,-0.539166539140349,
-30.0027317124838));
#21694=CARTESIAN_POINT('Ctrl Pts',(-1.10748671081373,-0.39881382089982,
-30.0129929121468));
#21695=CARTESIAN_POINT('Ctrl Pts',(-1.17174004169197,-0.0980896064647566,
-30.0339682398731));
#21696=CARTESIAN_POINT('Ctrl Pts',(-1.17458095923193,0.0580557480089826,
-30.0444045785676));
#21697=CARTESIAN_POINT('Ctrl Pts',(-1.12133155849895,0.357124825114059,
-30.0651345713814));
#21698=CARTESIAN_POINT('Ctrl Pts',(-1.06692428771505,0.497065064247616,
-30.0751966775202));
#21699=CARTESIAN_POINT('Ctrl Pts',(-0.899073814666865,0.757911412204312,
-30.0963454888149));
#21700=CARTESIAN_POINT('Ctrl Pts',(-0.790153055006947,0.871599909795869,
-30.106865770972));
#21701=CARTESIAN_POINT('Ctrl Pts',(-0.522012612882802,1.05825780349354,
-30.1291719730058));
#21702=CARTESIAN_POINT('Ctrl Pts',(-0.379417361706689,1.11015017237935,
-30.1393245042701));
#21703=CARTESIAN_POINT('Ctrl Pts',(-0.104280046962064,1.17139237118361,
-30.1585370007769));
#21704=CARTESIAN_POINT('Ctrl Pts',(0.0539287632978188,1.17564040536612,
-30.1691138461296));
#21705=CARTESIAN_POINT('Ctrl Pts',(0.377197010975913,1.11815960801923,-30.1915390075439));
#21706=CARTESIAN_POINT('Ctrl Pts',(0.513927950087521,1.05362922373646,-30.2016477260683));
#21707=CARTESIAN_POINT('Ctrl Pts',(0.747841111914739,0.907800899737522,
-30.2204328241846));
#21708=CARTESIAN_POINT('Ctrl Pts',(0.863967323007234,0.799686680741337,
-30.2310399931474));
#21709=CARTESIAN_POINT('Ctrl Pts',(1.03737331464879,0.553985095242687,-30.2515824802992));
#21710=CARTESIAN_POINT('Ctrl Pts',(1.09762881343296,0.419173795090948,-30.2614823608351));
#21711=CARTESIAN_POINT('Ctrl Pts',(1.16276126940395,0.154335596280972,-30.2800677488528));
#21712=CARTESIAN_POINT('Ctrl Pts',(1.18066367741776,-0.00367979153002535,
-30.2906843300022));
#21713=CARTESIAN_POINT('Ctrl Pts',(1.13041480057629,-0.323938901225899,
-30.3128272621468));
#21714=CARTESIAN_POINT('Ctrl Pts',(1.0795205548877,-0.463955778317749,-30.322808321568));
#21715=CARTESIAN_POINT('Ctrl Pts',(0.942308301897849,-0.69825914566429,
-30.3413124559352));
#21716=CARTESIAN_POINT('Ctrl Pts',(0.847055326004481,-0.823158197369145,
-30.3517991936555));
#21717=CARTESIAN_POINT('Ctrl Pts',(0.584739770160091,-1.02017668863557,
-30.3742033937154));
#21718=CARTESIAN_POINT('Ctrl Pts',(0.449064049193805,-1.0859423776572,-30.3842968490918));
#21719=CARTESIAN_POINT('Ctrl Pts',(0.18203342209547,-1.15920947493991,-30.4031702008643));
#21720=CARTESIAN_POINT('Ctrl Pts',(0.0285175083645084,-1.18025875562043,
-30.4135284112181));
#21721=CARTESIAN_POINT('Ctrl Pts',(-0.294874600697855,-1.13826266613818,
-30.4357926865411));
#21722=CARTESIAN_POINT('Ctrl Pts',(-0.439600076520489,-1.09001309956844,
-30.4459983687568));
#21723=CARTESIAN_POINT('Ctrl Pts',(-0.705575432041411,-0.941860126973679,
-30.4667552727384));
#21724=CARTESIAN_POINT('Ctrl Pts',(-0.820426902272153,-0.844168464163867,
-30.476857488784));
#21725=CARTESIAN_POINT('Ctrl Pts',(-1.00840900073706,-0.604724253435626,
-30.4976322732741));
#21726=CARTESIAN_POINT('Ctrl Pts',(-1.07871456427402,-0.467372055691353,
-30.5079482032156));
#21727=CARTESIAN_POINT('Ctrl Pts',(-1.16412445259043,-0.173935093258025,
-30.5287921900991));
#21728=CARTESIAN_POINT('Ctrl Pts',(-1.17695775141982,-0.0212095663596859,
-30.5390640088622));
#21729=CARTESIAN_POINT('Ctrl Pts',(-1.14090836976859,0.284233085157646,
-30.5600428339846));
#21730=CARTESIAN_POINT('Ctrl Pts',(-1.0933401417,0.432850881490686,-30.5704702882553));
#21731=CARTESIAN_POINT('Ctrl Pts',(-0.978811929812615,0.64075935756687,
-30.586669448521));
#21732=CARTESIAN_POINT('Ctrl Pts',(-0.930095050179522,0.710147925105241,
-30.5924283383721));
#21733=CARTESIAN_POINT('Ctrl Pts',(-0.817158328342888,0.837048290513652,
-30.6040347961641));
#21734=CARTESIAN_POINT('Ctrl Pts',(-0.753940956291978,0.893899707069815,
-30.6098044000168));
#21735=CARTESIAN_POINT('Ctrl Pts',(-0.685457562470264,0.943445394325056,
-30.6155686401302));
#21736=CARTESIAN_POINT('Ctrl Pts',(1.10908828377812,-0.360367111878588,
-28.7000562803704));
#21737=CARTESIAN_POINT('Ctrl Pts',(1.08313431805632,-0.440796246967518,
-28.705819594086));
#21738=CARTESIAN_POINT('Ctrl Pts',(1.04860765672726,-0.518475580504724,
-28.7115882695023));
#21739=CARTESIAN_POINT('Ctrl Pts',(0.96282271832024,-0.665102822246447,
-28.7231947647351));
#21740=CARTESIAN_POINT('Ctrl Pts',(0.91187758968706,-0.7328895791402,-28.7289545829027));
#21741=CARTESIAN_POINT('Ctrl Pts',(0.749526335843715,-0.90606998787968,
-28.7451547117448));
#21742=CARTESIAN_POINT('Ctrl Pts',(0.622881803069154,-0.997235485886485,
-28.7555821660155));
#21743=CARTESIAN_POINT('Ctrl Pts',(0.343528450555896,-1.12590745534022,
-28.7765609911379));
#21744=CARTESIAN_POINT('Ctrl Pts',(0.194312135562378,-1.16089704614948,
-28.7868328099008));
#21745=CARTESIAN_POINT('Ctrl Pts',(-0.111156106659175,-1.17034442347986,
-28.8076767967842));
#21746=CARTESIAN_POINT('Ctrl Pts',(-0.263511423283337,-1.14592402246402,
-28.8179927267257));
#21747=CARTESIAN_POINT('Ctrl Pts',(-0.549326063249702,-1.04113475309191,
-28.8387675112157));
#21748=CARTESIAN_POINT('Ctrl Pts',(-0.677727411882962,-0.962092897939833,
-28.8488697272613));
#21749=CARTESIAN_POINT('Ctrl Pts',(-0.900820166818571,-0.754917089196863,
-28.8696266312429));
#21750=CARTESIAN_POINT('Ctrl Pts',(-0.991430863061393,-0.632184918383185,
-28.8798323134585));
#21751=CARTESIAN_POINT('Ctrl Pts',(-1.13130517516951,-0.337598251088571,
-28.9020965887813));
#21752=CARTESIAN_POINT('Ctrl Pts',(-1.15872514586491,-0.185091355530289,
-28.9124547991351));
#21753=CARTESIAN_POINT('Ctrl Pts',(-1.17156099735629,0.091510640610664,
-28.9313281509076));
#21754=CARTESIAN_POINT('Ctrl Pts',(-1.15094021376636,0.240868634693107,
-28.9414216062841));
#21755=CARTESIAN_POINT('Ctrl Pts',(-1.0446244584618,0.551227615411831,-28.9638258063441));
#21756=CARTESIAN_POINT('Ctrl Pts',(-0.955273189774745,0.680414508389824,
-28.9743125440646));
#21757=CARTESIAN_POINT('Ctrl Pts',(-0.774838363480177,0.883314838060981,
-28.992816678432));
#21758=CARTESIAN_POINT('Ctrl Pts',(-0.657401586964166,0.974985736585907,
-29.0027977378534));
#21759=CARTESIAN_POINT('Ctrl Pts',(-0.36834483067665,1.12174076584231,-29.0249406699982));
#21760=CARTESIAN_POINT('Ctrl Pts',(-0.21253111810739,1.1535440042497,-29.0355572511477));
#21761=CARTESIAN_POINT('Ctrl Pts',(0.0594720124149227,1.17343886176816,
-29.0541426391653));
#21762=CARTESIAN_POINT('Ctrl Pts',(0.206305151023344,1.15779145978756,-29.0640425197011));
#21763=CARTESIAN_POINT('Ctrl Pts',(0.493566643319589,1.06879852693625,-29.0845850068529));
#21764=CARTESIAN_POINT('Ctrl Pts',(0.632274348520021,0.991765068167532,
-29.0951921758155));
#21765=CARTESIAN_POINT('Ctrl Pts',(0.843248468532104,0.814363861741656,
-29.1139772739316));
#21766=CARTESIAN_POINT('Ctrl Pts',(0.946872694845539,0.704265996517511,
-29.1240859924559));
#21767=CARTESIAN_POINT('Ctrl Pts',(1.10143556399853,0.414582166282656,-29.1465111538702));
#21768=CARTESIAN_POINT('Ctrl Pts',(1.14628465443799,0.262803931594657,-29.1570879992228));
#21769=CARTESIAN_POINT('Ctrl Pts',(1.17306196823584,-0.0177920846726962,
-29.1763004957296));
#21770=CARTESIAN_POINT('Ctrl Pts',(1.16777374859159,-0.169443851360738,
-29.186453026994));
#21771=CARTESIAN_POINT('Ctrl Pts',(1.07311149596803,-0.482141027412298,
-29.2087592290279));
#21772=CARTESIAN_POINT('Ctrl Pts',(0.998645675280905,-0.620862503467564,
-29.219279511185));
#21773=CARTESIAN_POINT('Ctrl Pts',(0.802434704990756,-0.861103744062567,
-29.2404283224797));
#21774=CARTESIAN_POINT('Ctrl Pts',(0.686156399960795,-0.956092045564654,
-29.2504904286183));
#21775=CARTESIAN_POINT('Ctrl Pts',(0.418179775124541,-1.09915266243817,
-29.2712204214321));
#21776=CARTESIAN_POINT('Ctrl Pts',(0.268798826463751,-1.14470235742467,
-29.2816567601266));
#21777=CARTESIAN_POINT('Ctrl Pts',(-0.0370622684688349,-1.17652270127989,
-29.3026320878529));
#21778=CARTESIAN_POINT('Ctrl Pts',(-0.189446380573858,-1.16172356518029,
-29.312893287516));
#21779=CARTESIAN_POINT('Ctrl Pts',(-0.481918237226863,-1.0723120858856,
-29.3337532413817));
#21780=CARTESIAN_POINT('Ctrl Pts',(-0.618455614369146,-1.00003027230852,
-29.3440814066923));
#21781=CARTESIAN_POINT('Ctrl Pts',(-0.854289106561791,-0.809574565893434,
-29.3647679855936));
#21782=CARTESIAN_POINT('Ctrl Pts',(-0.950818687642273,-0.693822895932154,
-29.374867056474));
#21783=CARTESIAN_POINT('Ctrl Pts',(-1.09602778432126,-0.424466988073762,
-29.3957304813277));
#21784=CARTESIAN_POINT('Ctrl Pts',(-1.14228730776674,-0.27886861171115,
-29.4059495558328));
#21785=CARTESIAN_POINT('Ctrl Pts',(-1.17969101994449,0.044954897808365,
-29.428203702503));
#21786=CARTESIAN_POINT('Ctrl Pts',(-1.15666344894799,0.197955069125252,
-29.4385479305756));
#21787=CARTESIAN_POINT('Ctrl Pts',(-1.07946856224424,0.464460329139423,
-29.4574599672389));
#21788=CARTESIAN_POINT('Ctrl Pts',(-1.01165109460016,0.599360219704595,
-29.4675668039155));
#21789=CARTESIAN_POINT('Ctrl Pts',(-0.811053751559636,0.858554997261854,
-29.4899490985111));
#21790=CARTESIAN_POINT('Ctrl Pts',(-0.685118451514121,0.951996193221797,
-29.5004201706339));
#21791=CARTESIAN_POINT('Ctrl Pts',(-0.448246304615079,1.08615128492057,
-29.5189722506929));
#21792=CARTESIAN_POINT('Ctrl Pts',(-0.307294849336651,1.1350476484419,-29.5289665694992));
#21793=CARTESIAN_POINT('Ctrl Pts',(0.0292016419244812,1.18278509811256,
-29.5521807517825));
#21794=CARTESIAN_POINT('Ctrl Pts',(0.189862921386267,1.15554169754148,-29.5630272484508));
#21795=CARTESIAN_POINT('Ctrl Pts',(0.435078569175386,1.09139610098499,-29.5802999567135));
#21796=CARTESIAN_POINT('Ctrl Pts',(0.568753885931894,1.02925174324196,-29.5901831320031));
#21797=CARTESIAN_POINT('Ctrl Pts',(0.803121960948698,0.858973369535553,
-29.6099718141569));
#21798=CARTESIAN_POINT('Ctrl Pts',(0.903532701937406,0.751044251113624,
-29.6198549894432));
#21799=CARTESIAN_POINT('Ctrl Pts',(1.04031459198799,0.537652390835985,-29.6371276977058));
#21800=CARTESIAN_POINT('Ctrl Pts',(1.11587167131852,0.393273107848698,-29.647974194374));
#21801=CARTESIAN_POINT('Ctrl Pts',(1.17445379308505,0.0584942439088389,
-29.6711883766573));
#21802=CARTESIAN_POINT('Ctrl Pts',(1.17150698299789,-0.0906683634061496,
-29.6811826954637));
#21803=CARTESIAN_POINT('Ctrl Pts',(1.11711542772956,-0.357403365460141,
-29.6997347755227));
#21804=CARTESIAN_POINT('Ctrl Pts',(1.06716371732723,-0.506049870726459,
-29.7102058476456));
#21805=CARTESIAN_POINT('Ctrl Pts',(0.882642823167698,-0.776924872095252,
-29.7325881422412));
#21806=CARTESIAN_POINT('Ctrl Pts',(0.775302153215673,-0.883109475340821,
-29.7426949789176));
#21807=CARTESIAN_POINT('Ctrl Pts',(0.545695120922612,-1.03888082979983,
-29.7616070155808));
#21808=CARTESIAN_POINT('Ctrl Pts',(0.407299221774572,-1.10806100432971,
-29.7719512436533));
#21809=CARTESIAN_POINT('Ctrl Pts',(0.0877663802010367,-1.17255492774913,
-29.7942053903235));
#21810=CARTESIAN_POINT('Ctrl Pts',(-0.0650008832968425,-1.17355187918509,
-29.8044244648287));
#21811=CARTESIAN_POINT('Ctrl Pts',(-0.366045653279393,-1.1186853746269,
-29.8252878896825));
#21812=CARTESIAN_POINT('Ctrl Pts',(-0.505961314281856,-1.06264952067055,
-29.835386960563));
#21813=CARTESIAN_POINT('Ctrl Pts',(-0.759972011863936,-0.897212591118072,
-29.8560735394644));
#21814=CARTESIAN_POINT('Ctrl Pts',(-0.870908471580342,-0.789694137648721,
-29.866401704775));
#21815=CARTESIAN_POINT('Ctrl Pts',(-1.04632261567739,-0.539166539140322,
-29.8872616586407));
#21816=CARTESIAN_POINT('Ctrl Pts',(-1.10748671081375,-0.398813820899789,
-29.8975228583038));
#21817=CARTESIAN_POINT('Ctrl Pts',(-1.17174004169197,-0.0980896064647195,
-29.9184981860302));
#21818=CARTESIAN_POINT('Ctrl Pts',(-1.17458095923193,0.0580557480090229,
-29.9289345247246));
#21819=CARTESIAN_POINT('Ctrl Pts',(-1.12133155849894,0.357124825114116,
-29.9496645175385));
#21820=CARTESIAN_POINT('Ctrl Pts',(-1.06692428771502,0.497065064247667,
-29.9597266236771));
#21821=CARTESIAN_POINT('Ctrl Pts',(-0.899073814666838,0.757911412204344,
-29.9808754349719));
#21822=CARTESIAN_POINT('Ctrl Pts',(-0.790153055006915,0.871599909795898,
-29.9913957171291));
#21823=CARTESIAN_POINT('Ctrl Pts',(-0.522012612882761,1.05825780349356,
-30.0137019191631));
#21824=CARTESIAN_POINT('Ctrl Pts',(-0.379417361706643,1.11015017237937,
-30.0238544504275));
#21825=CARTESIAN_POINT('Ctrl Pts',(-0.104280046962013,1.17139237118361,
-30.0430669469342));
#21826=CARTESIAN_POINT('Ctrl Pts',(0.0539287632978684,1.17564040536612,
-30.0536437922867));
#21827=CARTESIAN_POINT('Ctrl Pts',(0.377197010975957,1.11815960801922,-30.0760689537009));
#21828=CARTESIAN_POINT('Ctrl Pts',(0.513927950087557,1.05362922373644,-30.0861776722252));
#21829=CARTESIAN_POINT('Ctrl Pts',(0.747841111914757,0.907800899737507,
-30.1049627703414));
#21830=CARTESIAN_POINT('Ctrl Pts',(0.863967323007248,0.799686680741322,
-30.1155699393042));
#21831=CARTESIAN_POINT('Ctrl Pts',(1.0373733146488,0.553985095242675,-30.136112426456));
#21832=CARTESIAN_POINT('Ctrl Pts',(1.09762881343296,0.419173795090939,-30.1460123069918));
#21833=CARTESIAN_POINT('Ctrl Pts',(1.16276126940395,0.154335596280958,-30.1645976950093));
#21834=CARTESIAN_POINT('Ctrl Pts',(1.18066367741776,-0.00367979153003583,
-30.1752142761586));
#21835=CARTESIAN_POINT('Ctrl Pts',(1.13041480057629,-0.3239389012259,-30.1973572083032));
#21836=CARTESIAN_POINT('Ctrl Pts',(1.0795205548877,-0.463955778317747,-30.2073382677245));
#21837=CARTESIAN_POINT('Ctrl Pts',(0.94230830189785,-0.69825914566429,-30.2258424020917));
#21838=CARTESIAN_POINT('Ctrl Pts',(0.847055326004478,-0.823158197369149,
-30.2363291398121));
#21839=CARTESIAN_POINT('Ctrl Pts',(0.58473977016008,-1.02017668863558,-30.2587333398721));
#21840=CARTESIAN_POINT('Ctrl Pts',(0.449064049193789,-1.0859423776572,-30.2688267952486));
#21841=CARTESIAN_POINT('Ctrl Pts',(0.182033422095448,-1.15920947493991,
-30.2877001470212));
#21842=CARTESIAN_POINT('Ctrl Pts',(0.0285175083644867,-1.18025875562043,
-30.2980583573751));
#21843=CARTESIAN_POINT('Ctrl Pts',(-0.294874600697877,-1.13826266613818,
-30.320322632698));
#21844=CARTESIAN_POINT('Ctrl Pts',(-0.439600076520509,-1.09001309956843,
-30.3305283149136));
#21845=CARTESIAN_POINT('Ctrl Pts',(-0.705575432041423,-0.941860126973669,
-30.3512852188952));
#21846=CARTESIAN_POINT('Ctrl Pts',(-0.820426902272163,-0.844168464163858,
-30.3613874349407));
#21847=CARTESIAN_POINT('Ctrl Pts',(-1.00840900073707,-0.604724253435611,
-30.3821622194308));
#21848=CARTESIAN_POINT('Ctrl Pts',(-1.07871456427403,-0.467372055691335,
-30.3924781493725));
#21849=CARTESIAN_POINT('Ctrl Pts',(-1.16412445259044,-0.173935093258004,
-30.413322136256));
#21850=CARTESIAN_POINT('Ctrl Pts',(-1.17695775141982,-0.0212095663596662,
-30.423593955019));
#21851=CARTESIAN_POINT('Ctrl Pts',(-1.14090836976858,0.284233085157663,
-30.4445727801414));
#21852=CARTESIAN_POINT('Ctrl Pts',(-1.09334014169999,0.432850881490699,
-30.455000234412));
#21853=CARTESIAN_POINT('Ctrl Pts',(-0.978811871527169,0.640759463375194,
-30.4711994029217));
#21854=CARTESIAN_POINT('Ctrl Pts',(-0.930094913191883,0.710148119341155,
-30.4769583006743));
#21855=CARTESIAN_POINT('Ctrl Pts',(-0.817158075588233,0.837048534600839,
-30.4885647662489));
#21856=CARTESIAN_POINT('Ctrl Pts',(-0.753940691570741,0.893899928191477,
-30.49433436965));
#21857=CARTESIAN_POINT('Ctrl Pts',(-0.685457288884346,0.943445592256226,
-30.5000986093145));
#21858=CARTESIAN_POINT('Ctrl Pts',(-0.8405914827566,-0.809484597174,-26.82357429354));
#21859=CARTESIAN_POINT('Ctrl Pts',(-1.038951010123,-0.603502507076,-26.84307429354));
#21860=CARTESIAN_POINT('Ctrl Pts',(-1.27612225025,-0.0402741620545,-26.88207429354));
#21861=CARTESIAN_POINT('Ctrl Pts',(-0.9736143708746,0.8262775865961,-26.94057429354));
#21862=CARTESIAN_POINT('Ctrl Pts',(-0.1679846215786,1.265800345569,-26.99907429354));
#21863=CARTESIAN_POINT('Ctrl Pts',(0.7243492415226,1.051581514981,-27.05757429354));
#21864=CARTESIAN_POINT('Ctrl Pts',(1.242561604939,0.2941860805683,-27.11607429354));
#21865=CARTESIAN_POINT('Ctrl Pts',(1.118965951462,-0.6151566299544,-27.17457429354));
#21866=CARTESIAN_POINT('Ctrl Pts',(0.4174071783611,-1.206762071712,-27.23307429354));
#21867=CARTESIAN_POINT('Ctrl Pts',(-0.4997495938417,-1.175054711072,-27.29157429354));
#21868=CARTESIAN_POINT('Ctrl Pts',(-1.158777391072,-0.5364123471407,-27.35007429354));
#21869=CARTESIAN_POINT('Ctrl Pts',(-1.219277621892,0.3792958445976,-27.40857429354));
#21870=CARTESIAN_POINT('Ctrl Pts',(-0.6500008921559,1.099091485012,-27.46707429354));
#21871=CARTESIAN_POINT('Ctrl Pts',(0.2550119921671,1.251188290122,-27.52557429354));
#21872=CARTESIAN_POINT('Ctrl Pts',(1.028306986882,0.7570257552148,-27.58407429354));
#21873=CARTESIAN_POINT('Ctrl Pts',(1.270464502452,-0.128153038634,-27.64257429354));
#21874=CARTESIAN_POINT('Ctrl Pts',(0.8564061976507,-0.9471386793648,-27.70107429354));
#21875=CARTESIAN_POINT('Ctrl Pts',(0.,-1.276911607479,-27.75957429354));
#21876=CARTESIAN_POINT('Ctrl Pts',(-0.8564061976507,-0.9471386793648,-27.81807429354));
#21877=CARTESIAN_POINT('Ctrl Pts',(-1.270464502452,-0.128153038634,-27.87657429354));
#21878=CARTESIAN_POINT('Ctrl Pts',(-1.028306986882,0.7570257552148,-27.93507429354));
#21879=CARTESIAN_POINT('Ctrl Pts',(-0.2550119921671,1.251188290122,-27.99357429354));
#21880=CARTESIAN_POINT('Ctrl Pts',(0.6500008921559,1.099091485012,-28.05207429354));
#21881=CARTESIAN_POINT('Ctrl Pts',(1.219277621892,0.3792958445976,-28.11057429354));
#21882=CARTESIAN_POINT('Ctrl Pts',(1.158777391072,-0.5364123471407,-28.16907429354));
#21883=CARTESIAN_POINT('Ctrl Pts',(0.4997495938416,-1.175054711072,-28.22757429354));
#21884=CARTESIAN_POINT('Ctrl Pts',(-0.4174071783611,-1.206762071712,-28.28607429354));
#21885=CARTESIAN_POINT('Ctrl Pts',(-1.118965951462,-0.6151566299543,-28.34457429354));
#21886=CARTESIAN_POINT('Ctrl Pts',(-1.242561604939,0.2941860805683,-28.40307429354));
#21887=CARTESIAN_POINT('Ctrl Pts',(-0.7243492415226,1.051581514981,-28.46157429354));
#21888=CARTESIAN_POINT('Ctrl Pts',(0.1679846215786,1.265800345569,-28.52007429354));
#21889=CARTESIAN_POINT('Ctrl Pts',(0.9736143708746,0.8262775865961,-28.57857429354));
#21890=CARTESIAN_POINT('Ctrl Pts',(1.27612225025,-0.04027416205452,-28.63707429354));
#21891=CARTESIAN_POINT('Ctrl Pts',(1.038951010123,-0.603502507076,-28.67607429354));
#21892=CARTESIAN_POINT('Ctrl Pts',(0.8405914827566,-0.809484597174,-28.69557429354));
#21893=CARTESIAN_POINT('Ctrl Pts',(-0.8405914827566,-0.809484597174,-26.88906643118));
#21894=CARTESIAN_POINT('Ctrl Pts',(-1.038951010123,-0.603502507076,-26.90856643118));
#21895=CARTESIAN_POINT('Ctrl Pts',(-1.27612225025,-0.0402741620545,-26.94756643118));
#21896=CARTESIAN_POINT('Ctrl Pts',(-0.9736143708746,0.8262775865961,-27.00606643118));
#21897=CARTESIAN_POINT('Ctrl Pts',(-0.1679846215786,1.265800345569,-27.06456643118));
#21898=CARTESIAN_POINT('Ctrl Pts',(0.7243492415226,1.051581514981,-27.12306643118));
#21899=CARTESIAN_POINT('Ctrl Pts',(1.242561604939,0.2941860805683,-27.18156643118));
#21900=CARTESIAN_POINT('Ctrl Pts',(1.118965951462,-0.6151566299544,-27.24006643118));
#21901=CARTESIAN_POINT('Ctrl Pts',(0.4174071783611,-1.206762071712,-27.29856643118));
#21902=CARTESIAN_POINT('Ctrl Pts',(-0.4997495938417,-1.175054711072,-27.35706643118));
#21903=CARTESIAN_POINT('Ctrl Pts',(-1.158777391072,-0.5364123471407,-27.41556643118));
#21904=CARTESIAN_POINT('Ctrl Pts',(-1.219277621892,0.3792958445976,-27.47406643118));
#21905=CARTESIAN_POINT('Ctrl Pts',(-0.6500008921559,1.099091485012,-27.53256643118));
#21906=CARTESIAN_POINT('Ctrl Pts',(0.2550119921671,1.251188290122,-27.59106643118));
#21907=CARTESIAN_POINT('Ctrl Pts',(1.028306986882,0.7570257552148,-27.64956643118));
#21908=CARTESIAN_POINT('Ctrl Pts',(1.270464502452,-0.128153038634,-27.70806643118));
#21909=CARTESIAN_POINT('Ctrl Pts',(0.8564061976507,-0.9471386793648,-27.76656643118));
#21910=CARTESIAN_POINT('Ctrl Pts',(0.,-1.276911607479,-27.82506643118));
#21911=CARTESIAN_POINT('Ctrl Pts',(-0.8564061976507,-0.9471386793648,-27.88356643118));
#21912=CARTESIAN_POINT('Ctrl Pts',(-1.270464502452,-0.128153038634,-27.94206643118));
#21913=CARTESIAN_POINT('Ctrl Pts',(-1.028306986882,0.7570257552148,-28.00056643118));
#21914=CARTESIAN_POINT('Ctrl Pts',(-0.2550119921671,1.251188290122,-28.05906643118));
#21915=CARTESIAN_POINT('Ctrl Pts',(0.6500008921559,1.099091485012,-28.11756643118));
#21916=CARTESIAN_POINT('Ctrl Pts',(1.219277621892,0.3792958445976,-28.17606643118));
#21917=CARTESIAN_POINT('Ctrl Pts',(1.158777391072,-0.5364123471407,-28.23456643118));
#21918=CARTESIAN_POINT('Ctrl Pts',(0.4997495938416,-1.175054711072,-28.29306643118));
#21919=CARTESIAN_POINT('Ctrl Pts',(-0.4174071783611,-1.206762071712,-28.35156643118));
#21920=CARTESIAN_POINT('Ctrl Pts',(-1.118965951462,-0.6151566299543,-28.41006643118));
#21921=CARTESIAN_POINT('Ctrl Pts',(-1.242561604939,0.2941860805683,-28.46856643118));
#21922=CARTESIAN_POINT('Ctrl Pts',(-0.7243492415226,1.051581514981,-28.52706643118));
#21923=CARTESIAN_POINT('Ctrl Pts',(0.1679846215786,1.265800345569,-28.58556643118));
#21924=CARTESIAN_POINT('Ctrl Pts',(0.9736143708746,0.8262775865961,-28.64406643118));
#21925=CARTESIAN_POINT('Ctrl Pts',(1.27612225025,-0.04027416205452,-28.70256643118));
#21926=CARTESIAN_POINT('Ctrl Pts',(1.038951010123,-0.603502507076,-28.74156643118));
#21927=CARTESIAN_POINT('Ctrl Pts',(0.8405914827566,-0.809484597174,-28.76106643118));
#21928=CARTESIAN_POINT('Ctrl Pts',(-0.8405914827566,-0.809484597174,-26.95455856882));
#21929=CARTESIAN_POINT('Ctrl Pts',(-1.038951010123,-0.603502507076,-26.97405856882));
#21930=CARTESIAN_POINT('Ctrl Pts',(-1.27612225025,-0.0402741620545,-27.01305856882));
#21931=CARTESIAN_POINT('Ctrl Pts',(-0.9736143708746,0.8262775865961,-27.07155856882));
#21932=CARTESIAN_POINT('Ctrl Pts',(-0.1679846215786,1.265800345569,-27.13005856882));
#21933=CARTESIAN_POINT('Ctrl Pts',(0.7243492415226,1.051581514981,-27.18855856882));
#21934=CARTESIAN_POINT('Ctrl Pts',(1.242561604939,0.2941860805683,-27.24705856882));
#21935=CARTESIAN_POINT('Ctrl Pts',(1.118965951462,-0.6151566299544,-27.30555856882));
#21936=CARTESIAN_POINT('Ctrl Pts',(0.4174071783611,-1.206762071712,-27.36405856882));
#21937=CARTESIAN_POINT('Ctrl Pts',(-0.4997495938417,-1.175054711072,-27.42255856882));
#21938=CARTESIAN_POINT('Ctrl Pts',(-1.158777391072,-0.5364123471407,-27.48105856882));
#21939=CARTESIAN_POINT('Ctrl Pts',(-1.219277621892,0.3792958445976,-27.53955856882));
#21940=CARTESIAN_POINT('Ctrl Pts',(-0.6500008921559,1.099091485012,-27.59805856882));
#21941=CARTESIAN_POINT('Ctrl Pts',(0.2550119921671,1.251188290122,-27.65655856882));
#21942=CARTESIAN_POINT('Ctrl Pts',(1.028306986882,0.7570257552148,-27.71505856882));
#21943=CARTESIAN_POINT('Ctrl Pts',(1.270464502452,-0.128153038634,-27.77355856882));
#21944=CARTESIAN_POINT('Ctrl Pts',(0.8564061976507,-0.9471386793648,-27.83205856882));
#21945=CARTESIAN_POINT('Ctrl Pts',(0.,-1.276911607479,-27.89055856882));
#21946=CARTESIAN_POINT('Ctrl Pts',(-0.8564061976507,-0.9471386793648,-27.94905856882));
#21947=CARTESIAN_POINT('Ctrl Pts',(-1.270464502452,-0.128153038634,-28.00755856882));
#21948=CARTESIAN_POINT('Ctrl Pts',(-1.028306986882,0.7570257552148,-28.06605856882));
#21949=CARTESIAN_POINT('Ctrl Pts',(-0.2550119921671,1.251188290122,-28.12455856882));
#21950=CARTESIAN_POINT('Ctrl Pts',(0.6500008921559,1.099091485012,-28.18305856882));
#21951=CARTESIAN_POINT('Ctrl Pts',(1.219277621892,0.3792958445976,-28.24155856882));
#21952=CARTESIAN_POINT('Ctrl Pts',(1.158777391072,-0.5364123471407,-28.30005856882));
#21953=CARTESIAN_POINT('Ctrl Pts',(0.4997495938416,-1.175054711072,-28.35855856882));
#21954=CARTESIAN_POINT('Ctrl Pts',(-0.4174071783611,-1.206762071712,-28.41705856882));
#21955=CARTESIAN_POINT('Ctrl Pts',(-1.118965951462,-0.6151566299543,-28.47555856882));
#21956=CARTESIAN_POINT('Ctrl Pts',(-1.242561604939,0.2941860805683,-28.53405856882));
#21957=CARTESIAN_POINT('Ctrl Pts',(-0.7243492415226,1.051581514981,-28.59255856882));
#21958=CARTESIAN_POINT('Ctrl Pts',(0.1679846215786,1.265800345569,-28.65105856882));
#21959=CARTESIAN_POINT('Ctrl Pts',(0.9736143708746,0.8262775865961,-28.70955856882));
#21960=CARTESIAN_POINT('Ctrl Pts',(1.27612225025,-0.04027416205452,-28.76805856882));
#21961=CARTESIAN_POINT('Ctrl Pts',(1.038951010123,-0.603502507076,-28.80705856882));
#21962=CARTESIAN_POINT('Ctrl Pts',(0.8405914827566,-0.809484597174,-28.82655856882));
#21963=CARTESIAN_POINT('Ctrl Pts',(-0.8405914827566,-0.809484597174,-27.02005070646));
#21964=CARTESIAN_POINT('Ctrl Pts',(-1.038951010123,-0.603502507076,-27.03955070646));
#21965=CARTESIAN_POINT('Ctrl Pts',(-1.27612225025,-0.0402741620545,-27.07855070646));
#21966=CARTESIAN_POINT('Ctrl Pts',(-0.9736143708746,0.8262775865961,-27.13705070646));
#21967=CARTESIAN_POINT('Ctrl Pts',(-0.1679846215786,1.265800345569,-27.19555070646));
#21968=CARTESIAN_POINT('Ctrl Pts',(0.7243492415226,1.051581514981,-27.25405070646));
#21969=CARTESIAN_POINT('Ctrl Pts',(1.242561604939,0.2941860805683,-27.31255070646));
#21970=CARTESIAN_POINT('Ctrl Pts',(1.118965951462,-0.6151566299544,-27.37105070646));
#21971=CARTESIAN_POINT('Ctrl Pts',(0.4174071783611,-1.206762071712,-27.42955070646));
#21972=CARTESIAN_POINT('Ctrl Pts',(-0.4997495938417,-1.175054711072,-27.48805070646));
#21973=CARTESIAN_POINT('Ctrl Pts',(-1.158777391072,-0.5364123471407,-27.54655070646));
#21974=CARTESIAN_POINT('Ctrl Pts',(-1.219277621892,0.3792958445976,-27.60505070646));
#21975=CARTESIAN_POINT('Ctrl Pts',(-0.6500008921559,1.099091485012,-27.66355070646));
#21976=CARTESIAN_POINT('Ctrl Pts',(0.2550119921671,1.251188290122,-27.72205070646));
#21977=CARTESIAN_POINT('Ctrl Pts',(1.028306986882,0.7570257552148,-27.78055070646));
#21978=CARTESIAN_POINT('Ctrl Pts',(1.270464502452,-0.128153038634,-27.83905070646));
#21979=CARTESIAN_POINT('Ctrl Pts',(0.8564061976507,-0.9471386793648,-27.89755070646));
#21980=CARTESIAN_POINT('Ctrl Pts',(0.,-1.276911607479,-27.95605070646));
#21981=CARTESIAN_POINT('Ctrl Pts',(-0.8564061976507,-0.9471386793648,-28.01455070646));
#21982=CARTESIAN_POINT('Ctrl Pts',(-1.270464502452,-0.128153038634,-28.07305070646));
#21983=CARTESIAN_POINT('Ctrl Pts',(-1.028306986882,0.7570257552148,-28.13155070646));
#21984=CARTESIAN_POINT('Ctrl Pts',(-0.2550119921671,1.251188290122,-28.19005070646));
#21985=CARTESIAN_POINT('Ctrl Pts',(0.6500008921559,1.099091485012,-28.24855070646));
#21986=CARTESIAN_POINT('Ctrl Pts',(1.219277621892,0.3792958445976,-28.30705070646));
#21987=CARTESIAN_POINT('Ctrl Pts',(1.158777391072,-0.5364123471407,-28.36555070646));
#21988=CARTESIAN_POINT('Ctrl Pts',(0.4997495938416,-1.175054711072,-28.42405070646));
#21989=CARTESIAN_POINT('Ctrl Pts',(-0.4174071783611,-1.206762071712,-28.48255070646));
#21990=CARTESIAN_POINT('Ctrl Pts',(-1.118965951462,-0.6151566299543,-28.54105070646));
#21991=CARTESIAN_POINT('Ctrl Pts',(-1.242561604939,0.2941860805683,-28.59955070646));
#21992=CARTESIAN_POINT('Ctrl Pts',(-0.7243492415226,1.051581514981,-28.65805070646));
#21993=CARTESIAN_POINT('Ctrl Pts',(0.1679846215786,1.265800345569,-28.71655070646));
#21994=CARTESIAN_POINT('Ctrl Pts',(0.9736143708746,0.8262775865961,-28.77505070646));
#21995=CARTESIAN_POINT('Ctrl Pts',(1.27612225025,-0.04027416205452,-28.83355070646));
#21996=CARTESIAN_POINT('Ctrl Pts',(1.038951010123,-0.603502507076,-28.87255070646));
#21997=CARTESIAN_POINT('Ctrl Pts',(0.8405914827566,-0.809484597174,-28.89205070646));
#21998=CARTESIAN_POINT('',(-1.10987074437248,-0.360618864706213,-26.9000774755696));
#21999=CARTESIAN_POINT('',(-1.10987074442631,-0.360618864754735,-27.0155475173803));
#22000=CARTESIAN_POINT('',(-1.109870874299,-0.360618907335,-26.90007747308));
#22001=CARTESIAN_POINT('Ctrl Pts',(-1.1090896887684,-0.360362786612198,
-27.0155263221856));
#22002=CARTESIAN_POINT('Ctrl Pts',(-1.1353675790678,-0.280038839228305,
-27.021289639903));
#22003=CARTESIAN_POINT('Ctrl Pts',(-1.15309370880972,-0.196900618773424,
-27.0270583193289));
#22004=CARTESIAN_POINT('Ctrl Pts',(-1.16987757186606,-0.0278535081970832,
-27.0386648185785));
#22005=CARTESIAN_POINT('Ctrl Pts',(-1.16850615302417,0.0569319254105346,
-27.0444246367462));
#22006=CARTESIAN_POINT('Ctrl Pts',(-1.13895411984996,0.29246549187405,-27.0606247655881));
#22007=CARTESIAN_POINT('Ctrl Pts',(-1.09008227583705,0.440659717710459,
-27.0710522198587));
#22008=CARTESIAN_POINT('Ctrl Pts',(-0.939712152246719,0.708957308483853,
-27.0920310449811));
#22009=CARTESIAN_POINT('Ctrl Pts',(-0.839559983040467,0.824971631429354,
-27.102302863744));
#22010=CARTESIAN_POINT('Ctrl Pts',(-0.597984012908985,1.01216444806353,
-27.1231468506276));
#22011=CARTESIAN_POINT('Ctrl Pts',(-0.460372021004354,1.08196013685235,
-27.1334627805692));
#22012=CARTESIAN_POINT('Ctrl Pts',(-0.167549532895036,1.16518146736364,
-27.1542375650593));
#22013=CARTESIAN_POINT('Ctrl Pts',(-0.0172110229777723,1.17670768237989,
-27.1643397811049));
#22014=CARTESIAN_POINT('Ctrl Pts',(0.285049692098096,1.14022956352786,-27.1850966850866));
#22015=CARTESIAN_POINT('Ctrl Pts',(0.43049544521667,1.09419678253459,-27.1953023673022));
#22016=CARTESIAN_POINT('Ctrl Pts',(0.716809839346208,0.938087220208753,
-27.2175666426251));
#22017=CARTESIAN_POINT('Ctrl Pts',(0.828634365706049,0.830823604335811,
-27.2279248529789));
#22018=CARTESIAN_POINT('Ctrl Pts',(1.00160136178627,0.614592612986834,-27.2467982047513));
#22019=CARTESIAN_POINT('Ctrl Pts',(1.07270922365843,0.481638865043252,-27.2568916601276));
#22020=CARTESIAN_POINT('Ctrl Pts',(1.16912240263033,0.168062342229928,-27.2792958601875));
#22021=CARTESIAN_POINT('Ctrl Pts',(1.17276985827545,0.0110285923520621,
-27.2897825979079));
#22022=CARTESIAN_POINT('Ctrl Pts',(1.14605683889197,-0.259178152412114,
-27.3082867322752));
#22023=CARTESIAN_POINT('Ctrl Pts',(1.1049312931433,-0.402369072521155,-27.3182677916966));
#22024=CARTESIAN_POINT('Ctrl Pts',(0.957339906864926,-0.69099968362001,
-27.3404107238413));
#22025=CARTESIAN_POINT('Ctrl Pts',(0.849977439951136,-0.808314046320928,
-27.3510273049907));
#22026=CARTESIAN_POINT('Ctrl Pts',(0.641616188680965,-0.984288752852637,
-27.3696126930084));
#22027=CARTESIAN_POINT('Ctrl Pts',(0.513628372088824,-1.05793609215418,
-27.3795125735442));
#22028=CARTESIAN_POINT('Ctrl Pts',(0.228920209503694,-1.15478736582146,
-27.400055060696));
#22029=CARTESIAN_POINT('Ctrl Pts',(0.0714241877483168,-1.17399633203817,
-27.4106622296586));
#22030=CARTESIAN_POINT('Ctrl Pts',(-0.203531273591206,-1.15448321757536,
-27.4294473277747));
#22031=CARTESIAN_POINT('Ctrl Pts',(-0.352078935195878,-1.12632096557171,
-27.4395560462991));
#22032=CARTESIAN_POINT('Ctrl Pts',(-0.64739480628011,-0.982811598955728,
-27.4619812077134));
#22033=CARTESIAN_POINT('Ctrl Pts',(-0.772891490596436,-0.886382061656004,
-27.472558053066));
#22034=CARTESIAN_POINT('Ctrl Pts',(-0.959484992736287,-0.675114426088524,
-27.4917705495728));
#22035=CARTESIAN_POINT('Ctrl Pts',(-1.04434540511724,-0.549317232093508,
-27.5019230808371));
#22036=CARTESIAN_POINT('Ctrl Pts',(-1.1515608225355,-0.240698826534252,
-27.5242292828711));
#22037=CARTESIAN_POINT('Ctrl Pts',(-1.172855145901,-0.0847008837209633,
-27.5347495650282));
#22038=CARTESIAN_POINT('Ctrl Pts',(-1.1553273946675,0.2249882773451,-27.555898376323));
#22039=CARTESIAN_POINT('Ctrl Pts',(-1.11708899258416,0.370182100385514,
-27.5659604824617));
#22040=CARTESIAN_POINT('Ctrl Pts',(-0.984380269778333,0.643433278699838,
-27.5866904752756));
#22041=CARTESIAN_POINT('Ctrl Pts',(-0.890301982635328,0.768087674628798,
-27.59712681397));
#22042=CARTESIAN_POINT('Ctrl Pts',(-0.66155868775765,0.973611514425885,
-27.6181021416964));
#22043=CARTESIAN_POINT('Ctrl Pts',(-0.529578637445949,1.0512078955982,-27.6283633413595));
#22044=CARTESIAN_POINT('Ctrl Pts',(-0.240409186122318,1.15078313340772,
-27.6492232952252));
#22045=CARTESIAN_POINT('Ctrl Pts',(-0.087461943617362,1.17256057451052,
-27.6595514605358));
#22046=CARTESIAN_POINT('Ctrl Pts',(0.215278414854982,1.15709812005245,-27.6802380394372));
#22047=CARTESIAN_POINT('Ctrl Pts',(0.361409610940379,1.12019171609551,-27.6903371103176));
#22048=CARTESIAN_POINT('Ctrl Pts',(0.637209668148432,0.98762997462939,-27.7112005351714));
#22049=CARTESIAN_POINT('Ctrl Pts',(0.76021498715122,0.897029079457893,-27.7214196096765));
#22050=CARTESIAN_POINT('Ctrl Pts',(0.980813909196912,0.657035707477414,
-27.7436737563467));
#22051=CARTESIAN_POINT('Ctrl Pts',(1.05211545721986,0.519720702111876,-27.7540179844193));
#22052=CARTESIAN_POINT('Ctrl Pts',(1.14631134349229,0.258739401713321,-27.7729300210825));
#22053=CARTESIAN_POINT('Ctrl Pts',(1.17073802586279,0.10974099037791,-27.783036857759));
#22054=CARTESIAN_POINT('Ctrl Pts',(1.1608022340359,-0.217860149407178,-27.8054191523545));
#22055=CARTESIAN_POINT('Ctrl Pts',(1.11384179304919,-0.367478577023206,
-27.8158902244773));
#22056=CARTESIAN_POINT('Ctrl Pts',(1.00106258513422,-0.615242280715572,
-27.8344423045362));
#22057=CARTESIAN_POINT('Ctrl Pts',(0.915771023800586,-0.737649456469355,
-27.8444366233426));
#22058=CARTESIAN_POINT('Ctrl Pts',(0.671599012721525,-0.974057539532169,
-27.8676508056259));
#22059=CARTESIAN_POINT('Ctrl Pts',(0.525608038221144,-1.04645149616782,
-27.8784973022941));
#22060=CARTESIAN_POINT('Ctrl Pts',(0.289520576217103,-1.13869075984127,
-27.8957700105567));
#22061=CARTESIAN_POINT('Ctrl Pts',(0.144847436238182,-1.1669872981076,-27.9056531858431));
#22062=CARTESIAN_POINT('Ctrl Pts',(-0.144847436238183,-1.1669872981076,
-27.9254418679969));
#22063=CARTESIAN_POINT('Ctrl Pts',(-0.289520576217105,-1.13869075984127,
-27.9353250432865));
#22064=CARTESIAN_POINT('Ctrl Pts',(-0.525608038221115,-1.04645149616783,
-27.9525977515491));
#22065=CARTESIAN_POINT('Ctrl Pts',(-0.671599012721508,-0.974057539532187,
-27.9634442482174));
#22066=CARTESIAN_POINT('Ctrl Pts',(-0.915771023800589,-0.737649456469351,
-27.9866584305007));
#22067=CARTESIAN_POINT('Ctrl Pts',(-1.00106258513423,-0.615242280715567,
-27.9966527493071));
#22068=CARTESIAN_POINT('Ctrl Pts',(-1.11384179304919,-0.367478577023195,
-28.0152048293662));
#22069=CARTESIAN_POINT('Ctrl Pts',(-1.1608022340359,-0.217860149407165,
-28.025675901489));
#22070=CARTESIAN_POINT('Ctrl Pts',(-1.17073802586279,0.109740990377929,
-28.0480581960845));
#22071=CARTESIAN_POINT('Ctrl Pts',(-1.14631134349228,0.258739401713341,
-28.0581650327611));
#22072=CARTESIAN_POINT('Ctrl Pts',(-1.05211545721985,0.519720702111896,
-28.0770770694243));
#22073=CARTESIAN_POINT('Ctrl Pts',(-0.980813909196899,0.657035707477435,
-28.0874212974969));
#22074=CARTESIAN_POINT('Ctrl Pts',(-0.760214987151199,0.897029079457912,
-28.1096754441671));
#22075=CARTESIAN_POINT('Ctrl Pts',(-0.637209668148406,0.987629974629407,
-28.1198945186723));
#22076=CARTESIAN_POINT('Ctrl Pts',(-0.361409610940352,1.12019171609552,
-28.140757943526));
#22077=CARTESIAN_POINT('Ctrl Pts',(-0.215278414854954,1.15709812005246,
-28.1508570144065));
#22078=CARTESIAN_POINT('Ctrl Pts',(0.0874619436173922,1.17256057451051,
-28.1715435933079));
#22079=CARTESIAN_POINT('Ctrl Pts',(0.240409186122349,1.15078313340772,-28.1818717586184));
#22080=CARTESIAN_POINT('Ctrl Pts',(0.529578637445975,1.05120789559819,-28.202731712484));
#22081=CARTESIAN_POINT('Ctrl Pts',(0.661558687757671,0.97361151442587,-28.212992912147));
#22082=CARTESIAN_POINT('Ctrl Pts',(0.890301982635341,0.768087674628783,
-28.2339682398733));
#22083=CARTESIAN_POINT('Ctrl Pts',(0.984380269778343,0.643433278699822,
-28.2444045785678));
#22084=CARTESIAN_POINT('Ctrl Pts',(1.11708899258417,0.370182100385499,-28.2651345713816));
#22085=CARTESIAN_POINT('Ctrl Pts',(1.1553273946675,0.224988277345085,-28.2751966775203));
#22086=CARTESIAN_POINT('Ctrl Pts',(1.17285514590099,-0.0847008837209673,
-28.2963454888151));
#22087=CARTESIAN_POINT('Ctrl Pts',(1.15156082253549,-0.240698826534245,
-28.3068657709722));
#22088=CARTESIAN_POINT('Ctrl Pts',(1.04434540511724,-0.549317232093477,
-28.3291719730061));
#22089=CARTESIAN_POINT('Ctrl Pts',(0.959484992736284,-0.675114426088482,
-28.3393245042704));
#22090=CARTESIAN_POINT('Ctrl Pts',(0.77289149059643,-0.886382061655964,
-28.3585370007771));
#22091=CARTESIAN_POINT('Ctrl Pts',(0.647394806280091,-0.982811598955699,
-28.3691138461296));
#22092=CARTESIAN_POINT('Ctrl Pts',(0.352078935195832,-1.12632096557171,
-28.3915390075439));
#22093=CARTESIAN_POINT('Ctrl Pts',(0.203531273591148,-1.15448321757536,
-28.4016477260684));
#22094=CARTESIAN_POINT('Ctrl Pts',(-0.0714241877483651,-1.17399633203817,
-28.4204328241847));
#22095=CARTESIAN_POINT('Ctrl Pts',(-0.228920209503715,-1.15478736582145,
-28.4310399931476));
#22096=CARTESIAN_POINT('Ctrl Pts',(-0.513628372088804,-1.05793609215417,
-28.4515824802994));
#22097=CARTESIAN_POINT('Ctrl Pts',(-0.641616188680927,-0.984288752852624,
-28.4614823608352));
#22098=CARTESIAN_POINT('Ctrl Pts',(-0.849977439951157,-0.808314046320862,
-28.4800677488528));
#22099=CARTESIAN_POINT('Ctrl Pts',(-0.957339906864942,-0.69099968361991,
-28.4906843300021));
#22100=CARTESIAN_POINT('Ctrl Pts',(-1.1049312931433,-0.402369072521084,
-28.5128272621466));
#22101=CARTESIAN_POINT('Ctrl Pts',(-1.14605683889198,-0.25917815241204,
-28.5228083215678));
#22102=CARTESIAN_POINT('Ctrl Pts',(-1.17276985827545,0.011028592352134,
-28.5413124559349));
#22103=CARTESIAN_POINT('Ctrl Pts',(-1.16912240263032,0.168062342229976,
-28.5517991936552));
#22104=CARTESIAN_POINT('Ctrl Pts',(-1.07270922365842,0.481638865043274,
-28.5742033937153));
#22105=CARTESIAN_POINT('Ctrl Pts',(-1.00160136178626,0.614592612986856,
-28.5842968490919));
#22106=CARTESIAN_POINT('Ctrl Pts',(-0.828634365706032,0.830823604335828,
-28.6031702008645));
#22107=CARTESIAN_POINT('Ctrl Pts',(-0.716809839346184,0.938087220208773,
-28.6135284112185));
#22108=CARTESIAN_POINT('Ctrl Pts',(-0.430495445216628,1.0941967825346,-28.6357926865415));
#22109=CARTESIAN_POINT('Ctrl Pts',(-0.285049692098049,1.14022956352787,
-28.645998368757));
#22110=CARTESIAN_POINT('Ctrl Pts',(0.0172110229778327,1.17670768237989,
-28.6667552727386));
#22111=CARTESIAN_POINT('Ctrl Pts',(0.167549532895092,1.16518146736363,-28.6768574887841));
#22112=CARTESIAN_POINT('Ctrl Pts',(0.460372021004397,1.08196013685233,-28.6976322732742));
#22113=CARTESIAN_POINT('Ctrl Pts',(0.597984012909024,1.01216444806351,-28.7079482032158));
#22114=CARTESIAN_POINT('Ctrl Pts',(0.839559983040498,0.824971631429321,
-28.7287921900993));
#22115=CARTESIAN_POINT('Ctrl Pts',(0.939712152246743,0.708957308483815,
-28.7390640088623));
#22116=CARTESIAN_POINT('Ctrl Pts',(1.09008227583707,0.440659717710412,-28.7600428339848));
#22117=CARTESIAN_POINT('Ctrl Pts',(1.13895411984998,0.292465491873993,-28.7704702882555));
#22118=CARTESIAN_POINT('Ctrl Pts',(1.16850615302413,0.0569319254108322,
-28.7866704170975));
#22119=CARTESIAN_POINT('Ctrl Pts',(1.16987757186605,-0.0278535081964251,
-28.7924302352651));
#22120=CARTESIAN_POINT('Ctrl Pts',(1.15309371461848,-0.1969005602683,-28.8040367304978));
#22121=CARTESIAN_POINT('Ctrl Pts',(1.13536760373153,-0.280038723551826,
-28.809805405914));
#22122=CARTESIAN_POINT('Ctrl Pts',(1.10908974361186,-0.360362618971496,
-28.8155687196295));
#22123=CARTESIAN_POINT('Ctrl Pts',(-1.10908974361187,-0.360362618971445,
-26.9000562803705));
#22124=CARTESIAN_POINT('Ctrl Pts',(-1.13536760373151,-0.280038723551868,
-26.905819594086));
#22125=CARTESIAN_POINT('Ctrl Pts',(-1.15309371461845,-0.196900560268445,
-26.9115882695022));
#22126=CARTESIAN_POINT('Ctrl Pts',(-1.16987757186605,-0.0278535081965757,
-26.9231947647349));
#22127=CARTESIAN_POINT('Ctrl Pts',(-1.16850615302414,0.0569319254107759,
-26.9289545829025));
#22128=CARTESIAN_POINT('Ctrl Pts',(-1.13895411984997,0.292465491874028,
-26.9451547117445));
#22129=CARTESIAN_POINT('Ctrl Pts',(-1.09008227583706,0.440659717710443,
-26.9555821660152));
#22130=CARTESIAN_POINT('Ctrl Pts',(-0.939712152246728,0.708957308483841,
-26.9765609911377));
#22131=CARTESIAN_POINT('Ctrl Pts',(-0.839559983040477,0.824971631429344,
-26.9868328099007));
#22132=CARTESIAN_POINT('Ctrl Pts',(-0.597984012908997,1.01216444806352,
-27.0076767967842));
#22133=CARTESIAN_POINT('Ctrl Pts',(-0.460372021004369,1.08196013685234,
-27.0179927267258));
#22134=CARTESIAN_POINT('Ctrl Pts',(-0.167549532895057,1.16518146736364,
-27.0387675112159));
#22135=CARTESIAN_POINT('Ctrl Pts',(-0.0172110229777962,1.17670768237989,
-27.0488697272614));
#22136=CARTESIAN_POINT('Ctrl Pts',(0.285049692098077,1.14022956352786,-27.069626631243));
#22137=CARTESIAN_POINT('Ctrl Pts',(0.430495445216654,1.09419678253459,-27.0798323134585));
#22138=CARTESIAN_POINT('Ctrl Pts',(0.716809839346204,0.938087220208758,
-27.1020965887815));
#22139=CARTESIAN_POINT('Ctrl Pts',(0.828634365706049,0.830823604335812,
-27.1124547991355));
#22140=CARTESIAN_POINT('Ctrl Pts',(1.00160136178628,0.614592612986832,-27.1313281509081));
#22141=CARTESIAN_POINT('Ctrl Pts',(1.07270922365843,0.481638865043245,-27.1414216062847));
#22142=CARTESIAN_POINT('Ctrl Pts',(1.16912240263033,0.168062342229917,-27.1638258063448));
#22143=CARTESIAN_POINT('Ctrl Pts',(1.17276985827545,0.0110285923520512,
-27.1743125440651));
#22144=CARTESIAN_POINT('Ctrl Pts',(1.14605683889197,-0.25917815241212,-27.1928166784322));
#22145=CARTESIAN_POINT('Ctrl Pts',(1.1049312931433,-0.402369072521154,-27.2027977378534));
#22146=CARTESIAN_POINT('Ctrl Pts',(0.957339906864935,-0.690999683619994,
-27.2249406699979));
#22147=CARTESIAN_POINT('Ctrl Pts',(0.849977439951153,-0.80831404632091,
-27.2355572511472));
#22148=CARTESIAN_POINT('Ctrl Pts',(0.64161618868098,-0.984288752852628,
-27.2541426391648));
#22149=CARTESIAN_POINT('Ctrl Pts',(0.513628372088837,-1.05793609215418,
-27.2640425197005));
#22150=CARTESIAN_POINT('Ctrl Pts',(0.228920209503699,-1.15478736582146,
-27.2845850068524));
#22151=CARTESIAN_POINT('Ctrl Pts',(0.0714241877483137,-1.17399633203818,
-27.2951921758153));
#22152=CARTESIAN_POINT('Ctrl Pts',(-0.203531273591216,-1.15448321757536,
-27.3139772739317));
#22153=CARTESIAN_POINT('Ctrl Pts',(-0.352078935195889,-1.12632096557171,
-27.3240859924561));
#22154=CARTESIAN_POINT('Ctrl Pts',(-0.647394806280115,-0.982811598955724,
-27.3465111538704));
#22155=CARTESIAN_POINT('Ctrl Pts',(-0.772891490596438,-0.886382061656001,
-27.3570879992229));
#22156=CARTESIAN_POINT('Ctrl Pts',(-0.959484992736288,-0.675114426088524,
-27.3763004957296));
#22157=CARTESIAN_POINT('Ctrl Pts',(-1.04434540511724,-0.549317232093508,
-27.3864530269939));
#22158=CARTESIAN_POINT('Ctrl Pts',(-1.1515608225355,-0.240698826534257,
-27.4087592290278));
#22159=CARTESIAN_POINT('Ctrl Pts',(-1.172855145901,-0.084700883720971,-27.4192795111849));
#22160=CARTESIAN_POINT('Ctrl Pts',(-1.1553273946675,0.224988277345099,-27.4404283224797));
#22161=CARTESIAN_POINT('Ctrl Pts',(-1.11708899258416,0.370182100385512,
-27.4504904286184));
#22162=CARTESIAN_POINT('Ctrl Pts',(-0.984380269778341,0.643433278699826,
-27.4712204214322));
#22163=CARTESIAN_POINT('Ctrl Pts',(-0.890301982635338,0.768087674628786,
-27.4816567601267));
#22164=CARTESIAN_POINT('Ctrl Pts',(-0.661558687757666,0.973611514425873,
-27.502632087853));
#22165=CARTESIAN_POINT('Ctrl Pts',(-0.52957863744597,1.05120789559819,-27.512893287516));
#22166=CARTESIAN_POINT('Ctrl Pts',(-0.240409186122344,1.15078313340772,
-27.5337532413816));
#22167=CARTESIAN_POINT('Ctrl Pts',(-0.0874619436173883,1.17256057451051,
-27.5440814066922));
#22168=CARTESIAN_POINT('Ctrl Pts',(0.215278414854953,1.15709812005246,-27.5647679855935));
#22169=CARTESIAN_POINT('Ctrl Pts',(0.361409610940351,1.12019171609552,-27.574867056474));
#22170=CARTESIAN_POINT('Ctrl Pts',(0.637209668148408,0.987629974629406,
-27.5957304813277));
#22171=CARTESIAN_POINT('Ctrl Pts',(0.7602149871512,0.897029079457911,-27.6059495558329));
#22172=CARTESIAN_POINT('Ctrl Pts',(0.980813909196898,0.657035707477434,
-27.6282037025032));
#22173=CARTESIAN_POINT('Ctrl Pts',(1.05211545721985,0.519720702111898,-27.6385479305757));
#22174=CARTESIAN_POINT('Ctrl Pts',(1.14631134349228,0.258739401713341,-27.6574599672389));
#22175=CARTESIAN_POINT('Ctrl Pts',(1.17073802586279,0.109740990377928,-27.6675668039155));
#22176=CARTESIAN_POINT('Ctrl Pts',(1.1608022340359,-0.217860149407165,-27.689949098511));
#22177=CARTESIAN_POINT('Ctrl Pts',(1.11384179304919,-0.367478577023196,
-27.7004201706339));
#22178=CARTESIAN_POINT('Ctrl Pts',(1.00106258513423,-0.615242280715565,
-27.7189722506929));
#22179=CARTESIAN_POINT('Ctrl Pts',(0.91577102380059,-0.73764945646935,-27.7289665694993));
#22180=CARTESIAN_POINT('Ctrl Pts',(0.671599012721526,-0.974057539532169,
-27.7521807517826));
#22181=CARTESIAN_POINT('Ctrl Pts',(0.525608038221143,-1.04645149616782,
-27.7630272484509));
#22182=CARTESIAN_POINT('Ctrl Pts',(0.289520576217104,-1.13869075984127,
-27.7802999567135));
#22183=CARTESIAN_POINT('Ctrl Pts',(0.144847436238183,-1.1669872981076,-27.7901831320031));
#22184=CARTESIAN_POINT('Ctrl Pts',(-0.144847436238183,-1.1669872981076,
-27.8099718141569));
#22185=CARTESIAN_POINT('Ctrl Pts',(-0.289520576217104,-1.13869075984127,
-27.8198549894433));
#22186=CARTESIAN_POINT('Ctrl Pts',(-0.525608038221108,-1.04645149616784,
-27.8371276977059));
#22187=CARTESIAN_POINT('Ctrl Pts',(-0.671599012721502,-0.974057539532192,
-27.8479741943741));
#22188=CARTESIAN_POINT('Ctrl Pts',(-0.915771023800586,-0.737649456469355,
-27.8711883766574));
#22189=CARTESIAN_POINT('Ctrl Pts',(-1.00106258513422,-0.615242280715573,
-27.8811826954638));
#22190=CARTESIAN_POINT('Ctrl Pts',(-1.11384179304919,-0.367478577023206,
-27.8997347755227));
#22191=CARTESIAN_POINT('Ctrl Pts',(-1.1608022340359,-0.21786014940718,-27.9102058476455));
#22192=CARTESIAN_POINT('Ctrl Pts',(-1.17073802586279,0.10974099037791,-27.932588142241));
#22193=CARTESIAN_POINT('Ctrl Pts',(-1.14631134349229,0.25873940171332,-27.9426949789175));
#22194=CARTESIAN_POINT('Ctrl Pts',(-1.05211545721986,0.519720702111875,
-27.9616070155807));
#22195=CARTESIAN_POINT('Ctrl Pts',(-0.980813909196912,0.657035707477414,
-27.9719512436533));
#22196=CARTESIAN_POINT('Ctrl Pts',(-0.76021498715122,0.897029079457893,
-27.9942053903235));
#22197=CARTESIAN_POINT('Ctrl Pts',(-0.637209668148432,0.98762997462939,
-28.0044244648287));
#22198=CARTESIAN_POINT('Ctrl Pts',(-0.361409610940396,1.1201917160955,-28.0252878896824));
#22199=CARTESIAN_POINT('Ctrl Pts',(-0.215278414855001,1.15709812005245,
-28.0353869605628));
#22200=CARTESIAN_POINT('Ctrl Pts',(0.0874619436173592,1.17256057451052,
-28.0560735394642));
#22201=CARTESIAN_POINT('Ctrl Pts',(0.240409186122314,1.15078313340772,-28.0664017047748));
#22202=CARTESIAN_POINT('Ctrl Pts',(0.529578637445944,1.0512078955982,-28.0872616586405));
#22203=CARTESIAN_POINT('Ctrl Pts',(0.661558687757645,0.973611514425888,
-28.0975228583036));
#22204=CARTESIAN_POINT('Ctrl Pts',(0.890301982635324,0.768087674628803,
-28.11849818603));
#22205=CARTESIAN_POINT('Ctrl Pts',(0.984380269778329,0.643433278699844,
-28.1289345247244));
#22206=CARTESIAN_POINT('Ctrl Pts',(1.11708899258416,0.370182100385531,-28.1496645175383));
#22207=CARTESIAN_POINT('Ctrl Pts',(1.1553273946675,0.224988277345117,-28.159726623677));
#22208=CARTESIAN_POINT('Ctrl Pts',(1.172855145901,-0.0847008837209511,-28.1808754349718));
#22209=CARTESIAN_POINT('Ctrl Pts',(1.1515608225355,-0.240698826534231,-28.1913957171289));
#22210=CARTESIAN_POINT('Ctrl Pts',(1.04434540511724,-0.549317232093467,
-28.2137019191629));
#22211=CARTESIAN_POINT('Ctrl Pts',(0.959484992736289,-0.675114426088475,
-28.2238544504272));
#22212=CARTESIAN_POINT('Ctrl Pts',(0.772891490596436,-0.886382061655959,
-28.243066946934));
#22213=CARTESIAN_POINT('Ctrl Pts',(0.647394806280094,-0.982811598955698,
-28.2536437922866));
#22214=CARTESIAN_POINT('Ctrl Pts',(0.352078935195833,-1.12632096557171,
-28.2760689537009));
#22215=CARTESIAN_POINT('Ctrl Pts',(0.203531273591151,-1.15448321757536,
-28.2861776722252));
#22216=CARTESIAN_POINT('Ctrl Pts',(-0.0714241877483557,-1.17399633203817,
-28.3049627703414));
#22217=CARTESIAN_POINT('Ctrl Pts',(-0.228920209503697,-1.15478736582145,
-28.315569939304));
#22218=CARTESIAN_POINT('Ctrl Pts',(-0.513628372088781,-1.05793609215418,
-28.3361124264558));
#22219=CARTESIAN_POINT('Ctrl Pts',(-0.641616188680906,-0.984288752852638,
-28.3460123069916));
#22220=CARTESIAN_POINT('Ctrl Pts',(-0.849977439951128,-0.80831404632089,
-28.3645976950093));
#22221=CARTESIAN_POINT('Ctrl Pts',(-0.957339906864927,-0.690999683619937,
-28.3752142761587));
#22222=CARTESIAN_POINT('Ctrl Pts',(-1.1049312931433,-0.402369072521088,
-28.3973572083034));
#22223=CARTESIAN_POINT('Ctrl Pts',(-1.14605683889198,-0.259178152412038,
-28.4073382677248));
#22224=CARTESIAN_POINT('Ctrl Pts',(-1.17276985827545,0.0110285923521394,
-28.425842402092));
#22225=CARTESIAN_POINT('Ctrl Pts',(-1.16912240263032,0.168062342229981,
-28.4363291398125));
#22226=CARTESIAN_POINT('Ctrl Pts',(-1.07270922365842,0.481638865043275,
-28.4587333398723));
#22227=CARTESIAN_POINT('Ctrl Pts',(-1.00160136178626,0.614592612986852,
-28.4688267952487));
#22228=CARTESIAN_POINT('Ctrl Pts',(-0.828634365706037,0.830823604335824,
-28.4877001470211));
#22229=CARTESIAN_POINT('Ctrl Pts',(-0.716809839346193,0.938087220208765,
-28.4980583573749));
#22230=CARTESIAN_POINT('Ctrl Pts',(-0.430495445216648,1.0941967825346,-28.5203226326978));
#22231=CARTESIAN_POINT('Ctrl Pts',(-0.285049692098074,1.14022956352786,
-28.5305283149134));
#22232=CARTESIAN_POINT('Ctrl Pts',(0.0172110229777963,1.17670768237989,
-28.5512852188951));
#22233=CARTESIAN_POINT('Ctrl Pts',(0.16754953289506,1.16518146736364,-28.5613874349407));
#22234=CARTESIAN_POINT('Ctrl Pts',(0.460372021004377,1.08196013685234,-28.5821622194308));
#22235=CARTESIAN_POINT('Ctrl Pts',(0.597984012909007,1.01216444806352,-28.5924781493724));
#22236=CARTESIAN_POINT('Ctrl Pts',(0.839559983040483,0.824971631429336,
-28.6133221362559));
#22237=CARTESIAN_POINT('Ctrl Pts',(0.939712152246731,0.708957308483833,
-28.6235939550189));
#22238=CARTESIAN_POINT('Ctrl Pts',(1.09008227583706,0.440659717710434,-28.6445727801413));
#22239=CARTESIAN_POINT('Ctrl Pts',(1.13895411984997,0.292465491874021,-28.6550002344119));
#22240=CARTESIAN_POINT('Ctrl Pts',(1.16850615302418,0.0569319254104148,
-28.6712003632538));
#22241=CARTESIAN_POINT('Ctrl Pts',(1.16987757186606,-0.0278535081972872,
-28.6769601814215));
#22242=CARTESIAN_POINT('Ctrl Pts',(1.15309370880968,-0.19690061877361,-28.6885666806711));
#22243=CARTESIAN_POINT('Ctrl Pts',(1.13536757906777,-0.28003883922839,-28.694335360097));
#22244=CARTESIAN_POINT('Ctrl Pts',(1.1090896887684,-0.360362786612186,-28.7000986778144));
#22245=CARTESIAN_POINT('Ctrl Pts',(0.2042496867001,1.148974072566,-25.02357429354));
#22246=CARTESIAN_POINT('Ctrl Pts',(0.485799150132,1.098923865977,-25.04307429354));
#22247=CARTESIAN_POINT('Ctrl Pts',(1.008732028848,0.7826683203553,-25.08207429354));
#22248=CARTESIAN_POINT('Ctrl Pts',(1.273344351706,-0.09619644100725,-25.14057429354));
#22249=CARTESIAN_POINT('Ctrl Pts',(0.8799211891228,-0.9253151078751,-25.19907429354));
#22250=CARTESIAN_POINT('Ctrl Pts',(0.03209325983472,-1.276509118266,-25.25757429354));
#22251=CARTESIAN_POINT('Ctrl Pts',(-0.8323352153661,-0.9683609251365,-25.31607429354));
#22252=CARTESIAN_POINT('Ctrl Pts',(-1.266842465797,-0.1600395162514,-25.37457429354));
#22253=CARTESIAN_POINT('Ctrl Pts',(-1.047006449646,0.7309452405402,-25.43307429354));
#22254=CARTESIAN_POINT('Ctrl Pts',(-0.2863739154552,1.244384671677,-25.49157429354));
#22255=CARTESIAN_POINT('Ctrl Pts',(0.6221753352776,1.115078965991,-25.55007429354));
#22256=CARTESIAN_POINT('Ctrl Pts',(1.209360820682,0.4098166204233,-25.60857429354));
#22257=CARTESIAN_POINT('Ctrl Pts',(1.171891533923,-0.5071227513611,-25.66707429354));
#22258=CARTESIAN_POINT('Ctrl Pts',(0.5291209893422,-1.162124878025,-25.72557429354));
#22259=CARTESIAN_POINT('Ctrl Pts',(-0.3869492533009,-1.216870382867,-25.78407429354));
#22260=CARTESIAN_POINT('Ctrl Pts',(-1.103153839379,-0.6430823119665,-25.84257429354));
#22261=CARTESIAN_POINT('Ctrl Pts',(-1.249561315594,0.262868354685,-25.90107429354));
#22262=CARTESIAN_POINT('Ctrl Pts',(-0.7505498113574,1.033043190765,-25.95957429354));
#22263=CARTESIAN_POINT('Ctrl Pts',(0.1361330203811,1.269634220587,-26.01807429354));
#22264=CARTESIAN_POINT('Ctrl Pts',(0.9525009070881,0.850438284238,-26.07657429354));
#22265=CARTESIAN_POINT('Ctrl Pts',(1.276886402343,-0.00802301942994,-26.13507429354));
#22266=CARTESIAN_POINT('Ctrl Pts',(0.9417390602074,-0.8623403017182,-26.19357429354));
#22267=CARTESIAN_POINT('Ctrl Pts',(0.1201679976972,-1.271244628134,-26.25207429354));
#22268=CARTESIAN_POINT('Ctrl Pts',(-0.7634718132617,-1.023530188774,-26.31057429354));
#22269=CARTESIAN_POINT('Ctrl Pts',(-1.252765868871,-0.2471455563325,-26.36907429354));
#22270=CARTESIAN_POINT('Ctrl Pts',(-1.094985744155,0.6568937894785,-26.42757429354));
#22271=CARTESIAN_POINT('Ctrl Pts',(-0.3716274479098,1.221636807823,-26.48607429354));
#22272=CARTESIAN_POINT('Ctrl Pts',(0.5436824759227,1.155383851922,-26.54457429354));
#22273=CARTESIAN_POINT('Ctrl Pts',(1.178171694542,0.49235784776,-26.60307429354));
#22274=CARTESIAN_POINT('Ctrl Pts',(1.204114952343,-0.4249855149138,-26.66157429354));
#22275=CARTESIAN_POINT('Ctrl Pts',(0.6081163618214,-1.122792874227,-26.72007429354));
#22276=CARTESIAN_POINT('Ctrl Pts',(-0.3019967923042,-1.240748778247,-26.77857429354));
#22277=CARTESIAN_POINT('Ctrl Pts',(-1.056077145856,-0.7175033572827,-26.83707429354));
#22278=CARTESIAN_POINT('Ctrl Pts',(-1.195258896894,-0.1224362972325,-26.87607429354));
#22279=CARTESIAN_POINT('Ctrl Pts',(-1.155855903054,0.1607995190315,-26.89557429354));
#22280=CARTESIAN_POINT('Ctrl Pts',(0.2042496867001,1.148974072566,-25.08906643118));
#22281=CARTESIAN_POINT('Ctrl Pts',(0.485799150132,1.098923865977,-25.10856643118));
#22282=CARTESIAN_POINT('Ctrl Pts',(1.008732028848,0.7826683203553,-25.14756643118));
#22283=CARTESIAN_POINT('Ctrl Pts',(1.273344351706,-0.09619644100725,-25.20606643118));
#22284=CARTESIAN_POINT('Ctrl Pts',(0.8799211891228,-0.9253151078751,-25.26456643118));
#22285=CARTESIAN_POINT('Ctrl Pts',(0.03209325983472,-1.276509118266,-25.32306643118));
#22286=CARTESIAN_POINT('Ctrl Pts',(-0.8323352153661,-0.9683609251365,-25.38156643118));
#22287=CARTESIAN_POINT('Ctrl Pts',(-1.266842465797,-0.1600395162514,-25.44006643118));
#22288=CARTESIAN_POINT('Ctrl Pts',(-1.047006449646,0.7309452405402,-25.49856643118));
#22289=CARTESIAN_POINT('Ctrl Pts',(-0.2863739154552,1.244384671677,-25.55706643118));
#22290=CARTESIAN_POINT('Ctrl Pts',(0.6221753352776,1.115078965991,-25.61556643118));
#22291=CARTESIAN_POINT('Ctrl Pts',(1.209360820682,0.4098166204233,-25.67406643118));
#22292=CARTESIAN_POINT('Ctrl Pts',(1.171891533923,-0.5071227513611,-25.73256643118));
#22293=CARTESIAN_POINT('Ctrl Pts',(0.5291209893422,-1.162124878025,-25.79106643118));
#22294=CARTESIAN_POINT('Ctrl Pts',(-0.3869492533009,-1.216870382867,-25.84956643118));
#22295=CARTESIAN_POINT('Ctrl Pts',(-1.103153839379,-0.6430823119665,-25.90806643118));
#22296=CARTESIAN_POINT('Ctrl Pts',(-1.249561315594,0.262868354685,-25.96656643118));
#22297=CARTESIAN_POINT('Ctrl Pts',(-0.7505498113574,1.033043190765,-26.02506643118));
#22298=CARTESIAN_POINT('Ctrl Pts',(0.1361330203811,1.269634220587,-26.08356643118));
#22299=CARTESIAN_POINT('Ctrl Pts',(0.9525009070881,0.850438284238,-26.14206643118));
#22300=CARTESIAN_POINT('Ctrl Pts',(1.276886402343,-0.00802301942994,-26.20056643118));
#22301=CARTESIAN_POINT('Ctrl Pts',(0.9417390602074,-0.8623403017182,-26.25906643118));
#22302=CARTESIAN_POINT('Ctrl Pts',(0.1201679976972,-1.271244628134,-26.31756643118));
#22303=CARTESIAN_POINT('Ctrl Pts',(-0.7634718132617,-1.023530188774,-26.37606643118));
#22304=CARTESIAN_POINT('Ctrl Pts',(-1.252765868871,-0.2471455563325,-26.43456643118));
#22305=CARTESIAN_POINT('Ctrl Pts',(-1.094985744155,0.6568937894785,-26.49306643118));
#22306=CARTESIAN_POINT('Ctrl Pts',(-0.3716274479098,1.221636807823,-26.55156643118));
#22307=CARTESIAN_POINT('Ctrl Pts',(0.5436824759227,1.155383851922,-26.61006643118));
#22308=CARTESIAN_POINT('Ctrl Pts',(1.178171694542,0.49235784776,-26.66856643118));
#22309=CARTESIAN_POINT('Ctrl Pts',(1.204114952343,-0.4249855149138,-26.72706643118));
#22310=CARTESIAN_POINT('Ctrl Pts',(0.6081163618214,-1.122792874227,-26.78556643118));
#22311=CARTESIAN_POINT('Ctrl Pts',(-0.3019967923042,-1.240748778247,-26.84406643118));
#22312=CARTESIAN_POINT('Ctrl Pts',(-1.056077145856,-0.7175033572827,-26.90256643118));
#22313=CARTESIAN_POINT('Ctrl Pts',(-1.195258896894,-0.1224362972325,-26.94156643118));
#22314=CARTESIAN_POINT('Ctrl Pts',(-1.155855903054,0.1607995190315,-26.96106643118));
#22315=CARTESIAN_POINT('Ctrl Pts',(0.2042496867001,1.148974072566,-25.15455856882));
#22316=CARTESIAN_POINT('Ctrl Pts',(0.485799150132,1.098923865977,-25.17405856882));
#22317=CARTESIAN_POINT('Ctrl Pts',(1.008732028848,0.7826683203553,-25.21305856882));
#22318=CARTESIAN_POINT('Ctrl Pts',(1.273344351706,-0.09619644100725,-25.27155856882));
#22319=CARTESIAN_POINT('Ctrl Pts',(0.8799211891228,-0.9253151078751,-25.33005856882));
#22320=CARTESIAN_POINT('Ctrl Pts',(0.03209325983473,-1.276509118266,-25.38855856882));
#22321=CARTESIAN_POINT('Ctrl Pts',(-0.8323352153661,-0.9683609251365,-25.44705856882));
#22322=CARTESIAN_POINT('Ctrl Pts',(-1.266842465797,-0.1600395162514,-25.50555856882));
#22323=CARTESIAN_POINT('Ctrl Pts',(-1.047006449646,0.7309452405402,-25.56405856882));
#22324=CARTESIAN_POINT('Ctrl Pts',(-0.2863739154552,1.244384671677,-25.62255856882));
#22325=CARTESIAN_POINT('Ctrl Pts',(0.6221753352776,1.115078965991,-25.68105856882));
#22326=CARTESIAN_POINT('Ctrl Pts',(1.209360820682,0.4098166204233,-25.73955856882));
#22327=CARTESIAN_POINT('Ctrl Pts',(1.171891533923,-0.5071227513611,-25.79805856882));
#22328=CARTESIAN_POINT('Ctrl Pts',(0.5291209893422,-1.162124878025,-25.85655856882));
#22329=CARTESIAN_POINT('Ctrl Pts',(-0.3869492533009,-1.216870382867,-25.91505856882));
#22330=CARTESIAN_POINT('Ctrl Pts',(-1.103153839379,-0.6430823119665,-25.97355856882));
#22331=CARTESIAN_POINT('Ctrl Pts',(-1.249561315594,0.262868354685,-26.03205856882));
#22332=CARTESIAN_POINT('Ctrl Pts',(-0.7505498113574,1.033043190765,-26.09055856882));
#22333=CARTESIAN_POINT('Ctrl Pts',(0.1361330203811,1.269634220587,-26.14905856882));
#22334=CARTESIAN_POINT('Ctrl Pts',(0.9525009070881,0.850438284238,-26.20755856882));
#22335=CARTESIAN_POINT('Ctrl Pts',(1.276886402343,-0.008023019429937,-26.26605856882));
#22336=CARTESIAN_POINT('Ctrl Pts',(0.9417390602074,-0.8623403017182,-26.32455856882));
#22337=CARTESIAN_POINT('Ctrl Pts',(0.1201679976972,-1.271244628134,-26.38305856882));
#22338=CARTESIAN_POINT('Ctrl Pts',(-0.7634718132616,-1.023530188774,-26.44155856882));
#22339=CARTESIAN_POINT('Ctrl Pts',(-1.252765868871,-0.2471455563325,-26.50005856882));
#22340=CARTESIAN_POINT('Ctrl Pts',(-1.094985744155,0.6568937894785,-26.55855856882));
#22341=CARTESIAN_POINT('Ctrl Pts',(-0.3716274479098,1.221636807823,-26.61705856882));
#22342=CARTESIAN_POINT('Ctrl Pts',(0.5436824759227,1.155383851922,-26.67555856882));
#22343=CARTESIAN_POINT('Ctrl Pts',(1.178171694542,0.49235784776,-26.73405856882));
#22344=CARTESIAN_POINT('Ctrl Pts',(1.204114952343,-0.4249855149138,-26.79255856882));
#22345=CARTESIAN_POINT('Ctrl Pts',(0.6081163618214,-1.122792874227,-26.85105856882));
#22346=CARTESIAN_POINT('Ctrl Pts',(-0.3019967923042,-1.240748778247,-26.90955856882));
#22347=CARTESIAN_POINT('Ctrl Pts',(-1.056077145856,-0.7175033572827,-26.96805856882));
#22348=CARTESIAN_POINT('Ctrl Pts',(-1.195258896894,-0.1224362972325,-27.00705856882));
#22349=CARTESIAN_POINT('Ctrl Pts',(-1.155855903054,0.1607995190315,-27.02655856882));
#22350=CARTESIAN_POINT('Ctrl Pts',(0.2042496867001,1.148974072566,-25.22005070646));
#22351=CARTESIAN_POINT('Ctrl Pts',(0.485799150132,1.098923865977,-25.23955070646));
#22352=CARTESIAN_POINT('Ctrl Pts',(1.008732028848,0.7826683203553,-25.27855070646));
#22353=CARTESIAN_POINT('Ctrl Pts',(1.273344351706,-0.09619644100725,-25.33705070646));
#22354=CARTESIAN_POINT('Ctrl Pts',(0.8799211891228,-0.9253151078751,-25.39555070646));
#22355=CARTESIAN_POINT('Ctrl Pts',(0.03209325983472,-1.276509118266,-25.45405070646));
#22356=CARTESIAN_POINT('Ctrl Pts',(-0.8323352153661,-0.9683609251365,-25.51255070646));
#22357=CARTESIAN_POINT('Ctrl Pts',(-1.266842465797,-0.1600395162514,-25.57105070646));
#22358=CARTESIAN_POINT('Ctrl Pts',(-1.047006449646,0.7309452405402,-25.62955070646));
#22359=CARTESIAN_POINT('Ctrl Pts',(-0.2863739154552,1.244384671677,-25.68805070646));
#22360=CARTESIAN_POINT('Ctrl Pts',(0.6221753352776,1.115078965991,-25.74655070646));
#22361=CARTESIAN_POINT('Ctrl Pts',(1.209360820682,0.4098166204233,-25.80505070646));
#22362=CARTESIAN_POINT('Ctrl Pts',(1.171891533923,-0.5071227513611,-25.86355070646));
#22363=CARTESIAN_POINT('Ctrl Pts',(0.5291209893422,-1.162124878025,-25.92205070646));
#22364=CARTESIAN_POINT('Ctrl Pts',(-0.3869492533009,-1.216870382867,-25.98055070646));
#22365=CARTESIAN_POINT('Ctrl Pts',(-1.103153839379,-0.6430823119665,-26.03905070646));
#22366=CARTESIAN_POINT('Ctrl Pts',(-1.249561315594,0.262868354685,-26.09755070646));
#22367=CARTESIAN_POINT('Ctrl Pts',(-0.7505498113574,1.033043190765,-26.15605070646));
#22368=CARTESIAN_POINT('Ctrl Pts',(0.1361330203811,1.269634220587,-26.21455070646));
#22369=CARTESIAN_POINT('Ctrl Pts',(0.9525009070881,0.850438284238,-26.27305070646));
#22370=CARTESIAN_POINT('Ctrl Pts',(1.276886402343,-0.008023019429937,-26.33155070646));
#22371=CARTESIAN_POINT('Ctrl Pts',(0.9417390602074,-0.8623403017182,-26.39005070646));
#22372=CARTESIAN_POINT('Ctrl Pts',(0.1201679976972,-1.271244628134,-26.44855070646));
#22373=CARTESIAN_POINT('Ctrl Pts',(-0.7634718132616,-1.023530188774,-26.50705070646));
#22374=CARTESIAN_POINT('Ctrl Pts',(-1.252765868871,-0.2471455563325,-26.56555070646));
#22375=CARTESIAN_POINT('Ctrl Pts',(-1.094985744155,0.6568937894785,-26.62405070646));
#22376=CARTESIAN_POINT('Ctrl Pts',(-0.3716274479098,1.221636807823,-26.68255070646));
#22377=CARTESIAN_POINT('Ctrl Pts',(0.5436824759227,1.155383851922,-26.74105070646));
#22378=CARTESIAN_POINT('Ctrl Pts',(1.178171694542,0.49235784776,-26.79955070646));
#22379=CARTESIAN_POINT('Ctrl Pts',(1.204114952343,-0.4249855149138,-26.85805070646));
#22380=CARTESIAN_POINT('Ctrl Pts',(0.6081163618214,-1.122792874227,-26.91655070646));
#22381=CARTESIAN_POINT('Ctrl Pts',(-0.3019967923042,-1.240748778247,-26.97505070646));
#22382=CARTESIAN_POINT('Ctrl Pts',(-1.056077145856,-0.7175033572827,-27.03355070646));
#22383=CARTESIAN_POINT('Ctrl Pts',(-1.195258896894,-0.1224362972325,-27.07255070646));
#22384=CARTESIAN_POINT('Ctrl Pts',(-1.155855903054,0.1607995190315,-27.09205070646));
#22385=CARTESIAN_POINT('',(0.685937843384214,0.944112445532598,-25.1000774755696));
#22386=CARTESIAN_POINT('',(0.685937843399239,0.94411244560349,-25.2155475173803));
#22387=CARTESIAN_POINT('',(0.6859379234404,0.9441125563889,-25.10007747308));
#22388=CARTESIAN_POINT('Ctrl Pts',(0.685456475053999,0.943446181037267,
-25.2155263221855));
#22389=CARTESIAN_POINT('Ctrl Pts',(0.753928966560715,0.893908498927705,
-25.2212896399029));
#22390=CARTESIAN_POINT('Ctrl Pts',(0.817137126651638,0.837067423340081,
-25.2270583193288));
#22391=CARTESIAN_POINT('Ctrl Pts',(0.930078955634944,0.710170745214693,
-25.2386648185784));
#22392=CARTESIAN_POINT('Ctrl Pts',(0.978805081969252,0.640771788780588,
-25.244424636746));
#22393=CARTESIAN_POINT('Ctrl Pts',(1.09334014170001,0.432850881490653,-25.260624765588));
#22394=CARTESIAN_POINT('Ctrl Pts',(1.1409083697686,0.284233085157616,-25.2710522198586));
#22395=CARTESIAN_POINT('Ctrl Pts',(1.17695775141982,-0.0212095663597187,
-25.292031044981));
#22396=CARTESIAN_POINT('Ctrl Pts',(1.16412445259043,-0.173935093258059,
-25.302302863744));
#22397=CARTESIAN_POINT('Ctrl Pts',(1.07871456427401,-0.467372055691385,
-25.3231468506275));
#22398=CARTESIAN_POINT('Ctrl Pts',(1.00840900073704,-0.604724253435656,
-25.3334627805692));
#22399=CARTESIAN_POINT('Ctrl Pts',(0.820426902272126,-0.844168464163895,
-25.3542375650593));
#22400=CARTESIAN_POINT('Ctrl Pts',(0.705575432041381,-0.941860126973701,
-25.3643397811048));
#22401=CARTESIAN_POINT('Ctrl Pts',(0.439600076520464,-1.09001309956845,
-25.3850966850864));
#22402=CARTESIAN_POINT('Ctrl Pts',(0.294874600697833,-1.13826266613819,
-25.395302367302));
#22403=CARTESIAN_POINT('Ctrl Pts',(-0.0285175083645314,-1.18025875562043,
-25.4175666426249));
#22404=CARTESIAN_POINT('Ctrl Pts',(-0.182033422095494,-1.1592094749399,
-25.4279248529788));
#22405=CARTESIAN_POINT('Ctrl Pts',(-0.449064049193832,-1.08594237765718,
-25.4467982047514));
#22406=CARTESIAN_POINT('Ctrl Pts',(-0.58473977016012,-1.02017668863555,
-25.4568916601279));
#22407=CARTESIAN_POINT('Ctrl Pts',(-0.847055326004509,-0.823158197369117,
-25.4792958601879));
#22408=CARTESIAN_POINT('Ctrl Pts',(-0.942308301897876,-0.698259145664254,
-25.4897825979083));
#22409=CARTESIAN_POINT('Ctrl Pts',(-1.07952055488772,-0.463955778317708,
-25.5082867322755));
#22410=CARTESIAN_POINT('Ctrl Pts',(-1.1304148005763,-0.32393890122586,-25.5182677916968));
#22411=CARTESIAN_POINT('Ctrl Pts',(-1.18066367741776,-0.00367979153001349,
-25.5404107238414));
#22412=CARTESIAN_POINT('Ctrl Pts',(-1.16276126940395,0.154335596280979,
-25.5510273049907));
#22413=CARTESIAN_POINT('Ctrl Pts',(-1.09762881343295,0.419173795090977,
-25.5696126930082));
#22414=CARTESIAN_POINT('Ctrl Pts',(-1.03737331464878,0.553985095242714,
-25.579512573544));
#22415=CARTESIAN_POINT('Ctrl Pts',(-0.863967323007216,0.799686680741356,
-25.6000550606958));
#22416=CARTESIAN_POINT('Ctrl Pts',(-0.74784111191472,0.907800899737537,
-25.6106622296586));
#22417=CARTESIAN_POINT('Ctrl Pts',(-0.513927950087508,1.05362922373647,
-25.6294473277748));
#22418=CARTESIAN_POINT('Ctrl Pts',(-0.377197010975904,1.11815960801924,
-25.6395560462991));
#22419=CARTESIAN_POINT('Ctrl Pts',(-0.0539287632978119,1.17564040536612,
-25.6619812077133));
#22420=CARTESIAN_POINT('Ctrl Pts',(0.104280046962069,1.17139237118361,-25.6725580530658));
#22421=CARTESIAN_POINT('Ctrl Pts',(0.379417361706695,1.11015017237935,-25.6917705495726));
#22422=CARTESIAN_POINT('Ctrl Pts',(0.522012612882813,1.05825780349353,-25.7019230808369));
#22423=CARTESIAN_POINT('Ctrl Pts',(0.790153055006959,0.871599909795858,
-25.7242292828709));
#22424=CARTESIAN_POINT('Ctrl Pts',(0.899073814666876,0.7579114122043,-25.7347495650281));
#22425=CARTESIAN_POINT('Ctrl Pts',(1.06692428771505,0.497065064247596,-25.7558983763229));
#22426=CARTESIAN_POINT('Ctrl Pts',(1.12133155849896,0.357124825114038,-25.7659604824616));
#22427=CARTESIAN_POINT('Ctrl Pts',(1.17458095923193,0.058055748008961,-25.7866904752754));
#22428=CARTESIAN_POINT('Ctrl Pts',(1.17174004169197,-0.0980896064647793,
-25.7971268139698));
#22429=CARTESIAN_POINT('Ctrl Pts',(1.10748671081373,-0.398813820899846,
-25.8181021416962));
#22430=CARTESIAN_POINT('Ctrl Pts',(1.04632261567736,-0.539166539140376,
-25.8283633413593));
#22431=CARTESIAN_POINT('Ctrl Pts',(0.870908471580301,-0.789694137648766,
-25.849223295225));
#22432=CARTESIAN_POINT('Ctrl Pts',(0.759972011863893,-0.897212591118109,
-25.8595514605356));
#22433=CARTESIAN_POINT('Ctrl Pts',(0.505961314281782,-1.06264952067059,
-25.880238039437));
#22434=CARTESIAN_POINT('Ctrl Pts',(0.366045653279312,-1.11868537462692,
-25.8903371103175));
#22435=CARTESIAN_POINT('Ctrl Pts',(0.0650008832967905,-1.17355187918509,
-25.9112005351713));
#22436=CARTESIAN_POINT('Ctrl Pts',(-0.0877663802010868,-1.17255492774913,
-25.9214196096765));
#22437=CARTESIAN_POINT('Ctrl Pts',(-0.407299221774617,-1.10806100432969,
-25.9436737563468));
#22438=CARTESIAN_POINT('Ctrl Pts',(-0.545695120922654,-1.03888082979981,
-25.9540179844193));
#22439=CARTESIAN_POINT('Ctrl Pts',(-0.775302153215706,-0.883109475340792,
-25.9729300210824));
#22440=CARTESIAN_POINT('Ctrl Pts',(-0.882642823167725,-0.776924872095221,
-25.9830368577589));
#22441=CARTESIAN_POINT('Ctrl Pts',(-1.06716371732725,-0.506049870726424,
-26.0054191523544));
#22442=CARTESIAN_POINT('Ctrl Pts',(-1.11711542772957,-0.357403365460102,
-26.0158902244773));
#22443=CARTESIAN_POINT('Ctrl Pts',(-1.17150698299789,-0.0906683634061106,
-26.0344423045363));
#22444=CARTESIAN_POINT('Ctrl Pts',(-1.17445379308505,0.0584942439088762,
-26.0444366233427));
#22445=CARTESIAN_POINT('Ctrl Pts',(-1.11587167131851,0.393273107848679,
-26.067650805626));
#22446=CARTESIAN_POINT('Ctrl Pts',(-1.04031459198801,0.537652390835965,
-26.0784973022942));
#22447=CARTESIAN_POINT('Ctrl Pts',(-0.903532701937386,0.751044251113647,
-26.0957700105568));
#22448=CARTESIAN_POINT('Ctrl Pts',(-0.803121960948684,0.858973369535563,
-26.1056531858431));
#22449=CARTESIAN_POINT('Ctrl Pts',(-0.568753885931908,1.02925174324195,
-26.1254418679969));
#22450=CARTESIAN_POINT('Ctrl Pts',(-0.435078569175414,1.09139610098497,
-26.1353250432865));
#22451=CARTESIAN_POINT('Ctrl Pts',(-0.18986292138628,1.15554169754148,-26.1525977515492));
#22452=CARTESIAN_POINT('Ctrl Pts',(-0.0292016419244966,1.18278509811256,
-26.1634442482175));
#22453=CARTESIAN_POINT('Ctrl Pts',(0.307294849336613,1.13504764844191,-26.1866584305008));
#22454=CARTESIAN_POINT('Ctrl Pts',(0.448246304615041,1.08615128492058,-26.1966527493071));
#22455=CARTESIAN_POINT('Ctrl Pts',(0.685118451514085,0.951996193221822,
-26.2152048293661));
#22456=CARTESIAN_POINT('Ctrl Pts',(0.811053751559603,0.858554997261884,
-26.2256759014889));
#22457=CARTESIAN_POINT('Ctrl Pts',(1.01165109460014,0.599360219704633,-26.2480581960845));
#22458=CARTESIAN_POINT('Ctrl Pts',(1.07946856224422,0.464460329139464,-26.2581650327611));
#22459=CARTESIAN_POINT('Ctrl Pts',(1.15666344894798,0.197955069125299,-26.2770770694244));
#22460=CARTESIAN_POINT('Ctrl Pts',(1.17969101994448,0.0449548978084111,
-26.287421297497));
#22461=CARTESIAN_POINT('Ctrl Pts',(1.14228730776675,-0.278868611711105,
-26.3096754441672));
#22462=CARTESIAN_POINT('Ctrl Pts',(1.09602778432128,-0.424466988073717,
-26.3198945186723));
#22463=CARTESIAN_POINT('Ctrl Pts',(0.950818687642312,-0.693822895932095,
-26.3407579435259));
#22464=CARTESIAN_POINT('Ctrl Pts',(0.854289106561841,-0.809574565893386,
-26.3508570144063));
#22465=CARTESIAN_POINT('Ctrl Pts',(0.618455614369187,-1.00003027230849,
-26.3715435933077));
#22466=CARTESIAN_POINT('Ctrl Pts',(0.481918237226907,-1.07231208588558,
-26.3818717586183));
#22467=CARTESIAN_POINT('Ctrl Pts',(0.189446380573906,-1.16172356518028,
-26.402731712484));
#22468=CARTESIAN_POINT('Ctrl Pts',(0.0370622684688799,-1.17652270127989,
-26.4129929121471));
#22469=CARTESIAN_POINT('Ctrl Pts',(-0.268798826463713,-1.14470235742468,
-26.4339682398734));
#22470=CARTESIAN_POINT('Ctrl Pts',(-0.418179775124505,-1.09915266243818,
-26.4444045785679));
#22471=CARTESIAN_POINT('Ctrl Pts',(-0.686156399960757,-0.956092045564685,
-26.4651345713817));
#22472=CARTESIAN_POINT('Ctrl Pts',(-0.802434704990725,-0.861103744062606,
-26.4751966775203));
#22473=CARTESIAN_POINT('Ctrl Pts',(-0.998645675280886,-0.620862503467603,
-26.496345488815));
#22474=CARTESIAN_POINT('Ctrl Pts',(-1.07311149596802,-0.482141027412342,
-26.5068657709721));
#22475=CARTESIAN_POINT('Ctrl Pts',(-1.16777374859158,-0.169443851360786,
-26.529171973006));
#22476=CARTESIAN_POINT('Ctrl Pts',(-1.17306196823584,-0.0177920846727423,
-26.5393245042704));
#22477=CARTESIAN_POINT('Ctrl Pts',(-1.146284654438,0.262803931594615,-26.5585370007772));
#22478=CARTESIAN_POINT('Ctrl Pts',(-1.10143556399854,0.414582166282618,
-26.5691138461298));
#22479=CARTESIAN_POINT('Ctrl Pts',(-0.946872694845563,0.704265996517479,
-26.591539007544));
#22480=CARTESIAN_POINT('Ctrl Pts',(-0.843248468532132,0.814363861741629,
-26.6016477260684));
#22481=CARTESIAN_POINT('Ctrl Pts',(-0.632274348520049,0.991765068167514,
-26.6204328241844));
#22482=CARTESIAN_POINT('Ctrl Pts',(-0.493566643319621,1.06879852693624,
-26.6310399931471));
#22483=CARTESIAN_POINT('Ctrl Pts',(-0.206305151023379,1.15779145978755,
-26.6515824802988));
#22484=CARTESIAN_POINT('Ctrl Pts',(-0.059472012414958,1.17343886176815,
-26.6614823608346));
#22485=CARTESIAN_POINT('Ctrl Pts',(0.212531118107488,1.1535440042497,-26.6800677488523));
#22486=CARTESIAN_POINT('Ctrl Pts',(0.368344830676723,1.12174076584227,-26.6906843300017));
#22487=CARTESIAN_POINT('Ctrl Pts',(0.657401586964124,0.974985736585933,
-26.7128272621465));
#22488=CARTESIAN_POINT('Ctrl Pts',(0.774838363480133,0.883314838061018,
-26.722808321568));
#22489=CARTESIAN_POINT('Ctrl Pts',(0.955273189774572,0.680414508389969,
-26.7413124559353));
#22490=CARTESIAN_POINT('Ctrl Pts',(1.04462445846149,0.551227615412156,-26.7517991936558));
#22491=CARTESIAN_POINT('Ctrl Pts',(1.15094021376586,0.240868634693924,-26.7742033937157));
#22492=CARTESIAN_POINT('Ctrl Pts',(1.17156099735573,0.091510640611728,-26.784296849092));
#22493=CARTESIAN_POINT('Ctrl Pts',(1.15872514586447,-0.185091355529303,
-26.8031702008644));
#22494=CARTESIAN_POINT('Ctrl Pts',(1.13130517516905,-0.337598251087985,
-26.8135284112181));
#22495=CARTESIAN_POINT('Ctrl Pts',(0.991430863060781,-0.632184918383263,
-26.8357926865412));
#22496=CARTESIAN_POINT('Ctrl Pts',(0.900820166817858,-0.754917089197195,
-26.8459983687569));
#22497=CARTESIAN_POINT('Ctrl Pts',(0.677727411882154,-0.962092897940218,
-26.8667552727386));
#22498=CARTESIAN_POINT('Ctrl Pts',(0.549326063249094,-1.04113475309212,
-26.8768574887843));
#22499=CARTESIAN_POINT('Ctrl Pts',(0.263511423283125,-1.14592402246405,
-26.8976322732743));
#22500=CARTESIAN_POINT('Ctrl Pts',(0.111156106659097,-1.17034442347985,
-26.9079482032157));
#22501=CARTESIAN_POINT('Ctrl Pts',(-0.194312135562308,-1.16089704614949,
-26.9287921900991));
#22502=CARTESIAN_POINT('Ctrl Pts',(-0.343528450555829,-1.12590745534024,
-26.939064008862));
#22503=CARTESIAN_POINT('Ctrl Pts',(-0.622881803069089,-0.997235485886526,
-26.9600428339845));
#22504=CARTESIAN_POINT('Ctrl Pts',(-0.749526335843654,-0.906069987879729,
-26.9704702882552));
#22505=CARTESIAN_POINT('Ctrl Pts',(-0.911877589686957,-0.732889579140318,
-26.9866704170972));
#22506=CARTESIAN_POINT('Ctrl Pts',(-0.962822718320104,-0.665102822246633,
-26.9924302352649));
#22507=CARTESIAN_POINT('Ctrl Pts',(-1.04860765672717,-0.518475580504917,
-27.0040367304977));
#22508=CARTESIAN_POINT('Ctrl Pts',(-1.08313431805629,-0.440796246967627,
-27.009805405914));
#22509=CARTESIAN_POINT('Ctrl Pts',(-1.10908828377811,-0.360367111878606,
-27.0155687196296));
#22510=CARTESIAN_POINT('Ctrl Pts',(0.685456617960072,0.943446077649226,
-25.1000562803705));
#22511=CARTESIAN_POINT('Ctrl Pts',(0.75392905450701,0.893908419840442,-25.1058195940861));
#22512=CARTESIAN_POINT('Ctrl Pts',(0.817137165739417,0.837067379422799,
-25.1115882695023));
#22513=CARTESIAN_POINT('Ctrl Pts',(0.930078955635281,0.710170745214216,
-25.1231947647351));
#22514=CARTESIAN_POINT('Ctrl Pts',(0.978805081969397,0.640771788780325,
-25.1289545829027));
#22515=CARTESIAN_POINT('Ctrl Pts',(1.09334014170002,0.432850881490647,-25.1451547117447));
#22516=CARTESIAN_POINT('Ctrl Pts',(1.1409083697686,0.284233085157607,-25.1555821660154));
#22517=CARTESIAN_POINT('Ctrl Pts',(1.17695775141982,-0.0212095663597268,
-25.1765609911379));
#22518=CARTESIAN_POINT('Ctrl Pts',(1.16412445259043,-0.173935093258066,
-25.1868328099009));
#22519=CARTESIAN_POINT('Ctrl Pts',(1.07871456427401,-0.46737205569139,-25.2076767967844));
#22520=CARTESIAN_POINT('Ctrl Pts',(1.00840900073704,-0.60472425343566,-25.217992726726));
#22521=CARTESIAN_POINT('Ctrl Pts',(0.820426902272119,-0.844168464163902,
-25.238767511216));
#22522=CARTESIAN_POINT('Ctrl Pts',(0.705575432041372,-0.941860126973706,
-25.2488697272616));
#22523=CARTESIAN_POINT('Ctrl Pts',(0.439600076520457,-1.09001309956845,
-25.2696266312433));
#22524=CARTESIAN_POINT('Ctrl Pts',(0.294874600697824,-1.13826266613819,
-25.2798323134589));
#22525=CARTESIAN_POINT('Ctrl Pts',(-0.0285175083645393,-1.18025875562043,
-25.3020965887819));
#22526=CARTESIAN_POINT('Ctrl Pts',(-0.182033422095502,-1.1592094749399,
-25.3124547991358));
#22527=CARTESIAN_POINT('Ctrl Pts',(-0.449064049193836,-1.08594237765718,
-25.3313281509083));
#22528=CARTESIAN_POINT('Ctrl Pts',(-0.584739770160119,-1.02017668863555,
-25.3414216062847));
#22529=CARTESIAN_POINT('Ctrl Pts',(-0.847055326004502,-0.823158197369123,
-25.3638258063445));
#22530=CARTESIAN_POINT('Ctrl Pts',(-0.942308301897868,-0.698259145664264,
-25.3743125440648));
#22531=CARTESIAN_POINT('Ctrl Pts',(-1.07952055488771,-0.463955778317722,
-25.392816678432));
#22532=CARTESIAN_POINT('Ctrl Pts',(-1.1304148005763,-0.323938901225872,
-25.4027977378532));
#22533=CARTESIAN_POINT('Ctrl Pts',(-1.18066367741776,-0.00367979152997945,
-25.4249406699978));
#22534=CARTESIAN_POINT('Ctrl Pts',(-1.16276126940394,0.154335596281021,
-25.4355572511473));
#22535=CARTESIAN_POINT('Ctrl Pts',(-1.09762881343295,0.419173795090975,
-25.4541426391649));
#22536=CARTESIAN_POINT('Ctrl Pts',(-1.03737331464878,0.553985095242714,
-25.4640425197008));
#22537=CARTESIAN_POINT('Ctrl Pts',(-0.863967323007212,0.799686680741361,
-25.4845850068527));
#22538=CARTESIAN_POINT('Ctrl Pts',(-0.747841111914714,0.907800899737542,
-25.4951921758154));
#22539=CARTESIAN_POINT('Ctrl Pts',(-0.513927950087493,1.05362922373647,
-25.5139772739317));
#22540=CARTESIAN_POINT('Ctrl Pts',(-0.377197010975882,1.11815960801925,
-25.5240859924561));
#22541=CARTESIAN_POINT('Ctrl Pts',(-0.0539287632977854,1.17564040536612,
-25.5465111538705));
#22542=CARTESIAN_POINT('Ctrl Pts',(0.104280046962098,1.1713923711836,-25.5570879992231));
#22543=CARTESIAN_POINT('Ctrl Pts',(0.37941736170672,1.11015017237934,-25.5763004957299));
#22544=CARTESIAN_POINT('Ctrl Pts',(0.522012612882833,1.05825780349352,-25.5864530269942));
#22545=CARTESIAN_POINT('Ctrl Pts',(0.790153055006974,0.871599909795844,
-25.608759229028));
#22546=CARTESIAN_POINT('Ctrl Pts',(0.899073814666888,0.757911412204285,
-25.6192795111851));
#22547=CARTESIAN_POINT('Ctrl Pts',(1.06692428771506,0.497065064247585,-25.6404283224799));
#22548=CARTESIAN_POINT('Ctrl Pts',(1.12133155849896,0.357124825114025,-25.6504904286186));
#22549=CARTESIAN_POINT('Ctrl Pts',(1.17458095923193,0.0580557480089442,
-25.6712204214325));
#22550=CARTESIAN_POINT('Ctrl Pts',(1.17174004169196,-0.0980896064647949,
-25.6816567601269));
#22551=CARTESIAN_POINT('Ctrl Pts',(1.10748671081372,-0.398813820899856,
-25.7026320878532));
#22552=CARTESIAN_POINT('Ctrl Pts',(1.04632261567736,-0.539166539140384,
-25.7128932875163));
#22553=CARTESIAN_POINT('Ctrl Pts',(0.870908471580299,-0.789694137648768,
-25.7337532413819));
#22554=CARTESIAN_POINT('Ctrl Pts',(0.759972011863892,-0.897212591118109,
-25.7440814066925));
#22555=CARTESIAN_POINT('Ctrl Pts',(0.50596131428179,-1.06264952067058,-25.7647679855938));
#22556=CARTESIAN_POINT('Ctrl Pts',(0.366045653279324,-1.11868537462692,
-25.7748670564742));
#22557=CARTESIAN_POINT('Ctrl Pts',(0.0650008832968025,-1.17355187918509,
-25.7957304813279));
#22558=CARTESIAN_POINT('Ctrl Pts',(-0.0877663802010743,-1.17255492774913,
-25.8059495558329));
#22559=CARTESIAN_POINT('Ctrl Pts',(-0.407299221774608,-1.10806100432969,
-25.8282037025031));
#22560=CARTESIAN_POINT('Ctrl Pts',(-0.545695120922647,-1.03888082979981,
-25.8385479305757));
#22561=CARTESIAN_POINT('Ctrl Pts',(-0.7753021532157,-0.883109475340797,
-25.857459967239));
#22562=CARTESIAN_POINT('Ctrl Pts',(-0.882642823167722,-0.776924872095225,
-25.8675668039156));
#22563=CARTESIAN_POINT('Ctrl Pts',(-1.06716371732725,-0.506049870726427,
-25.8899490985112));
#22564=CARTESIAN_POINT('Ctrl Pts',(-1.11711542772957,-0.357403365460107,
-25.9004201706339));
#22565=CARTESIAN_POINT('Ctrl Pts',(-1.17150698299789,-0.090668363406114,
-25.9189722506929));
#22566=CARTESIAN_POINT('Ctrl Pts',(-1.17445379308505,0.0584942439088722,
-25.9289665694992));
#22567=CARTESIAN_POINT('Ctrl Pts',(-1.11587167131851,0.393273107848691,
-25.9521807517825));
#22568=CARTESIAN_POINT('Ctrl Pts',(-1.040314591988,0.537652390835977,-25.9630272484508));
#22569=CARTESIAN_POINT('Ctrl Pts',(-0.903532701937388,0.751044251113644,
-25.9802999567134));
#22570=CARTESIAN_POINT('Ctrl Pts',(-0.803121960948686,0.858973369535562,
-25.9901831320031));
#22571=CARTESIAN_POINT('Ctrl Pts',(-0.568753885931907,1.02925174324195,
-26.0099718141569));
#22572=CARTESIAN_POINT('Ctrl Pts',(-0.435078569175412,1.09139610098497,
-26.0198549894432));
#22573=CARTESIAN_POINT('Ctrl Pts',(-0.189862921386252,1.15554169754149,
-26.0371276977058));
#22574=CARTESIAN_POINT('Ctrl Pts',(-0.0292016419244725,1.18278509811255,
-26.047974194374));
#22575=CARTESIAN_POINT('Ctrl Pts',(0.307294849336617,1.13504764844191,-26.0711883766573));
#22576=CARTESIAN_POINT('Ctrl Pts',(0.448246304615045,1.08615128492058,-26.0811826954637));
#22577=CARTESIAN_POINT('Ctrl Pts',(0.685118451514086,0.951996193221821,
-26.0997347755227));
#22578=CARTESIAN_POINT('Ctrl Pts',(0.811053751559604,0.858554997261884,
-26.1102058476456));
#22579=CARTESIAN_POINT('Ctrl Pts',(1.01165109460013,0.599360219704635,-26.1325881422411));
#22580=CARTESIAN_POINT('Ctrl Pts',(1.07946856224422,0.46446032913947,-26.1426949789175));
#22581=CARTESIAN_POINT('Ctrl Pts',(1.15666344894798,0.197955069125303,-26.1616070155807));
#22582=CARTESIAN_POINT('Ctrl Pts',(1.17969101994448,0.0449548978084168,
-26.1719512436532));
#22583=CARTESIAN_POINT('Ctrl Pts',(1.14228730776675,-0.278868611711097,
-26.1942053903234));
#22584=CARTESIAN_POINT('Ctrl Pts',(1.09602778432128,-0.42446698807371,-26.2044244648286));
#22585=CARTESIAN_POINT('Ctrl Pts',(0.950818687642318,-0.693822895932088,
-26.2252878896824));
#22586=CARTESIAN_POINT('Ctrl Pts',(0.854289106561847,-0.809574565893382,
-26.235386960563));
#22587=CARTESIAN_POINT('Ctrl Pts',(0.618455614369189,-1.00003027230849,
-26.2560735394644));
#22588=CARTESIAN_POINT('Ctrl Pts',(0.48191823722691,-1.07231208588558,-26.2664017047749));
#22589=CARTESIAN_POINT('Ctrl Pts',(0.189446380573901,-1.16172356518028,
-26.2872616586406));
#22590=CARTESIAN_POINT('Ctrl Pts',(0.0370622684688708,-1.17652270127989,
-26.2975228583036));
#22591=CARTESIAN_POINT('Ctrl Pts',(-0.268798826463742,-1.14470235742468,
-26.3184981860299));
#22592=CARTESIAN_POINT('Ctrl Pts',(-0.418179775124553,-1.09915266243818,
-26.3289345247243));
#22593=CARTESIAN_POINT('Ctrl Pts',(-0.686156399960817,-0.95609204556468,
-26.3496645175382));
#22594=CARTESIAN_POINT('Ctrl Pts',(-0.802434704990775,-0.861103744062606,
-26.3597266236769));
#22595=CARTESIAN_POINT('Ctrl Pts',(-0.99864567528091,-0.620862503467622,
-26.3808754349718));
#22596=CARTESIAN_POINT('Ctrl Pts',(-1.07311149596802,-0.482141027412377,
-26.391395717129));
#22597=CARTESIAN_POINT('Ctrl Pts',(-1.16777374859159,-0.169443851360826,
-26.413701919163));
#22598=CARTESIAN_POINT('Ctrl Pts',(-1.17306196823585,-0.0177920846727685,
-26.4238544504273));
#22599=CARTESIAN_POINT('Ctrl Pts',(-1.146284654438,0.262803931594613,-26.443066946934));
#22600=CARTESIAN_POINT('Ctrl Pts',(-1.10143556399854,0.414582166282623,
-26.4536437922865));
#22601=CARTESIAN_POINT('Ctrl Pts',(-0.946872694845556,0.704265996517489,
-26.4760689537007));
#22602=CARTESIAN_POINT('Ctrl Pts',(-0.843248468532123,0.814363861741638,
-26.4861776722252));
#22603=CARTESIAN_POINT('Ctrl Pts',(-0.632274348520029,0.991765068167528,
-26.5049627703415));
#22604=CARTESIAN_POINT('Ctrl Pts',(-0.493566643319589,1.06879852693625,
-26.5155699393044));
#22605=CARTESIAN_POINT('Ctrl Pts',(-0.206305151023333,1.15779145978756,
-26.5361124264564));
#22606=CARTESIAN_POINT('Ctrl Pts',(-0.0594720124149067,1.17343886176816,
-26.5460123069922));
#22607=CARTESIAN_POINT('Ctrl Pts',(0.212531118107504,1.15354400424969,-26.5645976950098));
#22608=CARTESIAN_POINT('Ctrl Pts',(0.368344830676736,1.12174076584227,-26.5752142761591));
#22609=CARTESIAN_POINT('Ctrl Pts',(0.657401586964147,0.974985736585916,
-26.5973572083036));
#22610=CARTESIAN_POINT('Ctrl Pts',(0.774838363480147,0.883314838061005,
-26.6073382677247));
#22611=CARTESIAN_POINT('Ctrl Pts',(0.955273189774578,0.680414508389961,
-26.6258424020917));
#22612=CARTESIAN_POINT('Ctrl Pts',(1.04462445846149,0.551227615412151,-26.6363291398119));
#22613=CARTESIAN_POINT('Ctrl Pts',(1.15094021376586,0.240868634693926,-26.6587333398718));
#22614=CARTESIAN_POINT('Ctrl Pts',(1.17156099735573,0.0915106406117304,
-26.6688267952484));
#22615=CARTESIAN_POINT('Ctrl Pts',(1.15872514586447,-0.185091355529294,
-26.687700147021));
#22616=CARTESIAN_POINT('Ctrl Pts',(1.13130517516905,-0.33759825108798,-26.698058357375));
#22617=CARTESIAN_POINT('Ctrl Pts',(0.991430863060781,-0.632184918383261,
-26.720322632698));
#22618=CARTESIAN_POINT('Ctrl Pts',(0.90082016681786,-0.754917089197193,
-26.7305283149135));
#22619=CARTESIAN_POINT('Ctrl Pts',(0.677727411882152,-0.96209289794022,
-26.7512852188951));
#22620=CARTESIAN_POINT('Ctrl Pts',(0.549326063249092,-1.04113475309212,
-26.7613874349405));
#22621=CARTESIAN_POINT('Ctrl Pts',(0.263511423283129,-1.14592402246405,
-26.7821622194306));
#22622=CARTESIAN_POINT('Ctrl Pts',(0.111156106659096,-1.17034442347985,
-26.7924781493724));
#22623=CARTESIAN_POINT('Ctrl Pts',(-0.194312135562315,-1.16089704614949,
-26.813322136256));
#22624=CARTESIAN_POINT('Ctrl Pts',(-0.343528450555845,-1.12590745534024,
-26.8235939550191));
#22625=CARTESIAN_POINT('Ctrl Pts',(-0.622881803069112,-0.997235485886511,
-26.8445727801415));
#22626=CARTESIAN_POINT('Ctrl Pts',(-0.749526335843675,-0.906069987879712,
-26.8550002344121));
#22627=CARTESIAN_POINT('Ctrl Pts',(-0.911877589687278,-0.732889579139973,
-26.8712003632541));
#22628=CARTESIAN_POINT('Ctrl Pts',(-0.962822718320643,-0.665102822245911,
-26.8769601814217));
#22629=CARTESIAN_POINT('Ctrl Pts',(-1.04860768641633,-0.51847552975876,
-26.8885666806712));
#22630=CARTESIAN_POINT('Ctrl Pts',(-1.08313436609589,-0.440796138886276,
-26.8943353600971));
#22631=CARTESIAN_POINT('Ctrl Pts',(-1.10908833794558,-0.360366944018197,
-26.9000986778144));
#22632=CARTESIAN_POINT('Ctrl Pts',(0.5101085474843,-1.049594504429,-23.22357429354));
#22633=CARTESIAN_POINT('Ctrl Pts',(0.2529114735039,-1.174593659124,-23.24307429354));
#22634=CARTESIAN_POINT('Ctrl Pts',(-0.3560404579669,-1.226109782198,-23.28207429354));
#22635=CARTESIAN_POINT('Ctrl Pts',(-1.086700069569,-0.6706284754496,-23.34057429354));
#22636=CARTESIAN_POINT('Ctrl Pts',(-1.255757769843,0.2313909492768,-23.39907429354));
#22637=CARTESIAN_POINT('Ctrl Pts',(-0.776277226745,1.013853625323,-23.45757429354));
#22638=CARTESIAN_POINT('Ctrl Pts',(0.1041850635563,1.27265480968,-23.51607429354));
#22639=CARTESIAN_POINT('Ctrl Pts',(0.930828216589,0.8741060067922,-23.57457429354));
#22640=CARTESIAN_POINT('Ctrl Pts',(1.276684843607,0.02406782860266,-23.63307429354));
#22641=CARTESIAN_POINT('Ctrl Pts',(0.9631123225395,-0.8384019827806,-23.69157429354));
#22642=CARTESIAN_POINT('Ctrl Pts',(0.1520765516308,-1.267823319973,-23.75007429354));
#22643=CARTESIAN_POINT('Ctrl Pts',(-0.737509290634,-1.042393065597,-23.80857429354));
#22644=CARTESIAN_POINT('Ctrl Pts',(-1.24615944086,-0.2785496368411,-23.86707429354));
#22645=CARTESIAN_POINT('Ctrl Pts',(-1.111147737084,0.6291692616945,-23.92557429354));
#22646=CARTESIAN_POINT('Ctrl Pts',(-0.4022099431193,1.211911884167,-23.98407429354));
#22647=CARTESIAN_POINT('Ctrl Pts',(0.5144759044836,1.16868207696,-24.04257429354));
#22648=CARTESIAN_POINT('Ctrl Pts',(1.165426482007,0.5218087469177,-24.10107429354));
#22649=CARTESIAN_POINT('Ctrl Pts',(1.214415105026,-0.3945873870257,-24.15957429354));
#22650=CARTESIAN_POINT('Ctrl Pts',(0.6361383436829,-1.107172642825,-24.21807429354));
#22651=CARTESIAN_POINT('Ctrl Pts',(-0.2707143395318,-1.247885010597,-24.27657429354));
#22652=CARTESIAN_POINT('Ctrl Pts',(-1.037738611881,-0.7440442370847,-24.33507429354));
#22653=CARTESIAN_POINT('Ctrl Pts',(-1.268753815782,0.1441076279268,-24.39357429354));
#22654=CARTESIAN_POINT('Ctrl Pts',(-0.8444367967899,0.957825531324,-24.45207429354));
#22655=CARTESIAN_POINT('Ctrl Pts',(0.01604572141757,1.27681078935,-24.51057429354));
#22656=CARTESIAN_POINT('Ctrl Pts',(0.868240364708,0.9363022574552,-24.56907429354));
#22657=CARTESIAN_POINT('Ctrl Pts',(1.271974557398,0.1121782326973,-24.62757429354));
#22658=CARTESIAN_POINT('Ctrl Pts',(1.018713020232,-0.7698878052547,-24.68607429354));
#22659=CARTESIAN_POINT('Ctrl Pts',(0.2392692263315,-1.254293712509,-24.74457429354));
#22660=CARTESIAN_POINT('Ctrl Pts',(-0.6637602414119,-1.090837812872,-24.80307429354));
#22661=CARTESIAN_POINT('Ctrl Pts',(-1.223949677731,-0.3639405071239,-24.86157429354));
#22662=CARTESIAN_POINT('Ctrl Pts',(-1.151937564121,0.5509166872562,-24.92007429354));
#22663=CARTESIAN_POINT('Ctrl Pts',(-0.4849732964329,1.181296108108,-24.97857429354));
#22664=CARTESIAN_POINT('Ctrl Pts',(0.4326464664874,1.20121898118,-25.03707429354));
#22665=CARTESIAN_POINT('Ctrl Pts',(0.8950185104062,0.8016085974549,-25.07607429354));
#22666=CARTESIAN_POINT('Ctrl Pts',(1.029622654482,0.5493055100063,-25.09557429354));
#22667=CARTESIAN_POINT('Ctrl Pts',(0.5101085474843,-1.049594504429,-23.28906643118));
#22668=CARTESIAN_POINT('Ctrl Pts',(0.2529114735039,-1.174593659124,-23.30856643118));
#22669=CARTESIAN_POINT('Ctrl Pts',(-0.3560404579669,-1.226109782198,-23.34756643118));
#22670=CARTESIAN_POINT('Ctrl Pts',(-1.086700069569,-0.6706284754496,-23.40606643118));
#22671=CARTESIAN_POINT('Ctrl Pts',(-1.255757769843,0.2313909492768,-23.46456643118));
#22672=CARTESIAN_POINT('Ctrl Pts',(-0.776277226745,1.013853625323,-23.52306643118));
#22673=CARTESIAN_POINT('Ctrl Pts',(0.1041850635563,1.27265480968,-23.58156643118));
#22674=CARTESIAN_POINT('Ctrl Pts',(0.930828216589,0.8741060067922,-23.64006643118));
#22675=CARTESIAN_POINT('Ctrl Pts',(1.276684843607,0.02406782860266,-23.69856643118));
#22676=CARTESIAN_POINT('Ctrl Pts',(0.9631123225395,-0.8384019827806,-23.75706643118));
#22677=CARTESIAN_POINT('Ctrl Pts',(0.1520765516308,-1.267823319973,-23.81556643118));
#22678=CARTESIAN_POINT('Ctrl Pts',(-0.737509290634,-1.042393065597,-23.87406643118));
#22679=CARTESIAN_POINT('Ctrl Pts',(-1.24615944086,-0.2785496368411,-23.93256643118));
#22680=CARTESIAN_POINT('Ctrl Pts',(-1.111147737084,0.6291692616945,-23.99106643118));
#22681=CARTESIAN_POINT('Ctrl Pts',(-0.4022099431193,1.211911884167,-24.04956643118));
#22682=CARTESIAN_POINT('Ctrl Pts',(0.5144759044836,1.16868207696,-24.10806643118));
#22683=CARTESIAN_POINT('Ctrl Pts',(1.165426482007,0.5218087469177,-24.16656643118));
#22684=CARTESIAN_POINT('Ctrl Pts',(1.214415105026,-0.3945873870257,-24.22506643118));
#22685=CARTESIAN_POINT('Ctrl Pts',(0.6361383436829,-1.107172642825,-24.28356643118));
#22686=CARTESIAN_POINT('Ctrl Pts',(-0.2707143395318,-1.247885010597,-24.34206643118));
#22687=CARTESIAN_POINT('Ctrl Pts',(-1.037738611881,-0.7440442370847,-24.40056643118));
#22688=CARTESIAN_POINT('Ctrl Pts',(-1.268753815782,0.1441076279268,-24.45906643118));
#22689=CARTESIAN_POINT('Ctrl Pts',(-0.8444367967899,0.957825531324,-24.51756643118));
#22690=CARTESIAN_POINT('Ctrl Pts',(0.01604572141757,1.27681078935,-24.57606643118));
#22691=CARTESIAN_POINT('Ctrl Pts',(0.868240364708,0.9363022574552,-24.63456643118));
#22692=CARTESIAN_POINT('Ctrl Pts',(1.271974557398,0.1121782326973,-24.69306643118));
#22693=CARTESIAN_POINT('Ctrl Pts',(1.018713020232,-0.7698878052547,-24.75156643118));
#22694=CARTESIAN_POINT('Ctrl Pts',(0.2392692263315,-1.254293712509,-24.81006643118));
#22695=CARTESIAN_POINT('Ctrl Pts',(-0.6637602414119,-1.090837812872,-24.86856643118));
#22696=CARTESIAN_POINT('Ctrl Pts',(-1.223949677731,-0.3639405071239,-24.92706643118));
#22697=CARTESIAN_POINT('Ctrl Pts',(-1.151937564121,0.5509166872562,-24.98556643118));
#22698=CARTESIAN_POINT('Ctrl Pts',(-0.4849732964329,1.181296108108,-25.04406643118));
#22699=CARTESIAN_POINT('Ctrl Pts',(0.4326464664874,1.20121898118,-25.10256643118));
#22700=CARTESIAN_POINT('Ctrl Pts',(0.8950185104062,0.8016085974549,-25.14156643118));
#22701=CARTESIAN_POINT('Ctrl Pts',(1.029622654482,0.5493055100063,-25.16106643118));
#22702=CARTESIAN_POINT('Ctrl Pts',(0.5101085474843,-1.049594504429,-23.35455856882));
#22703=CARTESIAN_POINT('Ctrl Pts',(0.2529114735039,-1.174593659124,-23.37405856882));
#22704=CARTESIAN_POINT('Ctrl Pts',(-0.3560404579669,-1.226109782198,-23.41305856882));
#22705=CARTESIAN_POINT('Ctrl Pts',(-1.086700069569,-0.6706284754496,-23.47155856882));
#22706=CARTESIAN_POINT('Ctrl Pts',(-1.255757769843,0.2313909492768,-23.53005856882));
#22707=CARTESIAN_POINT('Ctrl Pts',(-0.776277226745,1.013853625323,-23.58855856882));
#22708=CARTESIAN_POINT('Ctrl Pts',(0.1041850635563,1.27265480968,-23.64705856882));
#22709=CARTESIAN_POINT('Ctrl Pts',(0.930828216589,0.8741060067922,-23.70555856882));
#22710=CARTESIAN_POINT('Ctrl Pts',(1.276684843607,0.02406782860266,-23.76405856882));
#22711=CARTESIAN_POINT('Ctrl Pts',(0.9631123225395,-0.8384019827806,-23.82255856882));
#22712=CARTESIAN_POINT('Ctrl Pts',(0.1520765516308,-1.267823319973,-23.88105856882));
#22713=CARTESIAN_POINT('Ctrl Pts',(-0.737509290634,-1.042393065597,-23.93955856882));
#22714=CARTESIAN_POINT('Ctrl Pts',(-1.24615944086,-0.2785496368411,-23.99805856882));
#22715=CARTESIAN_POINT('Ctrl Pts',(-1.111147737084,0.6291692616945,-24.05655856882));
#22716=CARTESIAN_POINT('Ctrl Pts',(-0.4022099431193,1.211911884167,-24.11505856882));
#22717=CARTESIAN_POINT('Ctrl Pts',(0.5144759044836,1.16868207696,-24.17355856882));
#22718=CARTESIAN_POINT('Ctrl Pts',(1.165426482007,0.5218087469177,-24.23205856882));
#22719=CARTESIAN_POINT('Ctrl Pts',(1.214415105026,-0.3945873870257,-24.29055856882));
#22720=CARTESIAN_POINT('Ctrl Pts',(0.6361383436829,-1.107172642825,-24.34905856882));
#22721=CARTESIAN_POINT('Ctrl Pts',(-0.2707143395318,-1.247885010597,-24.40755856882));
#22722=CARTESIAN_POINT('Ctrl Pts',(-1.037738611881,-0.7440442370847,-24.46605856882));
#22723=CARTESIAN_POINT('Ctrl Pts',(-1.268753815782,0.1441076279268,-24.52455856882));
#22724=CARTESIAN_POINT('Ctrl Pts',(-0.8444367967899,0.957825531324,-24.58305856882));
#22725=CARTESIAN_POINT('Ctrl Pts',(0.01604572141757,1.27681078935,-24.64155856882));
#22726=CARTESIAN_POINT('Ctrl Pts',(0.868240364708,0.9363022574552,-24.70005856882));
#22727=CARTESIAN_POINT('Ctrl Pts',(1.271974557398,0.1121782326973,-24.75855856882));
#22728=CARTESIAN_POINT('Ctrl Pts',(1.018713020232,-0.7698878052547,-24.81705856882));
#22729=CARTESIAN_POINT('Ctrl Pts',(0.2392692263315,-1.254293712509,-24.87555856882));
#22730=CARTESIAN_POINT('Ctrl Pts',(-0.6637602414119,-1.090837812872,-24.93405856882));
#22731=CARTESIAN_POINT('Ctrl Pts',(-1.223949677731,-0.3639405071239,-24.99255856882));
#22732=CARTESIAN_POINT('Ctrl Pts',(-1.151937564121,0.5509166872562,-25.05105856882));
#22733=CARTESIAN_POINT('Ctrl Pts',(-0.4849732964329,1.181296108108,-25.10955856882));
#22734=CARTESIAN_POINT('Ctrl Pts',(0.4326464664874,1.20121898118,-25.16805856882));
#22735=CARTESIAN_POINT('Ctrl Pts',(0.8950185104062,0.8016085974549,-25.20705856882));
#22736=CARTESIAN_POINT('Ctrl Pts',(1.029622654482,0.5493055100063,-25.22655856882));
#22737=CARTESIAN_POINT('Ctrl Pts',(0.5101085474843,-1.049594504429,-23.42005070646));
#22738=CARTESIAN_POINT('Ctrl Pts',(0.2529114735039,-1.174593659124,-23.43955070646));
#22739=CARTESIAN_POINT('Ctrl Pts',(-0.3560404579669,-1.226109782198,-23.47855070646));
#22740=CARTESIAN_POINT('Ctrl Pts',(-1.086700069569,-0.6706284754496,-23.53705070646));
#22741=CARTESIAN_POINT('Ctrl Pts',(-1.255757769843,0.2313909492768,-23.59555070646));
#22742=CARTESIAN_POINT('Ctrl Pts',(-0.776277226745,1.013853625323,-23.65405070646));
#22743=CARTESIAN_POINT('Ctrl Pts',(0.1041850635563,1.27265480968,-23.71255070646));
#22744=CARTESIAN_POINT('Ctrl Pts',(0.930828216589,0.8741060067922,-23.77105070646));
#22745=CARTESIAN_POINT('Ctrl Pts',(1.276684843607,0.02406782860266,-23.82955070646));
#22746=CARTESIAN_POINT('Ctrl Pts',(0.9631123225395,-0.8384019827806,-23.88805070646));
#22747=CARTESIAN_POINT('Ctrl Pts',(0.1520765516308,-1.267823319973,-23.94655070646));
#22748=CARTESIAN_POINT('Ctrl Pts',(-0.737509290634,-1.042393065597,-24.00505070646));
#22749=CARTESIAN_POINT('Ctrl Pts',(-1.24615944086,-0.2785496368411,-24.06355070646));
#22750=CARTESIAN_POINT('Ctrl Pts',(-1.111147737084,0.6291692616945,-24.12205070646));
#22751=CARTESIAN_POINT('Ctrl Pts',(-0.4022099431193,1.211911884167,-24.18055070646));
#22752=CARTESIAN_POINT('Ctrl Pts',(0.5144759044836,1.16868207696,-24.23905070646));
#22753=CARTESIAN_POINT('Ctrl Pts',(1.165426482007,0.5218087469177,-24.29755070646));
#22754=CARTESIAN_POINT('Ctrl Pts',(1.214415105026,-0.3945873870257,-24.35605070646));
#22755=CARTESIAN_POINT('Ctrl Pts',(0.6361383436829,-1.107172642825,-24.41455070646));
#22756=CARTESIAN_POINT('Ctrl Pts',(-0.2707143395318,-1.247885010597,-24.47305070646));
#22757=CARTESIAN_POINT('Ctrl Pts',(-1.037738611881,-0.7440442370847,-24.53155070646));
#22758=CARTESIAN_POINT('Ctrl Pts',(-1.268753815782,0.1441076279268,-24.59005070646));
#22759=CARTESIAN_POINT('Ctrl Pts',(-0.8444367967899,0.957825531324,-24.64855070646));
#22760=CARTESIAN_POINT('Ctrl Pts',(0.01604572141757,1.27681078935,-24.70705070646));
#22761=CARTESIAN_POINT('Ctrl Pts',(0.868240364708,0.9363022574552,-24.76555070646));
#22762=CARTESIAN_POINT('Ctrl Pts',(1.271974557398,0.1121782326973,-24.82405070646));
#22763=CARTESIAN_POINT('Ctrl Pts',(1.018713020232,-0.7698878052547,-24.88255070646));
#22764=CARTESIAN_POINT('Ctrl Pts',(0.2392692263315,-1.254293712509,-24.94105070646));
#22765=CARTESIAN_POINT('Ctrl Pts',(-0.6637602414119,-1.090837812872,-24.99955070646));
#22766=CARTESIAN_POINT('Ctrl Pts',(-1.223949677731,-0.3639405071239,-25.05805070646));
#22767=CARTESIAN_POINT('Ctrl Pts',(-1.151937564121,0.5509166872562,-25.11655070646));
#22768=CARTESIAN_POINT('Ctrl Pts',(-0.4849732964329,1.181296108108,-25.17505070646));
#22769=CARTESIAN_POINT('Ctrl Pts',(0.4326464664874,1.20121898118,-25.23355070646));
#22770=CARTESIAN_POINT('Ctrl Pts',(0.8950185104062,0.8016085974549,-25.27255070646));
#22771=CARTESIAN_POINT('Ctrl Pts',(1.029622654482,0.5493055100063,-25.29205070646));
#22772=CARTESIAN_POINT('',(7.7598198018898E-11,-1.1661651967976,-23.3000561186915));
#22773=CARTESIAN_POINT('',(-8.83583665353582E-11,-1.16616519683289,-23.4155261737951));
#22774=CARTESIAN_POINT('Ctrl Pts',(5.00307097096597E-18,-1.16616519645645,
-23.3000561186915));
#22775=CARTESIAN_POINT('Ctrl Pts',(2.42851199960663E-16,-1.16616519645645,
-23.3193082457943));
#22776=CARTESIAN_POINT('Ctrl Pts',(8.88178419700125E-15,-1.16616519645645,
-23.3385603728972));
#22777=CARTESIAN_POINT('Ctrl Pts',(8.88178419700125E-15,-1.16616519645645,
-23.377050391265));
#22778=CARTESIAN_POINT('Ctrl Pts',(2.5533440660903E-16,-1.16616519645645,
-23.3962882825301));
#22779=CARTESIAN_POINT('Ctrl Pts',(5.53195026095858E-18,-1.16616519645645,
-23.4155261737951));
#22780=CARTESIAN_POINT('Ctrl Pts',(-1.33558877062777E-10,-1.16616519645672,
-23.4155261731434));
#22781=CARTESIAN_POINT('Ctrl Pts',(-0.0845144697814676,-1.1663356487857,
-23.4212895959207));
#22782=CARTESIAN_POINT('Ctrl Pts',(-0.169062851789874,-1.15750290857422,
-23.4270583806262));
#22783=CARTESIAN_POINT('Ctrl Pts',(-0.335023329548445,-1.12122637131796,
-23.4386649290137));
#22784=CARTESIAN_POINT('Ctrl Pts',(-0.415234485903957,-1.09372210750977,
-23.4444246931359));
#22785=CARTESIAN_POINT('Ctrl Pts',(-0.630107390685444,-0.992832930186848,
-23.4606247655878));
#22786=CARTESIAN_POINT('Ctrl Pts',(-0.75594624449798,-0.900558510223427,
-23.4710522198585));
#22787=CARTESIAN_POINT('Ctrl Pts',(-0.964645492873469,-0.67463950922821,
-23.492031044981));
#22788=CARTESIAN_POINT('Ctrl Pts',(-1.04403294838599,-0.543538738702725,
-23.502302863744));
#22789=CARTESIAN_POINT('Ctrl Pts',(-1.14741281624633,-0.255940576564088,
-23.5231468506275));
#22790=CARTESIAN_POINT('Ctrl Pts',(-1.1712680167499,-0.103495740972837,
-23.5334627805691));
#22791=CARTESIAN_POINT('Ctrl Pts',(-1.1599290802664,0.200711799883823,-23.5542375650592));
#22792=CARTESIAN_POINT('Ctrl Pts',(-1.12443400769239,0.347254015711778,
-23.5643397811048));
#22793=CARTESIAN_POINT('Ctrl Pts',(-0.996337557365363,0.623448679756951,
-23.5850966850865));
#22794=CARTESIAN_POINT('Ctrl Pts',(-0.907612571565183,0.747550899402566,
-23.5953023673021));
#22795=CARTESIAN_POINT('Ctrl Pts',(-0.670667541538861,0.971611561905498,
-23.617566642625));
#22796=CARTESIAN_POINT('Ctrl Pts',(-0.534098101668266,1.04481672619882,
-23.6279248529788));
#22797=CARTESIAN_POINT('Ctrl Pts',(-0.275000467066175,1.14249906388745,
-23.6467982047513));
#22798=CARTESIAN_POINT('Ctrl Pts',(-0.126580400966591,1.16904169170034,
-23.6568916601278));
#22799=CARTESIAN_POINT('Ctrl Pts',(0.20144190519578,1.163835599232,-23.6792958601877));
#22800=CARTESIAN_POINT('Ctrl Pts',(0.35191700207576,1.11877843828859,-23.6897825979081));
#22801=CARTESIAN_POINT('Ctrl Pts',(0.600644110469965,1.00987437100721,-23.7082867322753));
#22802=CARTESIAN_POINT('Ctrl Pts',(0.724118275574684,0.926513224982849,
-23.7182677916966));
#22803=CARTESIAN_POINT('Ctrl Pts',(0.953014052479287,0.696953711387198,
-23.7404107238412));
#22804=CARTESIAN_POINT('Ctrl Pts',(1.03140981474657,0.558593805864354,-23.7510273049906));
#22805=CARTESIAN_POINT('Ctrl Pts',(1.13438453848494,0.306051305202018,-23.7696126930082));
#22806=CARTESIAN_POINT('Ctrl Pts',(1.16487691003558,0.161569378790797,-23.779512573544));
#22807=CARTESIAN_POINT('Ctrl Pts',(1.1690082842922,-0.139132863968416,-23.8000550606958));
#22808=CARTESIAN_POINT('Ctrl Pts',(1.13860814951507,-0.294856378754733,
-23.8106622296586));
#22809=CARTESIAN_POINT('Ctrl Pts',(1.03508416460198,-0.550324677970256,
-23.8294473277748));
#22810=CARTESIAN_POINT('Ctrl Pts',(0.962396519410018,-0.68289928505056,
-23.8395560462992));
#22811=CARTESIAN_POINT('Ctrl Pts',(0.734653378267124,-0.919414535474106,
-23.8619812077135));
#22812=CARTESIAN_POINT('Ctrl Pts',(0.604162830263392,-1.00897060908126,
-23.8725580530661));
#22813=CARTESIAN_POINT('Ctrl Pts',(0.345574805573191,-1.12114628543803,
-23.8917705495728));
#22814=CARTESIAN_POINT('Ctrl Pts',(0.199711254916898,-1.16297986281931,
-23.9019230808372));
#22815=CARTESIAN_POINT('Ctrl Pts',(-0.126933676780373,-1.16957945210744,
-23.9242292828711));
#22816=CARTESIAN_POINT('Ctrl Pts',(-0.281876844625177,-1.1416255416875,
-23.9347495650282));
#22817=CARTESIAN_POINT('Ctrl Pts',(-0.570992366278221,-1.02925644591801,
-23.9558983763229));
#22818=CARTESIAN_POINT('Ctrl Pts',(-0.697263581724959,-0.948022205646459,
-23.9659604824616));
#22819=CARTESIAN_POINT('Ctrl Pts',(-0.916131644797461,-0.737369452220616,
-23.9866904752755));
#22820=CARTESIAN_POINT('Ctrl Pts',(-1.00561323080168,-0.609375357425688,
-23.99712681397));
#22821=CARTESIAN_POINT('Ctrl Pts',(-1.13039245242821,-0.328317197026739,
-24.0181021416964));
#22822=CARTESIAN_POINT('Ctrl Pts',(-1.1634069179183,-0.178818109672421,
-24.0283633413595));
#22823=CARTESIAN_POINT('Ctrl Pts',(-1.16875032198559,0.12696882202449,-24.0492232952251));
#22824=CARTESIAN_POINT('Ctrl Pts',(-1.14219860207787,0.279159893052852,
-24.0595514605357));
#22825=CARTESIAN_POINT('Ctrl Pts',(-1.03394101835653,0.562304922521268,
-24.0802380394371));
#22826=CARTESIAN_POINT('Ctrl Pts',(-0.95368391938154,0.689879242768186,
-24.0903371103175));
#22827=CARTESIAN_POINT('Ctrl Pts',(-0.742383306622126,0.911216853453345,
-24.1112005351712));
#22828=CARTESIAN_POINT('Ctrl Pts',(-0.618206000916698,1.00020464731638,
-24.1214196096764));
#22829=CARTESIAN_POINT('Ctrl Pts',(-0.321789924774097,1.13584465913637,
-24.1436737563466));
#22830=CARTESIAN_POINT('Ctrl Pts',(-0.169162204071789,1.16122379076491,
-24.1540179844192));
#22831=CARTESIAN_POINT('Ctrl Pts',(0.108153891961831,1.17016174517532,-24.1729300210824));
#22832=CARTESIAN_POINT('Ctrl Pts',(0.257408061948685,1.14734985937776,-24.1830368577589));
#22833=CARTESIAN_POINT('Ctrl Pts',(0.565904932159938,1.03666604024609,-24.2054191523544));
#22834=CARTESIAN_POINT('Ctrl Pts',(0.693688938373763,0.945769370032585,
-24.2158902244772));
#22835=CARTESIAN_POINT('Ctrl Pts',(0.894475531414044,0.76194677441218,-24.2344423045361));
#22836=CARTESIAN_POINT('Ctrl Pts',(0.984535131627163,0.643003781679394,
-24.2444366233424));
#22837=CARTESIAN_POINT('Ctrl Pts',(1.13391927855465,0.337728284171994,-24.2676508056257));
#22838=CARTESIAN_POINT('Ctrl Pts',(1.1576563306076,0.176511653662717,-24.2784973022939));
#22839=CARTESIAN_POINT('Ctrl Pts',(1.17242604546444,-0.0765243655160787,
-24.2957700105566));
#22840=CARTESIAN_POINT('Ctrl Pts',(1.15463119368819,-0.222860809232089,
-24.3056531858431));
#22841=CARTESIAN_POINT('Ctrl Pts',(1.0651105549098,-0.498377005437864,-24.3254418679969));
#22842=CARTESIAN_POINT('Ctrl Pts',(0.993492488919996,-0.627225226741351,
-24.3353250432864));
#22843=CARTESIAN_POINT('Ctrl Pts',(0.83281269822665,-0.823254245872666,
-24.3525977515491));
#22844=CARTESIAN_POINT('Ctrl Pts',(0.718848261881902,-0.939728950600801,
-24.3634442482174));
#22845=CARTESIAN_POINT('Ctrl Pts',(0.418557513006822,-1.09889621756008,
-24.3866584305006));
#22846=CARTESIAN_POINT('Ctrl Pts',(0.275784828936188,-1.14218741521005,
-24.3966527493069));
#22847=CARTESIAN_POINT('Ctrl Pts',(0.00529685218042203,-1.17288362077003,
-24.4152048293658));
#22848=CARTESIAN_POINT('Ctrl Pts',(-0.15151030268991,-1.17131101737357,
-24.4256759014886));
#22849=CARTESIAN_POINT('Ctrl Pts',(-0.466147829955441,-1.07952619736496,
-24.4480581960842));
#22850=CARTESIAN_POINT('Ctrl Pts',(-0.60030548000498,-1.01025200068753,
-24.4581650327607));
#22851=CARTESIAN_POINT('Ctrl Pts',(-0.819405316722027,-0.840018732202679,
-24.477077069424));
#22852=CARTESIAN_POINT('Ctrl Pts',(-0.927966257295848,-0.7297742600928,
-24.4874212974965));
#22853=CARTESIAN_POINT('Ctrl Pts',(-1.08804470173287,-0.445810187314043,
-24.5096754441668));
#22854=CARTESIAN_POINT('Ctrl Pts',(-1.13620053949762,-0.300827960823797,
-24.519894518672));
#22855=CARTESIAN_POINT('Ctrl Pts',(-1.1770473428035,0.00243731169511532,
-24.5407579435258));
#22856=CARTESIAN_POINT('Ctrl Pts',(-1.16699039578116,0.152821043989816,
-24.5508570144063));
#22857=CARTESIAN_POINT('Ctrl Pts',(-1.08814414820036,0.445522395862589,
-24.5715435933077));
#22858=CARTESIAN_POINT('Ctrl Pts',(-1.02016927375459,0.584254268101373,
-24.5818717586182));
#22859=CARTESIAN_POINT('Ctrl Pts',(-0.836109320261249,0.82850031839418,
-24.6027317124839));
#22860=CARTESIAN_POINT('Ctrl Pts',(-0.721526697841524,0.93004220478004,
-24.612992912147));
#22861=CARTESIAN_POINT('Ctrl Pts',(-0.455376345281851,1.08407964668604,
-24.6339682398733));
#22862=CARTESIAN_POINT('Ctrl Pts',(-0.307751180219848,1.1350330879498,-24.6444045785678));
#22863=CARTESIAN_POINT('Ctrl Pts',(-0.00686461584986442,1.17680732571145,
-24.6651345713816));
#22864=CARTESIAN_POINT('Ctrl Pts',(0.143039231759796,1.16830684838774,-24.6751966775203));
#22865=CARTESIAN_POINT('Ctrl Pts',(0.44298749942166,1.08927751667136,-24.6963454888151));
#22866=CARTESIAN_POINT('Ctrl Pts',(0.584770051659173,1.0208193962577,-24.7068657709722));
#22867=CARTESIAN_POINT('Ctrl Pts',(0.84515221127406,0.823483142780032,-24.7291719730062));
#22868=CARTESIAN_POINT('Ctrl Pts',(0.938569142779572,0.703902623820296,
-24.7393245042705));
#22869=CARTESIAN_POINT('Ctrl Pts',(1.08183604106747,0.461156367959811,-24.7585370007774));
#22870=CARTESIAN_POINT('Ctrl Pts',(1.13476537268836,0.312003562781931,-24.76911384613));
#22871=CARTESIAN_POINT('Ctrl Pts',(1.17999326808417,-0.0132053539141161,
-24.7915390075444));
#22872=CARTESIAN_POINT('Ctrl Pts',(1.16087340945535,-0.163185189932334,
-24.8016477260688));
#22873=CARTESIAN_POINT('Ctrl Pts',(1.09446557386838,-0.430713257112194,
-24.820432824185));
#22874=CARTESIAN_POINT('Ctrl Pts',(1.02752781410787,-0.574564977887768,
-24.8310399931477));
#22875=CARTESIAN_POINT('Ctrl Pts',(0.847437118499067,-0.81540984166698,
-24.8515824802994));
#22876=CARTESIAN_POINT('Ctrl Pts',(0.737843926148438,-0.914375209208886,
-24.8614823608351));
#22877=CARTESIAN_POINT('Ctrl Pts',(0.506094867186335,-1.05815936007466,
-24.8800677488527));
#22878=CARTESIAN_POINT('Ctrl Pts',(0.3613454512501,-1.12401500207983,-24.890684330002));
#22879=CARTESIAN_POINT('Ctrl Pts',(0.0412331811787559,-1.17519098782271,
-24.9128272621465));
#22880=CARTESIAN_POINT('Ctrl Pts',(-0.107657969004568,-1.17005527833936,
-24.9228083215679));
#22881=CARTESIAN_POINT('Ctrl Pts',(-0.372894631319867,-1.11196239336716,
-24.9413124559351));
#22882=CARTESIAN_POINT('Ctrl Pts',(-0.521115476638633,-1.0599673595054,
-24.9517991936555));
#22883=CARTESIAN_POINT('Ctrl Pts',(-0.789551161232938,-0.871372502801514,
-24.9742033937154));
#22884=CARTESIAN_POINT('Ctrl Pts',(-0.894024151828224,-0.762659939827971,
-24.9842968490918));
#22885=CARTESIAN_POINT('Ctrl Pts',(-1.04622230392104,-0.531339500064551,
-25.0031702008643));
#22886=CARTESIAN_POINT('Ctrl Pts',(-1.11368038572552,-0.391841775405243,
-25.0135284112181));
#22887=CARTESIAN_POINT('Ctrl Pts',(-1.17367338871164,-0.0713000974154914,
-25.0357926865411));
#22888=CARTESIAN_POINT('Ctrl Pts',(-1.17250795556528,0.0812519454809356,
-25.0459983687568));
#22889=CARTESIAN_POINT('Ctrl Pts',(-1.11379701051142,0.379991326821873,
-25.0667552727385));
#22890=CARTESIAN_POINT('Ctrl Pts',(-1.05637777413877,0.519409950007744,
-25.0768574887841));
#22891=CARTESIAN_POINT('Ctrl Pts',(-0.886742460300511,0.772183880019224,
-25.0976322732742));
#22892=CARTESIAN_POINT('Ctrl Pts',(-0.777838371540452,0.881492607670503,
-25.1079482032157));
#22893=CARTESIAN_POINT('Ctrl Pts',(-0.525156343273892,1.05339924667952,
-25.1287921900992));
#22894=CARTESIAN_POINT('Ctrl Pts',(-0.383871443144744,1.11279922244327,
-25.1390640088622));
#22895=CARTESIAN_POINT('Ctrl Pts',(-0.0822383474976608,1.17290119324133,
-25.1600428339846));
#22896=CARTESIAN_POINT('Ctrl Pts',(0.0738049670078697,1.17358654470157,
-25.1704702882553));
#22897=CARTESIAN_POINT('Ctrl Pts',(0.30694278066829,1.12890832363893,-25.1866704170972));
#22898=CARTESIAN_POINT('Ctrl Pts',(0.388002311516126,1.10401248060505,-25.1924302352649));
#22899=CARTESIAN_POINT('Ctrl Pts',(0.543589114829183,1.03581167186204,-25.2040367304977));
#22900=CARTESIAN_POINT('Ctrl Pts',(0.617180537264655,0.993262033258738,
-25.2098054059139));
#22901=CARTESIAN_POINT('Ctrl Pts',(0.685452796065063,0.943448854418561,
-25.2155687196295));
#22902=CARTESIAN_POINT('Ctrl Pts',(1.1723987758447E-10,-1.16616519645621,
-23.3000561192829));
#22903=CARTESIAN_POINT('Ctrl Pts',(-0.0845143073622228,-1.16633564847594,
-23.3058195310012));
#22904=CARTESIAN_POINT('Ctrl Pts',(-0.169062527012607,-1.15750294251081,
-23.3115883046236));
#22905=CARTESIAN_POINT('Ctrl Pts',(-0.33502302258755,-1.12122647584571,
-23.3231948531434));
#22906=CARTESIAN_POINT('Ctrl Pts',(-0.415234336721324,-1.09372217755542,
-23.3289546280455));
#22907=CARTESIAN_POINT('Ctrl Pts',(-0.630107390685439,-0.992832930186849,
-23.3451547117448));
#22908=CARTESIAN_POINT('Ctrl Pts',(-0.755946244497973,-0.900558510223433,
-23.3555821660154));
#22909=CARTESIAN_POINT('Ctrl Pts',(-0.964645492873463,-0.674639509228219,
-23.3765609911377));
#22910=CARTESIAN_POINT('Ctrl Pts',(-1.04403294838599,-0.543538738702735,
-23.3868328099007));
#22911=CARTESIAN_POINT('Ctrl Pts',(-1.14741281624633,-0.2559405765641,-23.4076767967842));
#22912=CARTESIAN_POINT('Ctrl Pts',(-1.1712680167499,-0.103495740972848,
-23.4179927267258));
#22913=CARTESIAN_POINT('Ctrl Pts',(-1.1599290802664,0.200711799883798,-23.4387675112159));
#22914=CARTESIAN_POINT('Ctrl Pts',(-1.1244340076924,0.347254015711756,-23.4488697272615));
#22915=CARTESIAN_POINT('Ctrl Pts',(-0.996337557365367,0.623448679756947,
-23.4696266312432));
#22916=CARTESIAN_POINT('Ctrl Pts',(-0.907612571565185,0.747550899402563,
-23.4798323134588));
#22917=CARTESIAN_POINT('Ctrl Pts',(-0.670667541538861,0.971611561905498,
-23.5020965887818));
#22918=CARTESIAN_POINT('Ctrl Pts',(-0.534098101668265,1.04481672619882,
-23.5124547991357));
#22919=CARTESIAN_POINT('Ctrl Pts',(-0.275000467066174,1.14249906388745,
-23.5313281509082));
#22920=CARTESIAN_POINT('Ctrl Pts',(-0.12658040096659,1.16904169170034,-23.5414216062847));
#22921=CARTESIAN_POINT('Ctrl Pts',(0.201441905195779,1.163835599232,-23.5638258063446));
#22922=CARTESIAN_POINT('Ctrl Pts',(0.351917002075758,1.11877843828859,-23.5743125440649));
#22923=CARTESIAN_POINT('Ctrl Pts',(0.600644110469963,1.00987437100721,-23.5928166784321));
#22924=CARTESIAN_POINT('Ctrl Pts',(0.72411827557468,0.926513224982852,-23.6027977378534));
#22925=CARTESIAN_POINT('Ctrl Pts',(0.953014052479293,0.696953711387194,
-23.6249406699979));
#22926=CARTESIAN_POINT('Ctrl Pts',(1.03140981474657,0.558593805864345,-23.6355572511473));
#22927=CARTESIAN_POINT('Ctrl Pts',(1.13438453848494,0.306051305202025,-23.6541426391649));
#22928=CARTESIAN_POINT('Ctrl Pts',(1.16487691003558,0.161569378790804,-23.6640425197007));
#22929=CARTESIAN_POINT('Ctrl Pts',(1.1690082842922,-0.139132863968409,-23.6845850068526));
#22930=CARTESIAN_POINT('Ctrl Pts',(1.13860814951507,-0.294856378754726,
-23.6951921758154));
#22931=CARTESIAN_POINT('Ctrl Pts',(1.03508416460199,-0.550324677970245,
-23.7139772739316));
#22932=CARTESIAN_POINT('Ctrl Pts',(0.962396519410025,-0.682899285050549,
-23.724085992456));
#22933=CARTESIAN_POINT('Ctrl Pts',(0.734653378267133,-0.919414535474099,
-23.7465111538702));
#22934=CARTESIAN_POINT('Ctrl Pts',(0.604162830263402,-1.00897060908125,
-23.7570879992228));
#22935=CARTESIAN_POINT('Ctrl Pts',(0.3455748055732,-1.12114628543803,-23.7763004957295));
#22936=CARTESIAN_POINT('Ctrl Pts',(0.199711254916905,-1.16297986281931,
-23.7864530269939));
#22937=CARTESIAN_POINT('Ctrl Pts',(-0.126933676780369,-1.16957945210744,
-23.8087592290278));
#22938=CARTESIAN_POINT('Ctrl Pts',(-0.281876844625174,-1.14162554168751,
-23.819279511185));
#22939=CARTESIAN_POINT('Ctrl Pts',(-0.570992366278222,-1.02925644591801,
-23.8404283224798));
#22940=CARTESIAN_POINT('Ctrl Pts',(-0.697263581724958,-0.948022205646458,
-23.8504904286185));
#22941=CARTESIAN_POINT('Ctrl Pts',(-0.916131644797455,-0.737369452220623,
-23.8712204214323));
#22942=CARTESIAN_POINT('Ctrl Pts',(-1.00561323080168,-0.609375357425699,
-23.8816567601267));
#22943=CARTESIAN_POINT('Ctrl Pts',(-1.13039245242821,-0.328317197026754,
-23.902632087853));
#22944=CARTESIAN_POINT('Ctrl Pts',(-1.1634069179183,-0.17881810967244,-23.9128932875161));
#22945=CARTESIAN_POINT('Ctrl Pts',(-1.16875032198559,0.126968822024469,
-23.9337532413817));
#22946=CARTESIAN_POINT('Ctrl Pts',(-1.14219860207787,0.279159893052831,
-23.9440814066923));
#22947=CARTESIAN_POINT('Ctrl Pts',(-1.03394101835655,0.562304922521242,
-23.9647679855936));
#22948=CARTESIAN_POINT('Ctrl Pts',(-0.953683919381558,0.689879242768163,
-23.9748670564741));
#22949=CARTESIAN_POINT('Ctrl Pts',(-0.742383306622142,0.911216853453332,
-23.9957304813278));
#22950=CARTESIAN_POINT('Ctrl Pts',(-0.618206000916717,1.00020464731637,
-24.005949555833));
#22951=CARTESIAN_POINT('Ctrl Pts',(-0.321789924774117,1.13584465913636,
-24.0282037025032));
#22952=CARTESIAN_POINT('Ctrl Pts',(-0.169162204071811,1.16122379076491,
-24.0385479305758));
#22953=CARTESIAN_POINT('Ctrl Pts',(0.108153891961813,1.17016174517532,-24.057459967239));
#22954=CARTESIAN_POINT('Ctrl Pts',(0.25740806194867,1.14734985937777,-24.0675668039155));
#22955=CARTESIAN_POINT('Ctrl Pts',(0.565904932159931,1.03666604024609,-24.089949098511));
#22956=CARTESIAN_POINT('Ctrl Pts',(0.69368893837376,0.945769370032588,-24.1004201706339));
#22957=CARTESIAN_POINT('Ctrl Pts',(0.894475531414044,0.76194677441218,-24.118972250693));
#22958=CARTESIAN_POINT('Ctrl Pts',(0.984535131627164,0.643003781679392,
-24.1289665694994));
#22959=CARTESIAN_POINT('Ctrl Pts',(1.13391927855465,0.337728284171982,-24.1521807517827));
#22960=CARTESIAN_POINT('Ctrl Pts',(1.15765633060761,0.176511653662702,-24.163027248451));
#22961=CARTESIAN_POINT('Ctrl Pts',(1.17242604546444,-0.0765243655160832,
-24.1802999567137));
#22962=CARTESIAN_POINT('Ctrl Pts',(1.15463119368819,-0.222860809232091,
-24.1901831320031));
#22963=CARTESIAN_POINT('Ctrl Pts',(1.0651105549098,-0.498377005437862,-24.2099718141569));
#22964=CARTESIAN_POINT('Ctrl Pts',(0.993492488919999,-0.627225226741345,
-24.2198549894433));
#22965=CARTESIAN_POINT('Ctrl Pts',(0.832812698226625,-0.823254245872699,
-24.237127697706));
#22966=CARTESIAN_POINT('Ctrl Pts',(0.71884826188187,-0.939728950600817,
-24.2479741943742));
#22967=CARTESIAN_POINT('Ctrl Pts',(0.418557513006823,-1.09889621756008,
-24.2711883766575));
#22968=CARTESIAN_POINT('Ctrl Pts',(0.275784828936185,-1.14218741521005,
-24.2811826954639));
#22969=CARTESIAN_POINT('Ctrl Pts',(0.00529685218041781,-1.17288362077003,
-24.2997347755229));
#22970=CARTESIAN_POINT('Ctrl Pts',(-0.151510302689914,-1.17131101737357,
-24.3102058476458));
#22971=CARTESIAN_POINT('Ctrl Pts',(-0.466147829955446,-1.07952619736495,
-24.3325881422413));
#22972=CARTESIAN_POINT('Ctrl Pts',(-0.600305480004984,-1.01025200068752,
-24.3426949789178));
#22973=CARTESIAN_POINT('Ctrl Pts',(-0.819405316722026,-0.840018732202679,
-24.361607015581));
#22974=CARTESIAN_POINT('Ctrl Pts',(-0.927966257295847,-0.729774260092801,
-24.3719512436536));
#22975=CARTESIAN_POINT('Ctrl Pts',(-1.08804470173286,-0.445810187314049,
-24.3942053903238));
#22976=CARTESIAN_POINT('Ctrl Pts',(-1.13620053949761,-0.300827960823807,
-24.4044244648289));
#22977=CARTESIAN_POINT('Ctrl Pts',(-1.1770473428035,0.00243731169510533,
-24.4252878896826));
#22978=CARTESIAN_POINT('Ctrl Pts',(-1.16699039578116,0.152821043989804,
-24.435386960563));
#22979=CARTESIAN_POINT('Ctrl Pts',(-1.08814414820037,0.445522395862568,
-24.4560735394643));
#22980=CARTESIAN_POINT('Ctrl Pts',(-1.0201692737546,0.58425426810135,-24.4664017047749));
#22981=CARTESIAN_POINT('Ctrl Pts',(-0.836109320261269,0.828500318394159,
-24.4872616586406));
#22982=CARTESIAN_POINT('Ctrl Pts',(-0.721526697841547,0.930042204780023,
-24.4975228583036));
#22983=CARTESIAN_POINT('Ctrl Pts',(-0.455376345281878,1.08407964668603,
-24.51849818603));
#22984=CARTESIAN_POINT('Ctrl Pts',(-0.30775118021988,1.13503308794979,-24.5289345247244));
#22985=CARTESIAN_POINT('Ctrl Pts',(-0.00686461584989813,1.17680732571145,
-24.5496645175382));
#22986=CARTESIAN_POINT('Ctrl Pts',(0.143039231759763,1.16830684838775,-24.5597266236769));
#22987=CARTESIAN_POINT('Ctrl Pts',(0.442987499421629,1.08927751667137,-24.5808754349717));
#22988=CARTESIAN_POINT('Ctrl Pts',(0.584770051659144,1.02081939625772,-24.5913957171289));
#22989=CARTESIAN_POINT('Ctrl Pts',(0.845152211274036,0.823483142780056,
-24.6137019191628));
#22990=CARTESIAN_POINT('Ctrl Pts',(0.938569142779552,0.703902623820324,
-24.6238544504271));
#22991=CARTESIAN_POINT('Ctrl Pts',(1.08183604106745,0.461156367959846,-24.6430669469338));
#22992=CARTESIAN_POINT('Ctrl Pts',(1.13476537268834,0.312003562781974,-24.6536437922862));
#22993=CARTESIAN_POINT('Ctrl Pts',(1.17999326808417,-0.0132053539140601,
-24.6760689537004));
#22994=CARTESIAN_POINT('Ctrl Pts',(1.16087340945535,-0.163185189932275,
-24.6861776722248));
#22995=CARTESIAN_POINT('Ctrl Pts',(1.0944655738684,-0.430713257112141,-24.704962770341));
#22996=CARTESIAN_POINT('Ctrl Pts',(1.0275278141079,-0.57456497788772,-24.7155699393038));
#22997=CARTESIAN_POINT('Ctrl Pts',(0.847437118499099,-0.815409841666948,
-24.7361124264557));
#22998=CARTESIAN_POINT('Ctrl Pts',(0.737843926148467,-0.914375209208864,
-24.7460123069917));
#22999=CARTESIAN_POINT('Ctrl Pts',(0.506094867186354,-1.05815936007465,
-24.7645976950094));
#23000=CARTESIAN_POINT('Ctrl Pts',(0.361345451250116,-1.12401500207983,
-24.7752142761589));
#23001=CARTESIAN_POINT('Ctrl Pts',(0.041233181178773,-1.17519098782271,
-24.7973572083035));
#23002=CARTESIAN_POINT('Ctrl Pts',(-0.10765796900455,-1.17005527833937,
-24.8073382677247));
#23003=CARTESIAN_POINT('Ctrl Pts',(-0.372894631319849,-1.11196239336716,
-24.8258424020919));
#23004=CARTESIAN_POINT('Ctrl Pts',(-0.521115476638615,-1.05996735950541,
-24.8363291398122));
#23005=CARTESIAN_POINT('Ctrl Pts',(-0.789551161232922,-0.871372502801528,
-24.8587333398721));
#23006=CARTESIAN_POINT('Ctrl Pts',(-0.894024151828209,-0.762659939827989,
-24.8688267952486));
#23007=CARTESIAN_POINT('Ctrl Pts',(-1.04622230392103,-0.531339500064575,
-24.8877001470211));
#23008=CARTESIAN_POINT('Ctrl Pts',(-1.11368038572551,-0.391841775405268,
-24.8980583573751));
#23009=CARTESIAN_POINT('Ctrl Pts',(-1.17367338871164,-0.0713000974155191,
-24.920322632698));
#23010=CARTESIAN_POINT('Ctrl Pts',(-1.17250795556528,0.0812519454809048,
-24.9305283149136));
#23011=CARTESIAN_POINT('Ctrl Pts',(-1.11379701051143,0.37999132682184,-24.9512852188952));
#23012=CARTESIAN_POINT('Ctrl Pts',(-1.05637777413879,0.519409950007713,
-24.9613874349407));
#23013=CARTESIAN_POINT('Ctrl Pts',(-0.886742460300535,0.772183880019197,
-24.9821622194308));
#23014=CARTESIAN_POINT('Ctrl Pts',(-0.777838371540479,0.881492607670479,
-24.9924781493724));
#23015=CARTESIAN_POINT('Ctrl Pts',(-0.525156343273925,1.0533992466795,-25.0133221362559));
#23016=CARTESIAN_POINT('Ctrl Pts',(-0.383871443144776,1.11279922244326,
-25.023593955019));
#23017=CARTESIAN_POINT('Ctrl Pts',(-0.0822383474976909,1.17290119324133,
-25.0445727801414));
#23018=CARTESIAN_POINT('Ctrl Pts',(0.0738049670078393,1.17358654470157,
-25.055000234412));
#23019=CARTESIAN_POINT('Ctrl Pts',(0.306942780668673,1.12890832363886,-25.071200363254));
#23020=CARTESIAN_POINT('Ctrl Pts',(0.388002311516887,1.10401248060482,-25.0769601814217));
#23021=CARTESIAN_POINT('Ctrl Pts',(0.543589168675984,1.03581164825843,-25.0885666806713));
#23022=CARTESIAN_POINT('Ctrl Pts',(0.617180639658102,0.993261974056082,
-25.0943353600971));
#23023=CARTESIAN_POINT('Ctrl Pts',(0.685452938553338,0.943448750455471,
-25.1000986778145));
#23024=CARTESIAN_POINT('Origin',(0.,-1.5,-23.2));
#23025=CARTESIAN_POINT('',(0.,-1.5,-23.2));
#23026=CARTESIAN_POINT('',(-8.54668270915563E-15,-1.33934539329655,-23.2));
#23027=CARTESIAN_POINT('',(0.,-1.5,-23.2));
#23028=CARTESIAN_POINT('',(-1.17966937551839E-5,-1.49965598532183,-23.6078060837911));
#23029=CARTESIAN_POINT('',(0.,-1.5,-23.2));
#23030=CARTESIAN_POINT('Ctrl Pts',(4.62482517256554E-17,-1.16616519702491,
-23.4155261734628));
#23031=CARTESIAN_POINT('Ctrl Pts',(5.33250787523106E-15,-1.22186610458458,
-23.4477077782494));
#23032=CARTESIAN_POINT('Ctrl Pts',(4.91669986271183E-12,-1.277567012145,
-23.4798893830346));
#23033=CARTESIAN_POINT('Ctrl Pts',(4.91669986271183E-12,-1.38870769975953,
-23.5441017242884));
#23034=CARTESIAN_POINT('Ctrl Pts',(2.86542950228376E-14,-1.44414747981368,
-23.5761324607567));
#23035=CARTESIAN_POINT('Ctrl Pts',(-2.3555004955933E-17,-1.49958725986734,
-23.6081631972259));
#23036=CARTESIAN_POINT('Ctrl Pts',(-1.84338803809923E-15,-1.33934539329655,
-23.2));
#23037=CARTESIAN_POINT('Ctrl Pts',(-7.75535507767301E-14,-1.31070585588327,
-23.2165467012055));
#23038=CARTESIAN_POINT('Ctrl Pts',(-2.65179795051112E-12,-1.28206631847006,
-23.2330934024111));
#23039=CARTESIAN_POINT('Ctrl Pts',(-2.65179795051112E-12,-1.22433958636177,
-23.2664454420754));
#23040=CARTESIAN_POINT('Ctrl Pts',(-6.50204480007271E-15,-1.1952523916667,
-23.283250780534));
#23041=CARTESIAN_POINT('Ctrl Pts',(1.17253245002305E-16,-1.16616519697187,
-23.3000561189931));
#23042=CARTESIAN_POINT('Origin',(0.,0.,-23.2));
#23043=CARTESIAN_POINT('',(-1.37415215024357,-0.600878825228823,-23.1998750239129));
#23044=CARTESIAN_POINT('Ctrl Pts',(-1.37395140486162,-0.600796654813404,
-23.2));
#23045=CARTESIAN_POINT('Ctrl Pts',(-1.30510436453987,-0.726707931106893,
-23.2));
#23046=CARTESIAN_POINT('Ctrl Pts',(-1.21950806160512,-0.839865179830455,
-23.2));
#23047=CARTESIAN_POINT('Ctrl Pts',(-1.01762571865116,-1.03693888018822,
-23.2));
#23048=CARTESIAN_POINT('Ctrl Pts',(-0.904301269126984,-1.11974701485562,
-23.2));
#23049=CARTESIAN_POINT('Ctrl Pts',(-0.660860104715333,-1.24907445588305,
-23.2));
#23050=CARTESIAN_POINT('Ctrl Pts',(-0.530821098017273,-1.29615412710268,
-23.2));
#23051=CARTESIAN_POINT('Ctrl Pts',(-0.265883748469263,-1.3477441557919,
-23.2));
#23052=CARTESIAN_POINT('Ctrl Pts',(-0.131789325248617,-1.35315533998259,
-23.2));
#23053=CARTESIAN_POINT('Ctrl Pts',(-8.70831184940357E-15,-1.33934539329655,
-23.2));
#23054=CARTESIAN_POINT('',(-1.37630824614812,-0.596469288048168,-23.2));
#23055=CARTESIAN_POINT('Ctrl Pts',(-1.37435083629484,-0.600965705157694,
-23.1998750239129));
#23056=CARTESIAN_POINT('Ctrl Pts',(-1.37500575571379,-0.599467967360972,
-23.1999166826086));
#23057=CARTESIAN_POINT('Ctrl Pts',(-1.37565822682721,-0.597969158987785,
-23.1999583413043));
#23058=CARTESIAN_POINT('Ctrl Pts',(-1.37630824614812,-0.596469288048168,
-23.2));
#23059=CARTESIAN_POINT('Origin',(0.,0.,-23.2));
#23060=CARTESIAN_POINT('Ctrl Pts',(0.6710062646147,-1.380656119664,-23.05156091023));
#23061=CARTESIAN_POINT('Ctrl Pts',(0.3326844530463,-1.545082331076,-23.07106091023));
#23062=CARTESIAN_POINT('Ctrl Pts',(-0.4683422360403,-1.612847596885,-23.11006091023));
#23063=CARTESIAN_POINT('Ctrl Pts',(-1.42946546972,-0.8821571614021,-23.16856091023));
#23064=CARTESIAN_POINT('Ctrl Pts',(-1.651847110892,0.3043759554816,-23.22706091023));
#23065=CARTESIAN_POINT('Ctrl Pts',(-1.021129492522,1.333641902982,-23.28556091023));
#23066=CARTESIAN_POINT('Ctrl Pts',(0.1370469690624,1.674073791154,-23.34406091023));
#23067=CARTESIAN_POINT('Ctrl Pts',(1.224428737161,1.149815288114,-23.40256091023));
#23068=CARTESIAN_POINT('Ctrl Pts',(1.679374972687,0.03165926908636,-23.46106091023));
#23069=CARTESIAN_POINT('Ctrl Pts',(1.266895850185,-1.102849551308,-23.51956091023));
#23070=CARTESIAN_POINT('Ctrl Pts',(0.2000443226221,-1.667718359793,-23.57806091023));
#23071=CARTESIAN_POINT('Ctrl Pts',(-0.9701334287918,-1.371183213173,-23.63656091023));
#23072=CARTESIAN_POINT('Ctrl Pts',(-1.639221290546,-0.3664093696299,-23.69506091023));
#23073=CARTESIAN_POINT('Ctrl Pts',(-1.461624385972,0.8276209410372,-23.75356091023));
#23074=CARTESIAN_POINT('Ctrl Pts',(-0.52907443495,1.594171417921,-23.81206091023));
#23075=CARTESIAN_POINT('Ctrl Pts',(0.6767511671866,1.53730612602,-23.87056091023));
#23076=CARTESIAN_POINT('Ctrl Pts',(1.533023655909,0.686396924418,-23.92906091023));
#23077=CARTESIAN_POINT('Ctrl Pts',(1.597464201167,-0.519047582986,-23.98756091023));
#23078=CARTESIAN_POINT('Ctrl Pts',(0.8367882010172,-1.456395473099,-24.04606091023));
#23079=CARTESIAN_POINT('Ctrl Pts',(-0.3561026739166,-1.641491137051,-24.10456091023));
#23080=CARTESIAN_POINT('Ctrl Pts',(-1.365060658244,-0.9787296188165,-24.16306091023));
#23081=CARTESIAN_POINT('Ctrl Pts',(-1.668942351274,0.1895618522656,-24.22156091023));
#23082=CARTESIAN_POINT('Ctrl Pts',(-1.110787857823,1.259941506756,-24.28006091023));
#23083=CARTESIAN_POINT('Ctrl Pts',(0.02110684019029,1.679540644058,-24.33856091023));
#23084=CARTESIAN_POINT('Ctrl Pts',(1.142099513493,1.231629392261,-24.39706091023));
#23085=CARTESIAN_POINT('Ctrl Pts',(1.673178974659,0.1475613323174,-24.45556091023));
#23086=CARTESIAN_POINT('Ctrl Pts',(1.340034041364,-1.012724728735,-24.51406091023));
#23087=CARTESIAN_POINT('Ctrl Pts',(0.3147391875509,-1.649921262663,-24.57256091023));
#23088=CARTESIAN_POINT('Ctrl Pts',(-0.8731225586908,-1.434908334168,-24.63106091023));
#23089=CARTESIAN_POINT('Ctrl Pts',(-1.610006155319,-0.4787341075376,-24.68956091023));
#23090=CARTESIAN_POINT('Ctrl Pts',(-1.515280082606,0.7246860501608,-24.74806091023));
#23091=CARTESIAN_POINT('Ctrl Pts',(-0.6379428881994,1.553898857047,-24.80656091023));
#23092=CARTESIAN_POINT('Ctrl Pts',(0.569111203504,1.580105774587,-24.86506091023));
#23093=CARTESIAN_POINT('Ctrl Pts',(1.177323984063,1.054450848381,-24.90406091023));
#23094=CARTESIAN_POINT('Ctrl Pts',(1.354384777031,0.7225666776598,-24.92356091023));
#23095=CARTESIAN_POINT('Ctrl Pts',(0.6122628206918,-1.259786167148,-23.12915029444));
#23096=CARTESIAN_POINT('Ctrl Pts',(0.303559493203,-1.409817636753,-23.14865029444));
#23097=CARTESIAN_POINT('Ctrl Pts',(-0.4273410750521,-1.471650372119,-23.18765029444));
#23098=CARTESIAN_POINT('Ctrl Pts',(-1.304322488069,-0.804928449131,-23.24615029444));
#23099=CARTESIAN_POINT('Ctrl Pts',(-1.507235662021,0.2777292715157,-23.30465029444));
#23100=CARTESIAN_POINT('Ctrl Pts',(-0.9317344059998,1.216887824112,-23.36315029444));
#23101=CARTESIAN_POINT('Ctrl Pts',(0.1250491512082,1.527516500918,-23.42165029444));
#23102=CARTESIAN_POINT('Ctrl Pts',(1.117235757524,1.049154365167,-23.48015029444));
#23103=CARTESIAN_POINT('Ctrl Pts',(1.53235358893,0.02888764891485,-23.53865029444));
#23104=CARTESIAN_POINT('Ctrl Pts',(1.15598507445,-1.006300257822,-23.59715029444));
#23105=CARTESIAN_POINT('Ctrl Pts',(0.1825313826277,-1.521717457694,-23.65565029444));
#23106=CARTESIAN_POINT('Ctrl Pts',(-0.8852028079061,-1.251142569086,-23.71415029444));
#23107=CARTESIAN_POINT('Ctrl Pts',(-1.495715172889,-0.3343319518877,-23.77265029444));
#23108=CARTESIAN_POINT('Ctrl Pts',(-1.333666042389,0.7551666184726,-23.83115029444));
#23109=CARTESIAN_POINT('Ctrl Pts',(-0.4827564554623,1.454609204823,-23.88965029444));
#23110=CARTESIAN_POINT('Ctrl Pts',(0.6175047840515,1.402722201892,-23.94815029444));
#23111=CARTESIAN_POINT('Ctrl Pts',(1.398814641906,0.6263061005841,-24.00665029444));
#23112=CARTESIAN_POINT('Ctrl Pts',(1.457613720376,-0.4736074072494,-24.06515029444));
#23113=CARTESIAN_POINT('Ctrl Pts',(0.7635313279386,-1.328894896257,-24.12365029444));
#23114=CARTESIAN_POINT('Ctrl Pts',(-0.3249275589301,-1.497786305004,-24.18215029444));
#23115=CARTESIAN_POINT('Ctrl Pts',(-1.245556015057,-0.8930464419066,-24.24065029444));
#23116=CARTESIAN_POINT('Ctrl Pts',(-1.522834294475,0.1729666032706,-24.29915029444));
#23117=CARTESIAN_POINT('Ctrl Pts',(-1.013543602922,1.149639551094,-24.35765029444));
#23118=CARTESIAN_POINT('Ctrl Pts',(0.01925903555941,1.532504756551,-24.41615029444));
#23119=CARTESIAN_POINT('Ctrl Pts',(1.042114070341,1.123806029122,-24.47465029444));
#23120=CARTESIAN_POINT('Ctrl Pts',(1.5267000214,0.1346430313905,-24.53315029444));
#23121=CARTESIAN_POINT('Ctrl Pts',(1.22272036083,-0.9240654397699,-24.59165029444));
#23122=CARTESIAN_POINT('Ctrl Pts',(0.2871852513371,-1.50547841275,-24.65015029444));
#23123=CARTESIAN_POINT('Ctrl Pts',(-0.7966847834135,-1.309288855323,-24.70865029444));
#23124=CARTESIAN_POINT('Ctrl Pts',(-1.469057685405,-0.4368231870542,-24.76715029444));
#23125=CARTESIAN_POINT('Ctrl Pts',(-1.38262443503,0.6612431933735,-24.82565029444));
#23126=CARTESIAN_POINT('Ctrl Pts',(-0.5820939874436,1.417862317323,-24.88415029444));
#23127=CARTESIAN_POINT('Ctrl Pts',(0.5192881931508,1.441774942437,-24.94265029444));
#23128=CARTESIAN_POINT('Ctrl Pts',(1.07425480411,0.9621386338044,-24.98165029444));
#23129=CARTESIAN_POINT('Ctrl Pts',(1.235814757055,0.6593093619714,-25.00115029444));
#23130=CARTESIAN_POINT('Ctrl Pts',(0.5535193767689,-1.138916214631,-23.20673967864));
#23131=CARTESIAN_POINT('Ctrl Pts',(0.2744345333596,-1.27455294243,-23.22623967864));
#23132=CARTESIAN_POINT('Ctrl Pts',(-0.3863399140639,-1.330453147354,-23.26523967864));
#23133=CARTESIAN_POINT('Ctrl Pts',(-1.179179506419,-0.72769973686,-23.32373967864));
#23134=CARTESIAN_POINT('Ctrl Pts',(-1.362624213149,0.2510825875499,-23.38223967864));
#23135=CARTESIAN_POINT('Ctrl Pts',(-0.8423393194779,1.100133745242,-23.44073967864));
#23136=CARTESIAN_POINT('Ctrl Pts',(0.1130513333539,1.380959210682,-23.49923967864));
#23137=CARTESIAN_POINT('Ctrl Pts',(1.010042777888,0.9484934422207,-23.55773967864));
#23138=CARTESIAN_POINT('Ctrl Pts',(1.385332205172,0.02611602874334,-23.61623967864));
#23139=CARTESIAN_POINT('Ctrl Pts',(1.045074298715,-0.9097509643373,-23.67473967864));
#23140=CARTESIAN_POINT('Ctrl Pts',(0.1650184426333,-1.375716555595,-23.73323967864));
#23141=CARTESIAN_POINT('Ctrl Pts',(-0.8002721870203,-1.131101924998,-23.79173967864));
#23142=CARTESIAN_POINT('Ctrl Pts',(-1.352209055232,-0.3022545341455,-23.85023967864));
#23143=CARTESIAN_POINT('Ctrl Pts',(-1.205707698806,0.682712295908,-23.90873967864));
#23144=CARTESIAN_POINT('Ctrl Pts',(-0.4364384759746,1.315046991726,-23.96723967864));
#23145=CARTESIAN_POINT('Ctrl Pts',(0.5582584009165,1.268138277765,-24.02573967864));
#23146=CARTESIAN_POINT('Ctrl Pts',(1.264605627904,0.5662152767502,-24.08423967864));
#23147=CARTESIAN_POINT('Ctrl Pts',(1.317763239585,-0.4281672315128,-24.14273967864));
#23148=CARTESIAN_POINT('Ctrl Pts',(0.6902744548601,-1.201394319414,-24.20123967864));
#23149=CARTESIAN_POINT('Ctrl Pts',(-0.2937524439436,-1.354081472956,-24.25973967864));
#23150=CARTESIAN_POINT('Ctrl Pts',(-1.12605137187,-0.8073632649967,-24.31823967864));
#23151=CARTESIAN_POINT('Ctrl Pts',(-1.376726237677,0.1563713542756,-24.37673967864));
#23152=CARTESIAN_POINT('Ctrl Pts',(-0.9162993480212,1.039337595432,-24.43523967864));
#23153=CARTESIAN_POINT('Ctrl Pts',(0.01741123092852,1.385468869044,-24.49373967864));
#23154=CARTESIAN_POINT('Ctrl Pts',(0.9421286271891,1.015982665983,-24.55223967864));
#23155=CARTESIAN_POINT('Ctrl Pts',(1.380221068141,0.1217247304635,-24.61073967864));
#23156=CARTESIAN_POINT('Ctrl Pts',(1.105406680295,-0.8354061508049,-24.66923967864));
#23157=CARTESIAN_POINT('Ctrl Pts',(0.2596313151233,-1.361035562837,-24.72773967864));
#23158=CARTESIAN_POINT('Ctrl Pts',(-0.7202470081362,-1.183669376478,-24.78623967864));
#23159=CARTESIAN_POINT('Ctrl Pts',(-1.32810921549,-0.3949122665708,-24.84473967864));
#23160=CARTESIAN_POINT('Ctrl Pts',(-1.249968787454,0.5978003365862,-24.90323967864));
#23161=CARTESIAN_POINT('Ctrl Pts',(-0.5262450866879,1.2818257776,-24.96173967864));
#23162=CARTESIAN_POINT('Ctrl Pts',(0.4694651827977,1.303444110288,-25.02023967864));
#23163=CARTESIAN_POINT('Ctrl Pts',(0.9711856241576,0.8698264192279,-25.05923967864));
#23164=CARTESIAN_POINT('Ctrl Pts',(1.117244737079,0.5960520462829,-25.07873967864));
#23165=CARTESIAN_POINT('Ctrl Pts',(0.494775932846,-1.018046262115,-23.28432906285));
#23166=CARTESIAN_POINT('Ctrl Pts',(0.2453095735162,-1.139288248107,-23.30382906285));
#23167=CARTESIAN_POINT('Ctrl Pts',(-0.3453387530757,-1.189255922589,-23.34282906285));
#23168=CARTESIAN_POINT('Ctrl Pts',(-1.054036524768,-0.6504710245889,-23.40132906285));
#23169=CARTESIAN_POINT('Ctrl Pts',(-1.218012764277,0.224435903584,-23.45982906285));
#23170=CARTESIAN_POINT('Ctrl Pts',(-0.752944232956,0.9833796663719,-23.51832906285));
#23171=CARTESIAN_POINT('Ctrl Pts',(0.1010535154996,1.234401920446,-23.57682906285));
#23172=CARTESIAN_POINT('Ctrl Pts',(0.9028497982508,0.8478325192742,-23.63532906285));
#23173=CARTESIAN_POINT('Ctrl Pts',(1.238310821415,0.02334440857184,-23.69382906285));
#23174=CARTESIAN_POINT('Ctrl Pts',(0.9341635229797,-0.8132016708522,-23.75232906285));
#23175=CARTESIAN_POINT('Ctrl Pts',(0.147505502639,-1.229715653496,-23.81082906285));
#23176=CARTESIAN_POINT('Ctrl Pts',(-0.7153415661346,-1.011061280911,-23.86932906285));
#23177=CARTESIAN_POINT('Ctrl Pts',(-1.208702937575,-0.2701771164033,-23.92782906285));
#23178=CARTESIAN_POINT('Ctrl Pts',(-1.077749355224,0.6102579733435,-23.98632906285));
#23179=CARTESIAN_POINT('Ctrl Pts',(-0.390120496487,1.175484778628,-24.04482906285));
#23180=CARTESIAN_POINT('Ctrl Pts',(0.4990120177814,1.133554353637,-24.10332906285));
#23181=CARTESIAN_POINT('Ctrl Pts',(1.130396613902,0.5061244529163,-24.16182906285));
#23182=CARTESIAN_POINT('Ctrl Pts',(1.177912758794,-0.3827270557762,-24.22032906285));
#23183=CARTESIAN_POINT('Ctrl Pts',(0.6170175817815,-1.073893742571,-24.27882906285));
#23184=CARTESIAN_POINT('Ctrl Pts',(-0.2625773289571,-1.210376640909,-24.33732906285));
#23185=CARTESIAN_POINT('Ctrl Pts',(-1.006546728684,-0.7216800880868,-24.39582906285));
#23186=CARTESIAN_POINT('Ctrl Pts',(-1.230618180878,0.1397761052806,-24.45432906285));
#23187=CARTESIAN_POINT('Ctrl Pts',(-0.8190550931204,0.9290356397707,-24.51282906285));
#23188=CARTESIAN_POINT('Ctrl Pts',(0.01556342629763,1.238432981537,-24.57132906285));
#23189=CARTESIAN_POINT('Ctrl Pts',(0.8421431840371,0.9081593028442,-24.62982906285));
#23190=CARTESIAN_POINT('Ctrl Pts',(1.233742114882,0.1088064295365,-24.68832906285));
#23191=CARTESIAN_POINT('Ctrl Pts',(0.9880929997609,-0.74674686184,-24.74682906285));
#23192=CARTESIAN_POINT('Ctrl Pts',(0.2320773789096,-1.216592712924,-24.80532906285));
#23193=CARTESIAN_POINT('Ctrl Pts',(-0.6438092328589,-1.058049897633,-24.86382906285));
#23194=CARTESIAN_POINT('Ctrl Pts',(-1.187160745576,-0.3530013460875,-24.92232906285));
#23195=CARTESIAN_POINT('Ctrl Pts',(-1.117313139878,0.5343574797989,-24.98082906285));
#23196=CARTESIAN_POINT('Ctrl Pts',(-0.4703961859322,1.145789237877,-25.03932906285));
#23197=CARTESIAN_POINT('Ctrl Pts',(0.4196421724445,1.165113278138,-25.09782906285));
#23198=CARTESIAN_POINT('Ctrl Pts',(0.868116444205,0.7775142046514,-25.13682906285));
#23199=CARTESIAN_POINT('Ctrl Pts',(0.9986747171026,0.5327947305945,-25.15632906285));
#23200=CARTESIAN_POINT('',(0.881417616740998,1.21316726808339,-24.9080680842712));
#23201=CARTESIAN_POINT('',(0.8816778784387,1.213525491562,-24.9078125));
#23202=CARTESIAN_POINT('Ctrl Pts',(0.881292186436105,1.2129552818722,-24.9076220436819));
#23203=CARTESIAN_POINT('Ctrl Pts',(0.813750271409058,1.26196190916497,-24.9033243807288));
#23204=CARTESIAN_POINT('Ctrl Pts',(0.742132286672347,1.30535258528533,-24.8990878485097));
#23205=CARTESIAN_POINT('Ctrl Pts',(0.608818775191422,1.37169837443908,-24.8914037622482));
#23206=CARTESIAN_POINT('Ctrl Pts',(0.548260654619934,1.39706761640043,-24.8879781469134));
#23207=CARTESIAN_POINT('Ctrl Pts',(0.39749304186689,1.44874200558769,-24.8794109477088));
#23208=CARTESIAN_POINT('Ctrl Pts',(0.305935590287384,1.47074921695453,-24.8741977037729));
#23209=CARTESIAN_POINT('Ctrl Pts',(0.15278657673726,1.4927545949536,-24.8656689066726));
#23210=CARTESIAN_POINT('Ctrl Pts',(0.0918784597345684,1.49775789527344,
-24.8623263527439));
#23211=CARTESIAN_POINT('Ctrl Pts',(-0.0886411888191926,1.50144175853413,
-24.852665407421));
#23212=CARTESIAN_POINT('Ctrl Pts',(-0.208315581115914,1.48940022238857,
-24.8466068804931));
#23213=CARTESIAN_POINT('Ctrl Pts',(-0.39236239919342,1.44861653779783,-24.8369761561396));
#23214=CARTESIAN_POINT('Ctrl Pts',(-0.458874442850795,1.4290120499256,-24.8334250708226));
#23215=CARTESIAN_POINT('Ctrl Pts',(-0.63199737795491,1.36460644461159,-24.8237016461764));
#23216=CARTESIAN_POINT('Ctrl Pts',(-0.735128019387501,1.31179606028223,
-24.8173189749409));
#23217=CARTESIAN_POINT('Ctrl Pts',(-0.882982165912429,1.21340966409492,
-24.8075323201994));
#23218=CARTESIAN_POINT('Ctrl Pts',(-0.933036895109152,1.17538518997163,
-24.8040917368683));
#23219=CARTESIAN_POINT('Ctrl Pts',(-1.06916735064738,1.05767099961853,-24.7944542492941));
#23220=CARTESIAN_POINT('Ctrl Pts',(-1.1485937720974,0.970569640255831,-24.7884997685678));
#23221=CARTESIAN_POINT('Ctrl Pts',(-1.25838806744895,0.818037383718444,
-24.7788910714682));
#23222=CARTESIAN_POINT('Ctrl Pts',(-1.2957921674127,0.757516126799102,-24.7752483055596));
#23223=CARTESIAN_POINT('Ctrl Pts',(-1.38323055549452,0.590505260775706,
-24.7653254281035));
#23224=CARTESIAN_POINT('Ctrl Pts',(-1.42510970387548,0.480319881150026,
-24.7588302302505));
#23225=CARTESIAN_POINT('Ctrl Pts',(-1.46898630328235,0.306611347798785,
-24.7489566081849));
#23226=CARTESIAN_POINT('Ctrl Pts',(-1.48049392039261,0.245226787825081,
-24.7455389360445));
#23227=CARTESIAN_POINT('Ctrl Pts',(-1.5024994387051,0.0663503691542141,
-24.7358897487153));
#23228=CARTESIAN_POINT('Ctrl Pts',(-1.50288937912599,-0.0522048494724794,
-24.7299055858667));
#23229=CARTESIAN_POINT('Ctrl Pts',(-1.4817105010691,-0.239134287010421,
-24.7202890613195));
#23230=CARTESIAN_POINT('Ctrl Pts',(-1.4688737986894,-0.308622107701723,
-24.7166706810548));
#23231=CARTESIAN_POINT('Ctrl Pts',(-1.42180898819625,-0.490309138131947,
-24.706791054986));
#23232=CARTESIAN_POINT('Ctrl Pts',(-1.37906692655925,-0.599786657877916,
-24.7003149527047));
#23233=CARTESIAN_POINT('Ctrl Pts',(-1.29526185013709,-0.757783930027831,
-24.6904587784379));
#23234=CARTESIAN_POINT('Ctrl Pts',(-1.26261342105573,-0.811057262292604,
-24.6870394931226));
#23235=CARTESIAN_POINT('Ctrl Pts',(-1.15900292604867,-0.958435669844394,
-24.677393871737));
#23236=CARTESIAN_POINT('Ctrl Pts',(-1.07985190574382,-1.04656613879994,
-24.6714141517122));
#23237=CARTESIAN_POINT('Ctrl Pts',(-0.938821515558382,-1.17101393298127,
-24.6617994293038));
#23238=CARTESIAN_POINT('Ctrl Pts',(-0.882652752376579,-1.21398931661285,
-24.658178068226));
#23239=CARTESIAN_POINT('Ctrl Pts',(-0.725847001858296,-1.31722777390087,
-24.6482956722769));
#23240=CARTESIAN_POINT('Ctrl Pts',(-0.62072554295621,-1.36976964615758,
-24.6418200195264));
#23241=CARTESIAN_POINT('Ctrl Pts',(-0.452588776858701,-1.43077115137843,
-24.631963162524));
#23242=CARTESIAN_POINT('Ctrl Pts',(-0.392626605356742,-1.44839704644404,
-24.6285429153169));
#23243=CARTESIAN_POINT('Ctrl Pts',(-0.216923859472755,-1.48823041094892,
-24.6188968450495));
#23244=CARTESIAN_POINT('Ctrl Pts',(-0.0991174670356461,-1.50051832964543,
-24.6129175660533));
#23245=CARTESIAN_POINT('Ctrl Pts',(0.0889566198733414,-1.49824840253018,
-24.6033027545031));
#23246=CARTESIAN_POINT('Ctrl Pts',(0.159453701695883,-1.49245512572619,
-24.5996808117517));
#23247=CARTESIAN_POINT('Ctrl Pts',(0.345044403354946,-1.46386267850922,
-24.589796258383));
#23248=CARTESIAN_POINT('Ctrl Pts',(0.458284854486528,-1.43232338869741,
-24.5833189041695));
#23249=CARTESIAN_POINT('Ctrl Pts',(0.623927363713742,-1.36479135546227,
-24.5734609757527));
#23250=CARTESIAN_POINT('Ctrl Pts',(0.68021580859676,-1.33765248581722,-24.57004128029));
#23251=CARTESIAN_POINT('Ctrl Pts',(0.837251949738321,-1.24935791899591,
-24.5603955359266));
#23252=CARTESIAN_POINT('Ctrl Pts',(0.932878002667334,-1.17945695385794,
-24.5544160740831));
#23253=CARTESIAN_POINT('Ctrl Pts',(1.07085431523807,-1.05163277204398,-24.5448013759728));
#23254=CARTESIAN_POINT('Ctrl Pts',(1.11925441241422,-1.00005817266383,-24.5411797608701));
#23255=CARTESIAN_POINT('Ctrl Pts',(1.23773373934732,-0.854379964570187,
-24.5312954975683));
#23256=CARTESIAN_POINT('Ctrl Pts',(1.30057562534765,-0.755035607038862,
-24.524818073943));
#23257=CARTESIAN_POINT('Ctrl Pts',(1.37814483295167,-0.593849848204767,
-24.5149601914699));
#23258=CARTESIAN_POINT('Ctrl Pts',(1.40169350712799,-0.535969264020991,
-24.511540594146));
#23259=CARTESIAN_POINT('Ctrl Pts',(1.45894404008101,-0.365186416635365,
-24.5018966389706));
#23260=CARTESIAN_POINT('Ctrl Pts',(1.48298857842733,-0.249234655671714,
-24.4959186763304));
#23261=CARTESIAN_POINT('Ctrl Pts',(1.49961006934388,-0.0619021396642318,
-24.4863049087931));
#23262=CARTESIAN_POINT('Ctrl Pts',(1.50092325670157,0.00882732721460973,
-24.4826826532579));
#23263=CARTESIAN_POINT('Ctrl Pts',(1.49110174781038,0.196414588786735,-24.4727948396999));
#23264=CARTESIAN_POINT('Ctrl Pts',(1.47107248443378,0.312304732375535,-24.4663142250903));
#23265=CARTESIAN_POINT('Ctrl Pts',(1.42047933685597,0.483918369138487,-24.4564543923671));
#23266=CARTESIAN_POINT('Ctrl Pts',(1.39912933998889,0.542625566360721,-24.4530358789866));
#23267=CARTESIAN_POINT('Ctrl Pts',(1.32710453912062,0.707560423036113,-24.443400022294));
#23268=CARTESIAN_POINT('Ctrl Pts',(1.26724730078268,0.809584908205953,-24.4374283054397));
#23269=CARTESIAN_POINT('Ctrl Pts',(1.15401414708386,0.959645746089114,-24.427818696445));
#23270=CARTESIAN_POINT('Ctrl Pts',(1.10752727641671,1.01303417658909,-24.4241940858983));
#23271=CARTESIAN_POINT('Ctrl Pts',(0.9742325963301,1.14581559669533,-24.4142908555267));
#23272=CARTESIAN_POINT('Ctrl Pts',(0.88143995646911,1.21848666838532,-24.407795873451));
#23273=CARTESIAN_POINT('Ctrl Pts',(0.728639877624673,1.31187350357391,-24.3979274052997));
#23274=CARTESIAN_POINT('Ctrl Pts',(0.67349734345046,1.34104294964111,-24.3945138908));
#23275=CARTESIAN_POINT('Ctrl Pts',(0.510072211568302,1.41475472021774,-24.3849160593254));
#23276=CARTESIAN_POINT('Ctrl Pts',(0.397850923756175,1.45014455786576,-24.3789737568079));
#23277=CARTESIAN_POINT('Ctrl Pts',(0.21361703934987,1.48561996992641,-24.3693836366579));
#23278=CARTESIAN_POINT('Ctrl Pts',(0.143103616043984,1.49412400232197,-24.3657478588718));
#23279=CARTESIAN_POINT('Ctrl Pts',(-0.0462245798991654,1.50338481745475,
-24.3557722684762));
#23280=CARTESIAN_POINT('Ctrl Pts',(-0.16497506476068,1.49489169683256,-24.3492099394591));
#23281=CARTESIAN_POINT('Ctrl Pts',(-0.341635297904301,1.46122051886648,
-24.339300929914));
#23282=CARTESIAN_POINT('Ctrl Pts',(-0.40168846752061,1.44588807069254,-24.3359106954327));
#23283=CARTESIAN_POINT('Ctrl Pts',(-0.569165069113878,1.39179256958006,
-24.326492277347));
#23284=CARTESIAN_POINT('Ctrl Pts',(-0.673574380521842,1.34419321597958,
-24.3206893223395));
#23285=CARTESIAN_POINT('Ctrl Pts',(-0.832983653401516,1.24859302731924,
-24.3111902997536));
#23286=CARTESIAN_POINT('Ctrl Pts',(-0.89205425273673,1.20717492033352,-24.3075009205939));
#23287=CARTESIAN_POINT('Ctrl Pts',(-1.04426960828044,1.08314089363536,-24.2971765530218));
#23288=CARTESIAN_POINT('Ctrl Pts',(-1.13034759047191,0.99276491454057,-24.2902882687428));
#23289=CARTESIAN_POINT('Ctrl Pts',(-1.23975512101156,0.845378328185136,
-24.2801829784649));
#23290=CARTESIAN_POINT('Ctrl Pts',(-1.27261687360187,0.795087916784433,
-24.2769030093859));
#23291=CARTESIAN_POINT('Ctrl Pts',(-1.35016124987809,0.659084689820279,
-24.2685413130271));
#23292=CARTESIAN_POINT('Ctrl Pts',(-1.38976628412931,0.570545163521608,
-24.2635940533201));
#23293=CARTESIAN_POINT('Ctrl Pts',(-1.45734660921659,0.370092757231955,
-24.2527865695785));
#23294=CARTESIAN_POINT('Ctrl Pts',(-1.48171110516211,0.256732925585599,
-24.2469103074676));
#23295=CARTESIAN_POINT('Ctrl Pts',(-1.49878345438743,0.0772267943211951,
-24.2372239416081));
#23296=CARTESIAN_POINT('Ctrl Pts',(-1.50069825172818,0.0122604498412598,
-24.2336574519884));
#23297=CARTESIAN_POINT('Ctrl Pts',(-1.49442141966965,-0.166418379349362,
-24.2237960813223));
#23298=CARTESIAN_POINT('Ctrl Pts',(-1.47747513477829,-0.280015777404685,
-24.2174920903743));
#23299=CARTESIAN_POINT('Ctrl Pts',(-1.42862829365822,-0.460529189075349,
-24.2076773817912));
#23300=CARTESIAN_POINT('Ctrl Pts',(-1.40465643945064,-0.528987438284961,
-24.203972765019));
#23301=CARTESIAN_POINT('Ctrl Pts',(-1.32987150064611,-0.701764400345165,
-24.1943537829878));
#23302=CARTESIAN_POINT('Ctrl Pts',(-1.27151458210261,-0.803020441266229,
-24.1884335009969));
#23303=CARTESIAN_POINT('Ctrl Pts',(-1.16311715722858,-0.948414882803426,
-24.1786901896031));
#23304=CARTESIAN_POINT('Ctrl Pts',(-1.12085812636559,-0.99796742210812,
-24.1751161589507));
#23305=CARTESIAN_POINT('Ctrl Pts',(-0.996464372208961,-1.12603876221773,
-24.1652683401806));
#23306=CARTESIAN_POINT('Ctrl Pts',(-0.907991374518774,-1.19866787009211,
-24.158986199618));
#23307=CARTESIAN_POINT('Ctrl Pts',(-0.751094390359184,-1.29958205710181,
-24.1491949064351));
#23308=CARTESIAN_POINT('Ctrl Pts',(-0.687472040199729,-1.33426379509695,
-24.1454937678829));
#23309=CARTESIAN_POINT('Ctrl Pts',(-0.516034566704189,-1.41236834930936,
-24.1358683944185));
#23310=CARTESIAN_POINT('Ctrl Pts',(-0.404651865476461,-1.44841095506151,
-24.1299385363247));
#23311=CARTESIAN_POINT('Ctrl Pts',(-0.226510571785679,-1.48358649221646,
-24.1201828209351));
#23312=CARTESIAN_POINT('Ctrl Pts',(-0.161901953900477,-1.49199639775794,
-24.1166071409542));
#23313=CARTESIAN_POINT('Ctrl Pts',(0.016208666646669,-1.50353686146712,
-24.1067622797767));
#23314=CARTESIAN_POINT('Ctrl Pts',(0.130459101926883,-1.4980701290517,-24.100484909495));
#23315=CARTESIAN_POINT('Ctrl Pts',(0.314420568759343,-1.46771724748399,
-24.0906987270847));
#23316=CARTESIAN_POINT('Ctrl Pts',(0.384857966348204,-1.45077906986724,
-24.0869983458818));
#23317=CARTESIAN_POINT('Ctrl Pts',(0.564433582448083,-1.39373616655142,
-24.0773715740196));
#23318=CARTESIAN_POINT('Ctrl Pts',(0.671265280341864,-1.34575275193793,
-24.071439624749));
#23319=CARTESIAN_POINT('Ctrl Pts',(0.827032804048919,-1.25233919616798,
-24.0616811953725));
#23320=CARTESIAN_POINT('Ctrl Pts',(0.88060050168267,-1.21524032396105,-24.058105150167));
#23321=CARTESIAN_POINT('Ctrl Pts',(1.02044021136514,-1.10434754659587,-24.0482609298713));
#23322=CARTESIAN_POINT('Ctrl Pts',(1.10150410730434,-1.02367874592046,-24.0419846020692));
#23323=CARTESIAN_POINT('Ctrl Pts',(1.21758661059533,-0.877802170786594,
-24.0321995178782));
#23324=CARTESIAN_POINT('Ctrl Pts',(1.25847168705654,-0.818000102121312,
-24.0284992847203));
#23325=CARTESIAN_POINT('Ctrl Pts',(1.35341775156855,-0.655246657205866,
-24.0188722160153));
#23326=CARTESIAN_POINT('Ctrl Pts',(1.40048172163325,-0.547996899633102,
-24.0129398344978));
#23327=CARTESIAN_POINT('Ctrl Pts',(1.45337233543707,-0.374226951070174,
-24.0031808300433));
#23328=CARTESIAN_POINT('Ctrl Pts',(1.46822410367749,-0.310780476710637,
-23.9996046939037));
#23329=CARTESIAN_POINT('Ctrl Pts',(1.49757300893425,-0.134742336175255,
-23.9897607141101));
#23330=CARTESIAN_POINT('Ctrl Pts',(1.50359769498047,-0.0205445865747881,
-23.9834847242317));
#23331=CARTESIAN_POINT('Ctrl Pts',(1.49186521076666,0.1655038259662,-23.9737001202437));
#23332=CARTESIAN_POINT('Ctrl Pts',(1.48208405018167,0.237279392863777,-23.9700000507006));
#23333=CARTESIAN_POINT('Ctrl Pts',(1.443354829439,0.421682017743482,-23.9603728791471));
#23334=CARTESIAN_POINT('Ctrl Pts',(1.40633221427024,0.53280431410137,-23.9544402446658));
#23335=CARTESIAN_POINT('Ctrl Pts',(1.3290170891885,0.697172897033738,-23.9446810631271));
#23336=CARTESIAN_POINT('Ctrl Pts',(1.2974818058085,0.754192951728386,-23.9411050426264));
#23337=CARTESIAN_POINT('Ctrl Pts',(1.20118138229273,0.904458840363217,-23.9312606180205));
#23338=CARTESIAN_POINT('Ctrl Pts',(1.12905258297626,0.993212264983639,-23.9249840655136));
#23339=CARTESIAN_POINT('Ctrl Pts',(0.99555468038911,1.12335461280545,-23.9151984677531));
#23340=CARTESIAN_POINT('Ctrl Pts',(0.94015286025791,1.1700379249029,-23.9114979455082));
#23341=CARTESIAN_POINT('Ctrl Pts',(0.787747907437857,1.28083574158385,-23.9018708469453));
#23342=CARTESIAN_POINT('Ctrl Pts',(0.685767216586177,1.33842155135958,-23.8959387021292));
#23343=CARTESIAN_POINT('Ctrl Pts',(0.518179799229006,1.40848436018197,-23.8861795305405));
#23344=CARTESIAN_POINT('Ctrl Pts',(0.456536185774643,1.42963027762125,-23.8826029416154));
#23345=CARTESIAN_POINT('Ctrl Pts',(0.284344918213945,1.47649031407643,-23.8727597710839));
#23346=CARTESIAN_POINT('Ctrl Pts',(0.171350805511131,1.49394174300891,-23.8664850805791));
#23347=CARTESIAN_POINT('Ctrl Pts',(-0.0149067568169257,1.50094304571182,
-23.8567019973112));
#23348=CARTESIAN_POINT('Ctrl Pts',(-0.0872953159708956,1.49841681252354,
-23.8530022513087));
#23349=CARTESIAN_POINT('Ctrl Pts',(-0.274653153292379,1.47839610883237,
-23.8433751700276));
#23350=CARTESIAN_POINT('Ctrl Pts',(-0.388935673680077,1.4527147936456,-23.8374423246153));
#23351=CARTESIAN_POINT('Ctrl Pts',(-0.560227605017933,1.39229294224809,
-23.8276836033757));
#23352=CARTESIAN_POINT('Ctrl Pts',(-0.620113874544232,1.36664666328502,
-23.8241082892213));
#23353=CARTESIAN_POINT('Ctrl Pts',(-0.779273560583134,1.28592927114846,
-23.814264837881));
#23354=CARTESIAN_POINT('Ctrl Pts',(-0.874816906047994,1.22308003203388,
-23.8079884291192));
#23355=CARTESIAN_POINT('Ctrl Pts',(-1.01765919442854,1.10336579439268,-23.7982060714263));
#23356=CARTESIAN_POINT('Ctrl Pts',(-1.06963151729626,1.05297467866217,-23.7945084502914));
#23357=CARTESIAN_POINT('Ctrl Pts',(-1.19521011167544,0.912456583884857,
-23.7848800324962));
#23358=CARTESIAN_POINT('Ctrl Pts',(-1.26279982894885,0.81670182455948,-23.7789439151475));
#23359=CARTESIAN_POINT('Ctrl Pts',(-1.34935216351238,0.656945061118655,
-23.7691821278869));
#23360=CARTESIAN_POINT('Ctrl Pts',(-1.37656451834724,0.597768821033822,
-23.7656076108186));
#23361=CARTESIAN_POINT('Ctrl Pts',(-1.44058442680957,0.430883963769553,
-23.7557483227243));
#23362=CARTESIAN_POINT('Ctrl Pts',(-1.46934288907299,0.319885892868802,
-23.7494556404723));
#23363=CARTESIAN_POINT('Ctrl Pts',(-1.49499671235264,0.134531929525419,
-23.7396342765976));
#23364=CARTESIAN_POINT('Ctrl Pts',(-1.49970494926013,0.0618465296069818,
-23.7359139852706));
#23365=CARTESIAN_POINT('Ctrl Pts',(-1.49833434475102,-0.12642650271697,
-23.7262924158087));
#23366=CARTESIAN_POINT('Ctrl Pts',(-1.48422494267998,-0.242142611424862,
-23.720383982627));
#23367=CARTESIAN_POINT('Ctrl Pts',(-1.44128641455023,-0.418464996353218,
-23.7106322664842));
#23368=CARTESIAN_POINT('Ctrl Pts',(-1.42162126502408,-0.480979297208294,
-23.7070351775453));
#23369=CARTESIAN_POINT('Ctrl Pts',(-1.35759602968765,-0.646103273059249,
-23.6972677758374));
#23370=CARTESIAN_POINT('Ctrl Pts',(-1.30553330549334,-0.745938503150817,
-23.6910898598436));
#23371=CARTESIAN_POINT('Ctrl Pts',(-1.20289977957849,-0.897698210470899,
-23.6814734943211));
#23372=CARTESIAN_POINT('Ctrl Pts',(-1.15906515562584,-0.953520068604759,
-23.6778476851766));
#23373=CARTESIAN_POINT('Ctrl Pts',(-1.03225726041117,-1.09356592048758,
-23.6682017104795));
#23374=CARTESIAN_POINT('Ctrl Pts',(-0.942582500787517,-1.17197371523185,
-23.6621823589794));
#23375=CARTESIAN_POINT('Ctrl Pts',(-0.792172583544227,-1.27455337196535,
-23.6524064769686));
#23376=CARTESIAN_POINT('Ctrl Pts',(-0.737419037677256,-1.30697126142047,
-23.6489159470707));
#23377=CARTESIAN_POINT('Ctrl Pts',(-0.596280754156468,-1.37890722070677,
-23.640173961861));
#23378=CARTESIAN_POINT('Ctrl Pts',(-0.507594195380326,-1.41402878226614,
-23.6349050185627));
#23379=CARTESIAN_POINT('Ctrl Pts',(-0.316036897635311,-1.46937081547821,
-23.6242553807404));
#23380=CARTESIAN_POINT('Ctrl Pts',(-0.212669147446816,-1.48775200308733,
-23.6189163456654));
#23381=CARTESIAN_POINT('Ctrl Pts',(-0.0724009869030183,-1.49795898083252,
-23.6117213803296));
#23382=CARTESIAN_POINT('Ctrl Pts',(-0.0362014860425619,-1.49928841111174,
-23.6098685598738));
#23383=CARTESIAN_POINT('Ctrl Pts',(-1.44394147025245E-6,-1.4993119708072,
-23.6080042218746));
#23384=CARTESIAN_POINT('Ctrl Pts',(-2.21494460401153E-5,-1.49999999983647,
-23.6076079457077));
#23385=CARTESIAN_POINT('Ctrl Pts',(0.0610512616330307,-1.50000090166462,
-23.6044870183155));
#23386=CARTESIAN_POINT('Ctrl Pts',(0.122065160139671,-1.49627182965613,
-23.6013464945155));
#23387=CARTESIAN_POINT('Ctrl Pts',(0.255962644401841,-1.4798427421027,-23.5941670216917));
#23388=CARTESIAN_POINT('Ctrl Pts',(0.328479811699856,-1.46545266079536,
-23.590095995072));
#23389=CARTESIAN_POINT('Ctrl Pts',(0.483909921285898,-1.42248916477728,
-23.5811996134758));
#23390=CARTESIAN_POINT('Ctrl Pts',(0.565987731379545,-1.3918705780163,-23.5763953841136));
#23391=CARTESIAN_POINT('Ctrl Pts',(0.778985033664735,-1.29043694267683,
-23.5637480203523));
#23392=CARTESIAN_POINT('Ctrl Pts',(0.902815515892788,-1.20705073239231,
-23.5562615648057));
#23393=CARTESIAN_POINT('Ctrl Pts',(1.0491205572373,-1.07323120591599,-23.5461215215063));
#23394=CARTESIAN_POINT('Ctrl Pts',(1.08416347801703,-1.03781900299683,-23.5435591375015));
#23395=CARTESIAN_POINT('Ctrl Pts',(1.17589390811468,-0.935396301720369,
-23.536304716054));
#23396=CARTESIAN_POINT('Ctrl Pts',(1.22855978406094,-0.865060983721391,
-23.5314596871629));
#23397=CARTESIAN_POINT('Ctrl Pts',(1.32009699721817,-0.7174533077395,-23.5218784328483));
#23398=CARTESIAN_POINT('Ctrl Pts',(1.35905270075097,-0.640603367541495,
-23.5171640521621));
#23399=CARTESIAN_POINT('Ctrl Pts',(1.43746671825191,-0.446089540182238,
-23.5059457278048));
#23400=CARTESIAN_POINT('Ctrl Pts',(1.46935172592144,-0.326059318947462,
-23.4996324550146));
#23401=CARTESIAN_POINT('Ctrl Pts',(1.49428732622014,-0.143933261681204,
-23.4902635412337));
#23402=CARTESIAN_POINT('Ctrl Pts',(1.49885342576748,-0.0839599013022765,
-23.4872013986174));
#23403=CARTESIAN_POINT('Ctrl Pts',(1.50081555415856,0.0392886786925357,
-23.4807580546551));
#23404=CARTESIAN_POINT('Ctrl Pts',(1.49782969294123,0.102446272228486,-23.4773443297187));
#23405=CARTESIAN_POINT('Ctrl Pts',(1.4799645131146,0.263653130021101,-23.4684439696149));
#23406=CARTESIAN_POINT('Ctrl Pts',(1.45933379792741,0.3607690875887,-23.4629454401956));
#23407=CARTESIAN_POINT('Ctrl Pts',(1.40014971170343,0.546624578076728,-23.4523907855226));
#23408=CARTESIAN_POINT('Ctrl Pts',(1.3623010153063,0.635103174225821,-23.447349924324));
#23409=CARTESIAN_POINT('Ctrl Pts',(1.27231522371821,0.799754549063724,-23.4376952019255));
#23410=CARTESIAN_POINT('Ctrl Pts',(1.22110731836698,0.875950726096881,-23.4330887732277));
#23411=CARTESIAN_POINT('Ctrl Pts',(1.12501199052552,0.99399205870297,-23.4252319952568));
#23412=CARTESIAN_POINT('Ctrl Pts',(1.08394732001753,1.03861910145001,-23.4220350972597));
#23413=CARTESIAN_POINT('Ctrl Pts',(0.972808301740653,1.1456086397659,-23.4136572393688));
#23414=CARTESIAN_POINT('Ctrl Pts',(0.899384500212469,1.20411084509114,-23.4084404180098));
#23415=CARTESIAN_POINT('Ctrl Pts',(0.744344138092426,1.30550278825905,-23.3983035776558));
#23416=CARTESIAN_POINT('Ctrl Pts',(0.663271081098984,1.34850270185102,-23.3934013753622));
#23417=CARTESIAN_POINT('Ctrl Pts',(0.495787299847338,1.41855102515141,-23.3839263068296));
#23418=CARTESIAN_POINT('Ctrl Pts',(0.409843129215484,1.44572517188591,-23.3793665661827));
#23419=CARTESIAN_POINT('Ctrl Pts',(0.244796967294499,1.48199849690076,-23.3707448905942));
#23420=CARTESIAN_POINT('Ctrl Pts',(0.16640320555457,1.49283445240194,-23.3666912231762));
#23421=CARTESIAN_POINT('Ctrl Pts',(0.0337154774817,1.50058903644668,-23.359547166957));
#23422=CARTESIAN_POINT('Ctrl Pts',(-0.0202118811268179,1.50083152916805,
-23.356586196228));
#23423=CARTESIAN_POINT('Ctrl Pts',(-0.141338295927296,1.49484599034754,
-23.3498998826809));
#23424=CARTESIAN_POINT('Ctrl Pts',(-0.208344787705541,1.48698821739586,
-23.346178279403));
#23425=CARTESIAN_POINT('Ctrl Pts',(-0.368108567587156,1.4572384051594,-23.3373357410272));
#23426=CARTESIAN_POINT('Ctrl Pts',(-0.459757384516831,1.43096938147552,
-23.3322987413637));
#23427=CARTESIAN_POINT('Ctrl Pts',(-0.64532285006907,1.35809505391628,-23.3219848572406));
#23428=CARTESIAN_POINT('Ctrl Pts',(-0.738101034400311,1.30998850421461,
-23.3167599218195));
#23429=CARTESIAN_POINT('Ctrl Pts',(-0.875729358686173,1.21933088560281,
-23.3082536226009));
#23430=CARTESIAN_POINT('Ctrl Pts',(-0.924246277437874,1.18297835351376,
-23.3050582831458));
#23431=CARTESIAN_POINT('Ctrl Pts',(-1.02443016465529,1.09797867852197,-23.2979235383796));
#23432=CARTESIAN_POINT('Ctrl Pts',(-1.07511362030052,1.04840106642832,-23.2939982324414));
#23433=CARTESIAN_POINT('Ctrl Pts',(-1.19166537252994,0.917017377479984,
-23.2843259939895));
#23434=CARTESIAN_POINT('Ctrl Pts',(-1.25282046894653,0.831523616904168,
-23.2786523187085));
#23435=CARTESIAN_POINT('Ctrl Pts',(-1.34688514110225,0.665772338535599,
-23.2686518583943));
#23436=CARTESIAN_POINT('Ctrl Pts',(-1.38273478368918,0.587705535401598,
-23.2642794417706));
#23437=CARTESIAN_POINT('Ctrl Pts',(-1.44209863967229,0.422409896427763,
-23.255329574732));
#23438=CARTESIAN_POINT('Ctrl Pts',(-1.46481145689039,0.335268966929233,
-23.2507632454323));
#23439=CARTESIAN_POINT('Ctrl Pts',(-1.48800856425733,0.196095877764329,
-23.2432034960859));
#23440=CARTESIAN_POINT('Ctrl Pts',(-1.49383577848236,0.145180448122853,
-23.2403976575781));
#23441=CARTESIAN_POINT('Ctrl Pts',(-1.50469129040932,-0.0275780324609217,
-23.2308668633208));
#23442=CARTESIAN_POINT('Ctrl Pts',(-1.49747999659813,-0.149715711461895,
-23.2241534790374));
#23443=CARTESIAN_POINT('Ctrl Pts',(-1.45503235568658,-0.382007620591668,
-23.2116320695379));
#23444=CARTESIAN_POINT('Ctrl Pts',(-1.42173049413197,-0.491660849941786,
-23.2058275953147));
#23445=CARTESIAN_POINT('Ctrl Pts',(-1.37630824614812,-0.596469288048168,
-23.2));
#23446=CARTESIAN_POINT('Origin',(0.,0.,-32.2));
#23447=CARTESIAN_POINT('Ctrl Pts',(0.494775932846,-1.018046262115,-23.35929593715));
#23448=CARTESIAN_POINT('Ctrl Pts',(0.2453095735162,-1.139288248107,-23.37879593715));
#23449=CARTESIAN_POINT('Ctrl Pts',(-0.3453387530757,-1.189255922589,-23.41779593715));
#23450=CARTESIAN_POINT('Ctrl Pts',(-1.054036524768,-0.6504710245889,-23.47629593715));
#23451=CARTESIAN_POINT('Ctrl Pts',(-1.218012764277,0.224435903584,-23.53479593715));
#23452=CARTESIAN_POINT('Ctrl Pts',(-0.752944232956,0.9833796663719,-23.59329593715));
#23453=CARTESIAN_POINT('Ctrl Pts',(0.1010535154996,1.234401920446,-23.65179593715));
#23454=CARTESIAN_POINT('Ctrl Pts',(0.9028497982508,0.8478325192742,-23.71029593715));
#23455=CARTESIAN_POINT('Ctrl Pts',(1.238310821415,0.02334440857184,-23.76879593715));
#23456=CARTESIAN_POINT('Ctrl Pts',(0.9341635229797,-0.8132016708522,-23.82729593715));
#23457=CARTESIAN_POINT('Ctrl Pts',(0.147505502639,-1.229715653496,-23.88579593715));
#23458=CARTESIAN_POINT('Ctrl Pts',(-0.7153415661346,-1.011061280911,-23.94429593715));
#23459=CARTESIAN_POINT('Ctrl Pts',(-1.208702937575,-0.2701771164033,-24.00279593715));
#23460=CARTESIAN_POINT('Ctrl Pts',(-1.077749355224,0.6102579733435,-24.06129593715));
#23461=CARTESIAN_POINT('Ctrl Pts',(-0.390120496487,1.175484778628,-24.11979593715));
#23462=CARTESIAN_POINT('Ctrl Pts',(0.4990120177814,1.133554353637,-24.17829593715));
#23463=CARTESIAN_POINT('Ctrl Pts',(1.130396613902,0.5061244529163,-24.23679593715));
#23464=CARTESIAN_POINT('Ctrl Pts',(1.177912758794,-0.3827270557762,-24.29529593715));
#23465=CARTESIAN_POINT('Ctrl Pts',(0.6170175817815,-1.073893742571,-24.35379593715));
#23466=CARTESIAN_POINT('Ctrl Pts',(-0.2625773289571,-1.210376640909,-24.41229593715));
#23467=CARTESIAN_POINT('Ctrl Pts',(-1.006546728684,-0.7216800880868,-24.47079593715));
#23468=CARTESIAN_POINT('Ctrl Pts',(-1.230618180878,0.1397761052806,-24.52929593715));
#23469=CARTESIAN_POINT('Ctrl Pts',(-0.8190550931204,0.9290356397707,-24.58779593715));
#23470=CARTESIAN_POINT('Ctrl Pts',(0.01556342629763,1.238432981537,-24.64629593715));
#23471=CARTESIAN_POINT('Ctrl Pts',(0.8421431840371,0.9081593028442,-24.70479593715));
#23472=CARTESIAN_POINT('Ctrl Pts',(1.233742114882,0.1088064295365,-24.76329593715));
#23473=CARTESIAN_POINT('Ctrl Pts',(0.9880929997609,-0.74674686184,-24.82179593715));
#23474=CARTESIAN_POINT('Ctrl Pts',(0.2320773789096,-1.216592712924,-24.88029593715));
#23475=CARTESIAN_POINT('Ctrl Pts',(-0.6438092328589,-1.058049897633,-24.93879593715));
#23476=CARTESIAN_POINT('Ctrl Pts',(-1.187160745576,-0.3530013460875,-24.99729593715));
#23477=CARTESIAN_POINT('Ctrl Pts',(-1.117313139878,0.5343574797989,-25.05579593715));
#23478=CARTESIAN_POINT('Ctrl Pts',(-0.4703961859321,1.145789237877,-25.11429593715));
#23479=CARTESIAN_POINT('Ctrl Pts',(0.4196421724445,1.165113278138,-25.17279593715));
#23480=CARTESIAN_POINT('Ctrl Pts',(0.868116444205,0.7775142046514,-25.21179593715));
#23481=CARTESIAN_POINT('Ctrl Pts',(0.9986747171026,0.5327947305945,-25.23129593715));
#23482=CARTESIAN_POINT('Ctrl Pts',(0.5535193767689,-1.138916214631,-23.43688532136));
#23483=CARTESIAN_POINT('Ctrl Pts',(0.2744345333596,-1.27455294243,-23.45638532136));
#23484=CARTESIAN_POINT('Ctrl Pts',(-0.3863399140639,-1.330453147354,-23.49538532136));
#23485=CARTESIAN_POINT('Ctrl Pts',(-1.179179506419,-0.72769973686,-23.55388532136));
#23486=CARTESIAN_POINT('Ctrl Pts',(-1.362624213149,0.2510825875499,-23.61238532136));
#23487=CARTESIAN_POINT('Ctrl Pts',(-0.8423393194779,1.100133745242,-23.67088532136));
#23488=CARTESIAN_POINT('Ctrl Pts',(0.1130513333539,1.380959210682,-23.72938532136));
#23489=CARTESIAN_POINT('Ctrl Pts',(1.010042777888,0.9484934422207,-23.78788532136));
#23490=CARTESIAN_POINT('Ctrl Pts',(1.385332205172,0.02611602874334,-23.84638532136));
#23491=CARTESIAN_POINT('Ctrl Pts',(1.045074298715,-0.9097509643373,-23.90488532136));
#23492=CARTESIAN_POINT('Ctrl Pts',(0.1650184426333,-1.375716555595,-23.96338532136));
#23493=CARTESIAN_POINT('Ctrl Pts',(-0.8002721870203,-1.131101924998,-24.02188532136));
#23494=CARTESIAN_POINT('Ctrl Pts',(-1.352209055232,-0.3022545341455,-24.08038532136));
#23495=CARTESIAN_POINT('Ctrl Pts',(-1.205707698806,0.682712295908,-24.13888532136));
#23496=CARTESIAN_POINT('Ctrl Pts',(-0.4364384759746,1.315046991726,-24.19738532136));
#23497=CARTESIAN_POINT('Ctrl Pts',(0.5582584009165,1.268138277765,-24.25588532136));
#23498=CARTESIAN_POINT('Ctrl Pts',(1.264605627904,0.5662152767502,-24.31438532136));
#23499=CARTESIAN_POINT('Ctrl Pts',(1.317763239585,-0.4281672315128,-24.37288532136));
#23500=CARTESIAN_POINT('Ctrl Pts',(0.6902744548601,-1.201394319414,-24.43138532136));
#23501=CARTESIAN_POINT('Ctrl Pts',(-0.2937524439436,-1.354081472956,-24.48988532136));
#23502=CARTESIAN_POINT('Ctrl Pts',(-1.12605137187,-0.8073632649967,-24.54838532136));
#23503=CARTESIAN_POINT('Ctrl Pts',(-1.376726237677,0.1563713542756,-24.60688532136));
#23504=CARTESIAN_POINT('Ctrl Pts',(-0.9162993480212,1.039337595432,-24.66538532136));
#23505=CARTESIAN_POINT('Ctrl Pts',(0.01741123092852,1.385468869044,-24.72388532136));
#23506=CARTESIAN_POINT('Ctrl Pts',(0.9421286271891,1.015982665983,-24.78238532136));
#23507=CARTESIAN_POINT('Ctrl Pts',(1.380221068141,0.1217247304635,-24.84088532136));
#23508=CARTESIAN_POINT('Ctrl Pts',(1.105406680295,-0.8354061508049,-24.89938532136));
#23509=CARTESIAN_POINT('Ctrl Pts',(0.2596313151233,-1.361035562837,-24.95788532136));
#23510=CARTESIAN_POINT('Ctrl Pts',(-0.7202470081362,-1.183669376478,-25.01638532136));
#23511=CARTESIAN_POINT('Ctrl Pts',(-1.32810921549,-0.3949122665708,-25.07488532136));
#23512=CARTESIAN_POINT('Ctrl Pts',(-1.249968787454,0.5978003365862,-25.13338532136));
#23513=CARTESIAN_POINT('Ctrl Pts',(-0.5262450866879,1.2818257776,-25.19188532136));
#23514=CARTESIAN_POINT('Ctrl Pts',(0.4694651827977,1.303444110288,-25.25038532136));
#23515=CARTESIAN_POINT('Ctrl Pts',(0.9711856241576,0.8698264192279,-25.28938532136));
#23516=CARTESIAN_POINT('Ctrl Pts',(1.117244737079,0.5960520462829,-25.30888532136));
#23517=CARTESIAN_POINT('Ctrl Pts',(0.6122628206918,-1.259786167148,-23.51447470556));
#23518=CARTESIAN_POINT('Ctrl Pts',(0.303559493203,-1.409817636753,-23.53397470556));
#23519=CARTESIAN_POINT('Ctrl Pts',(-0.4273410750521,-1.471650372119,-23.57297470556));
#23520=CARTESIAN_POINT('Ctrl Pts',(-1.304322488069,-0.804928449131,-23.63147470556));
#23521=CARTESIAN_POINT('Ctrl Pts',(-1.507235662021,0.2777292715157,-23.68997470556));
#23522=CARTESIAN_POINT('Ctrl Pts',(-0.9317344059998,1.216887824112,-23.74847470556));
#23523=CARTESIAN_POINT('Ctrl Pts',(0.1250491512082,1.527516500918,-23.80697470556));
#23524=CARTESIAN_POINT('Ctrl Pts',(1.117235757524,1.049154365167,-23.86547470556));
#23525=CARTESIAN_POINT('Ctrl Pts',(1.53235358893,0.02888764891485,-23.92397470556));
#23526=CARTESIAN_POINT('Ctrl Pts',(1.15598507445,-1.006300257822,-23.98247470556));
#23527=CARTESIAN_POINT('Ctrl Pts',(0.1825313826277,-1.521717457694,-24.04097470556));
#23528=CARTESIAN_POINT('Ctrl Pts',(-0.8852028079061,-1.251142569086,-24.09947470556));
#23529=CARTESIAN_POINT('Ctrl Pts',(-1.495715172889,-0.3343319518877,-24.15797470556));
#23530=CARTESIAN_POINT('Ctrl Pts',(-1.333666042389,0.7551666184726,-24.21647470556));
#23531=CARTESIAN_POINT('Ctrl Pts',(-0.4827564554623,1.454609204823,-24.27497470556));
#23532=CARTESIAN_POINT('Ctrl Pts',(0.6175047840515,1.402722201892,-24.33347470556));
#23533=CARTESIAN_POINT('Ctrl Pts',(1.398814641906,0.6263061005841,-24.39197470556));
#23534=CARTESIAN_POINT('Ctrl Pts',(1.457613720376,-0.4736074072494,-24.45047470556));
#23535=CARTESIAN_POINT('Ctrl Pts',(0.7635313279386,-1.328894896257,-24.50897470556));
#23536=CARTESIAN_POINT('Ctrl Pts',(-0.3249275589301,-1.497786305004,-24.56747470556));
#23537=CARTESIAN_POINT('Ctrl Pts',(-1.245556015057,-0.8930464419066,-24.62597470556));
#23538=CARTESIAN_POINT('Ctrl Pts',(-1.522834294475,0.1729666032706,-24.68447470556));
#23539=CARTESIAN_POINT('Ctrl Pts',(-1.013543602922,1.149639551094,-24.74297470556));
#23540=CARTESIAN_POINT('Ctrl Pts',(0.01925903555941,1.532504756551,-24.80147470556));
#23541=CARTESIAN_POINT('Ctrl Pts',(1.042114070341,1.123806029122,-24.85997470556));
#23542=CARTESIAN_POINT('Ctrl Pts',(1.5267000214,0.1346430313905,-24.91847470556));
#23543=CARTESIAN_POINT('Ctrl Pts',(1.22272036083,-0.9240654397699,-24.97697470556));
#23544=CARTESIAN_POINT('Ctrl Pts',(0.2871852513371,-1.50547841275,-25.03547470556));
#23545=CARTESIAN_POINT('Ctrl Pts',(-0.7966847834135,-1.309288855323,-25.09397470556));
#23546=CARTESIAN_POINT('Ctrl Pts',(-1.469057685405,-0.4368231870542,-25.15247470556));
#23547=CARTESIAN_POINT('Ctrl Pts',(-1.38262443503,0.6612431933735,-25.21097470556));
#23548=CARTESIAN_POINT('Ctrl Pts',(-0.5820939874436,1.417862317323,-25.26947470556));
#23549=CARTESIAN_POINT('Ctrl Pts',(0.5192881931508,1.441774942437,-25.32797470556));
#23550=CARTESIAN_POINT('Ctrl Pts',(1.07425480411,0.9621386338044,-25.36697470556));
#23551=CARTESIAN_POINT('Ctrl Pts',(1.235814757055,0.6593093619714,-25.38647470556));
#23552=CARTESIAN_POINT('Ctrl Pts',(0.6710062646147,-1.380656119664,-23.59206408977));
#23553=CARTESIAN_POINT('Ctrl Pts',(0.3326844530463,-1.545082331076,-23.61156408977));
#23554=CARTESIAN_POINT('Ctrl Pts',(-0.4683422360403,-1.612847596885,-23.65056408977));
#23555=CARTESIAN_POINT('Ctrl Pts',(-1.42946546972,-0.8821571614021,-23.70906408977));
#23556=CARTESIAN_POINT('Ctrl Pts',(-1.651847110892,0.3043759554816,-23.76756408977));
#23557=CARTESIAN_POINT('Ctrl Pts',(-1.021129492522,1.333641902982,-23.82606408977));
#23558=CARTESIAN_POINT('Ctrl Pts',(0.1370469690624,1.674073791154,-23.88456408977));
#23559=CARTESIAN_POINT('Ctrl Pts',(1.224428737161,1.149815288114,-23.94306408977));
#23560=CARTESIAN_POINT('Ctrl Pts',(1.679374972687,0.03165926908636,-24.00156408977));
#23561=CARTESIAN_POINT('Ctrl Pts',(1.266895850185,-1.102849551308,-24.06006408977));
#23562=CARTESIAN_POINT('Ctrl Pts',(0.2000443226221,-1.667718359793,-24.11856408977));
#23563=CARTESIAN_POINT('Ctrl Pts',(-0.9701334287918,-1.371183213173,-24.17706408977));
#23564=CARTESIAN_POINT('Ctrl Pts',(-1.639221290546,-0.3664093696299,-24.23556408977));
#23565=CARTESIAN_POINT('Ctrl Pts',(-1.461624385972,0.8276209410372,-24.29406408977));
#23566=CARTESIAN_POINT('Ctrl Pts',(-0.52907443495,1.594171417921,-24.35256408977));
#23567=CARTESIAN_POINT('Ctrl Pts',(0.6767511671866,1.53730612602,-24.41106408977));
#23568=CARTESIAN_POINT('Ctrl Pts',(1.533023655909,0.686396924418,-24.46956408977));
#23569=CARTESIAN_POINT('Ctrl Pts',(1.597464201167,-0.519047582986,-24.52806408977));
#23570=CARTESIAN_POINT('Ctrl Pts',(0.8367882010172,-1.456395473099,-24.58656408977));
#23571=CARTESIAN_POINT('Ctrl Pts',(-0.3561026739166,-1.641491137051,-24.64506408977));
#23572=CARTESIAN_POINT('Ctrl Pts',(-1.365060658244,-0.9787296188165,-24.70356408977));
#23573=CARTESIAN_POINT('Ctrl Pts',(-1.668942351274,0.1895618522656,-24.76206408977));
#23574=CARTESIAN_POINT('Ctrl Pts',(-1.110787857823,1.259941506756,-24.82056408977));
#23575=CARTESIAN_POINT('Ctrl Pts',(0.02110684019029,1.679540644058,-24.87906408977));
#23576=CARTESIAN_POINT('Ctrl Pts',(1.142099513493,1.231629392261,-24.93756408977));
#23577=CARTESIAN_POINT('Ctrl Pts',(1.673178974659,0.1475613323174,-24.99606408977));
#23578=CARTESIAN_POINT('Ctrl Pts',(1.340034041364,-1.012724728735,-25.05456408977));
#23579=CARTESIAN_POINT('Ctrl Pts',(0.3147391875509,-1.649921262663,-25.11306408977));
#23580=CARTESIAN_POINT('Ctrl Pts',(-0.8731225586908,-1.434908334168,-25.17156408977));
#23581=CARTESIAN_POINT('Ctrl Pts',(-1.610006155319,-0.4787341075376,-25.23006408977));
#23582=CARTESIAN_POINT('Ctrl Pts',(-1.515280082606,0.7246860501608,-25.28856408977));
#23583=CARTESIAN_POINT('Ctrl Pts',(-0.6379428881994,1.553898857047,-25.34706408977));
#23584=CARTESIAN_POINT('Ctrl Pts',(0.569111203504,1.580105774587,-25.40556408977));
#23585=CARTESIAN_POINT('Ctrl Pts',(1.177323984063,1.054450848381,-25.44456408977));
#23586=CARTESIAN_POINT('Ctrl Pts',(1.354384777031,0.7225666776598,-25.46406408977));
#23587=CARTESIAN_POINT('',(0.88141761294346,1.21316727086581,-25.4075569156963));
#23588=CARTESIAN_POINT('Ctrl Pts',(0.881272060753893,1.21292427294373,-24.9076008241125));
#23589=CARTESIAN_POINT('Ctrl Pts',(0.996854232029655,1.12941607459641,-24.9151108232887));
#23590=CARTESIAN_POINT('Ctrl Pts',(1.09903748426639,1.03061271571212,-24.922888098466));
#23591=CARTESIAN_POINT('Ctrl Pts',(1.26828247410366,0.81113931730235,-24.9378733243509));
#23592=CARTESIAN_POINT('Ctrl Pts',(1.33595204838605,0.692845852390926,-24.9448956623844));
#23593=CARTESIAN_POINT('Ctrl Pts',(1.42935208810126,0.46448502774489,-24.9576888333645));
#23594=CARTESIAN_POINT('Ctrl Pts',(1.46035128052924,0.356433930622584,-24.9634772614354));
#23595=CARTESIAN_POINT('Ctrl Pts',(1.49775994046669,0.13564250301949,-24.975383500877));
#23596=CARTESIAN_POINT('Ctrl Pts',(1.50382443165145,0.0241606386654887,
-24.9815225190637));
#23597=CARTESIAN_POINT('Ctrl Pts',(1.48757937945927,-0.248131031019487,
-24.9963697308979));
#23598=CARTESIAN_POINT('Ctrl Pts',(1.45140820792574,-0.40686417356901,-25.0046989308054));
#23599=CARTESIAN_POINT('Ctrl Pts',(1.34071624949762,-0.684366848185125,
-25.0201942046533));
#23600=CARTESIAN_POINT('Ctrl Pts',(1.27196490382923,-0.806121698603482,
-25.0274086698495));
#23601=CARTESIAN_POINT('Ctrl Pts',(1.12526332452217,-0.996878599573301,
-25.0404730867428));
#23602=CARTESIAN_POINT('Ctrl Pts',(1.055053532006,-1.07084246642367,-25.0460952204423));
#23603=CARTESIAN_POINT('Ctrl Pts',(0.900866720644833,-1.20260014134437,
-25.0569359673065));
#23604=CARTESIAN_POINT('Ctrl Pts',(0.818038542621622,-1.26002586650043,
-25.062163772409));
#23605=CARTESIAN_POINT('Ctrl Pts',(0.627936459696357,-1.36593650206767,
-25.0734565570246));
#23606=CARTESIAN_POINT('Ctrl Pts',(0.518806191168035,-1.41129028572528,
-25.0795222275456));
#23607=CARTESIAN_POINT('Ctrl Pts',(0.29457123980294,-1.47502535777107,-25.091885171377));
#23608=CARTESIAN_POINT('Ctrl Pts',(0.180846817453055,-1.49338989670108,
-25.0982048412207));
#23609=CARTESIAN_POINT('Ctrl Pts',(-0.0801360635283695,-1.50447944522687,
-25.1124180147734));
#23610=CARTESIAN_POINT('Ctrl Pts',(-0.22643540767658,-1.48879367987403,
-25.1200025038582));
#23611=CARTESIAN_POINT('Ctrl Pts',(-0.475813301844074,-1.42568036311793,
-25.1333434648599));
#23612=CARTESIAN_POINT('Ctrl Pts',(-0.581342893248654,-1.38632056710971,
-25.1391417409856));
#23613=CARTESIAN_POINT('Ctrl Pts',(-0.780638853926507,-1.28537566237664,
-25.1510164952203));
#23614=CARTESIAN_POINT('Ctrl Pts',(-0.87329259886436,-1.22445335145697,
-25.1571101120661));
#23615=CARTESIAN_POINT('Ctrl Pts',(-1.05143659264298,-1.07599275375337,
-25.1697221953949));
#23616=CARTESIAN_POINT('Ctrl Pts',(-1.13447948010956,-0.98723527130443,
-25.1760565796546));
#23617=CARTESIAN_POINT('Ctrl Pts',(-1.31542362877098,-0.74146902433613,
-25.1919170784518));
#23618=CARTESIAN_POINT('Ctrl Pts',(-1.39834713694402,-0.572369695431689,
-25.2014459946615));
#23619=CARTESIAN_POINT('Ctrl Pts',(-1.47766193566027,-0.281894798315009,
-25.2178464657796));
#23620=CARTESIAN_POINT('Ctrl Pts',(-1.49474758269074,-0.167816718099114,
-25.224163502727));
#23621=CARTESIAN_POINT('Ctrl Pts',(-1.50224798014019,0.0671521060380822,
-25.2366170198868));
#23622=CARTESIAN_POINT('Ctrl Pts',(-1.49184489770568,0.186787458005913,
-25.2427734719892));
#23623=CARTESIAN_POINT('Ctrl Pts',(-1.44764485166995,0.401517274028821,
-25.2541548609197));
#23624=CARTESIAN_POINT('Ctrl Pts',(-1.41786426926399,0.497540003891422,
-25.2593772772489));
#23625=CARTESIAN_POINT('Ctrl Pts',(-1.34056704157422,0.679550937711682,
-25.2699691425619));
#23626=CARTESIAN_POINT('Ctrl Pts',(-1.29385520043036,0.764820066777107,
-25.2753309368534));
#23627=CARTESIAN_POINT('Ctrl Pts',(-1.15764425661784,0.963893360333778,
-25.2884292940504));
#23628=CARTESIAN_POINT('Ctrl Pts',(-1.0589086197412,1.07051008241031,-25.2959099928094));
#23629=CARTESIAN_POINT('Ctrl Pts',(-0.823750133175226,1.2623201806948,-25.3116467956406));
#23630=CARTESIAN_POINT('Ctrl Pts',(-0.68372051272252,1.34425016727509,-25.3199680385646));
#23631=CARTESIAN_POINT('Ctrl Pts',(-0.423365338694491,1.44370500948602,
-25.3351649382959));
#23632=CARTESIAN_POINT('Ctrl Pts',(-0.308952727975757,1.47222251714957,
-25.3416186189514));
#23633=CARTESIAN_POINT('Ctrl Pts',(-0.071322839538722,1.50214058415113,
-25.3542951995422));
#23634=CARTESIAN_POINT('Ctrl Pts',(0.0507139592723535,1.50274269520359,
-25.3605452492806));
#23635=CARTESIAN_POINT('Ctrl Pts',(0.295625083841534,1.47490327186699,-25.3733440948517));
#23636=CARTESIAN_POINT('Ctrl Pts',(0.418716827588455,1.44539674806488,-25.3799246413091));
#23637=CARTESIAN_POINT('Ctrl Pts',(0.659291920030595,1.35366265978716,-25.3939167140426));
#23638=CARTESIAN_POINT('Ctrl Pts',(0.774758582836638,1.29074282062916,-25.4010793596211));
#23639=CARTESIAN_POINT('Ctrl Pts',(0.881231260302741,1.2129539171392,-25.4080241608977));
#23640=CARTESIAN_POINT('',(0.6859379234404,0.9441125563889,-25.21554752692));
#23641=CARTESIAN_POINT('Ctrl Pts',(0.1981104409423,1.114438723627,-25.15929593715));
#23642=CARTESIAN_POINT('Ctrl Pts',(0.47119721649,1.065892903769,-25.17879593715));
#23643=CARTESIAN_POINT('Ctrl Pts',(0.9784120125535,0.7591432259322,-25.21779593715));
#23644=CARTESIAN_POINT('Ctrl Pts',(1.235070736526,-0.09330501139523,-25.27629593715));
#23645=CARTESIAN_POINT('Ctrl Pts',(0.8534729114545,-0.8975024000936,-25.33479593715));
#23646=CARTESIAN_POINT('Ctrl Pts',(0.03112861498029,-1.238140377948,-25.39329593715));
#23647=CARTESIAN_POINT('Ctrl Pts',(-0.80731725562,-0.9392543654266,-25.45179593715));
#23648=CARTESIAN_POINT('Ctrl Pts',(-1.228764281396,-0.1552291200295,-25.51029593715));
#23649=CARTESIAN_POINT('Ctrl Pts',(-1.015535997925,0.7089748153235,-25.56879593715));
#23650=CARTESIAN_POINT('Ctrl Pts',(-0.2777662163492,1.206981513611,-25.62729593715));
#23651=CARTESIAN_POINT('Ctrl Pts',(0.6034742672396,1.081562421011,-25.68579593715));
#23652=CARTESIAN_POINT('Ctrl Pts',(1.173010393869,0.3974985356856,-25.74429593715));
#23653=CARTESIAN_POINT('Ctrl Pts',(1.136667342178,-0.4918798824477,-25.80279593715));
#23654=CARTESIAN_POINT('Ctrl Pts',(0.5132169072275,-1.127194248056,-25.86129593715));
#23655=CARTESIAN_POINT('Ctrl Pts',(-0.3753185056597,-1.180294236991,-25.91979593715));
#23656=CARTESIAN_POINT('Ctrl Pts',(-1.069995734522,-0.6237528313713,-25.97829593715));
#23657=CARTESIAN_POINT('Ctrl Pts',(-1.212002560279,0.2549671752147,-26.03679593715));
#23658=CARTESIAN_POINT('Ctrl Pts',(-0.7279901207168,1.001992440436,-26.09529593715));
#23659=CARTESIAN_POINT('Ctrl Pts',(0.1320411949229,1.231472122869,-26.15379593715));
#23660=CARTESIAN_POINT('Ctrl Pts',(0.9238710607093,0.8248761905421,-26.21229593715));
#23661=CARTESIAN_POINT('Ctrl Pts',(1.238506321788,-0.007781867099203,-26.27079593715));
#23662=CARTESIAN_POINT('Ctrl Pts',(0.9134326886102,-0.8364204625026,-26.32929593715));
#23663=CARTESIAN_POINT('Ctrl Pts',(0.1165560417524,-1.233034125506,-26.38779593715));
#23664=CARTESIAN_POINT('Ctrl Pts',(-0.7405237188655,-0.992765376005,-26.44629593715));
#23665=CARTESIAN_POINT('Ctrl Pts',(-1.215110792527,-0.2397169657051,-26.50479593715));
#23666=CARTESIAN_POINT('Ctrl Pts',(-1.062073152252,0.6371491696676,-26.56329593715));
#23667=CARTESIAN_POINT('Ctrl Pts',(-0.3604572362442,1.184917394878,-26.62179593715));
#23668=CARTESIAN_POINT('Ctrl Pts',(0.5273407111552,1.120655840702,-26.68029593715));
#23669=CARTESIAN_POINT('Ctrl Pts',(1.142758736536,0.4775587757172,-26.73879593715));
#23670=CARTESIAN_POINT('Ctrl Pts',(1.167922203495,-0.412211490328,-26.79729593715));
#23671=CARTESIAN_POINT('Ctrl Pts',(0.5898378721215,-1.089044468041,-26.85579593715));
#23672=CARTESIAN_POINT('Ctrl Pts',(-0.2929195077513,-1.20345490624,-26.91429593715));
#23673=CARTESIAN_POINT('Ctrl Pts',(-1.024334051204,-0.6959369621828,-26.97279593715));
#23674=CARTESIAN_POINT('Ctrl Pts',(-1.1593323394,-0.1187561617546,-27.01179593715));
#23675=CARTESIAN_POINT('Ctrl Pts',(-1.121113703131,0.1559662789859,-27.03129593715));
#23676=CARTESIAN_POINT('Ctrl Pts',(0.2216315720351,1.246753099329,-25.23688532136));
#23677=CARTESIAN_POINT('Ctrl Pts',(0.527141221495,1.192443562085,-25.25638532136));
#23678=CARTESIAN_POINT('Ctrl Pts',(1.094576294964,0.8492743025702,-25.29538532136));
#23679=CARTESIAN_POINT('Ctrl Pts',(1.381707433535,-0.1043828697565,-25.35388532136));
#23680=CARTESIAN_POINT('Ctrl Pts',(0.9548035033152,-1.004060497225,-25.41238532136));
#23681=CARTESIAN_POINT('Ctrl Pts',(0.03482443348539,-1.385141525401,-25.47088532136));
#23682=CARTESIAN_POINT('Ctrl Pts',(-0.9031679079763,-1.050769563483,-25.52938532136));
#23683=CARTESIAN_POINT('Ctrl Pts',(-1.37465222959,-0.1736590647829,-25.58788532136));
#23684=CARTESIAN_POINT('Ctrl Pts',(-1.136107913383,0.793149528647,-25.64638532136));
#23685=CARTESIAN_POINT('Ctrl Pts',(-0.3107446679484,1.350283251132,-25.70488532136));
#23686=CARTESIAN_POINT('Ctrl Pts',(0.6751231782377,1.209973479856,-25.76338532136));
#23687=CARTESIAN_POINT('Ctrl Pts',(1.312278829779,0.4446924903434,-25.82188532136));
#23688=CARTESIAN_POINT('Ctrl Pts',(1.27162086324,-0.5502794859312,-25.88038532136));
#23689=CARTESIAN_POINT('Ctrl Pts',(0.5741497994896,-1.261023053592,-25.93888532136));
#23690=CARTESIAN_POINT('Ctrl Pts',(-0.4198790837452,-1.320427464418,-25.99738532136));
#23691=CARTESIAN_POINT('Ctrl Pts',(-1.197033511132,-0.6978093629019,-26.05588532136));
#23692=CARTESIAN_POINT('Ctrl Pts',(-1.355900433453,0.2852387566824,-26.11438532136));
#23693=CARTESIAN_POINT('Ctrl Pts',(-0.8144224711886,1.120956364969,-26.17288532136));
#23694=CARTESIAN_POINT('Ctrl Pts',(0.1477180983746,1.377681565952,-26.23138532136));
#23695=CARTESIAN_POINT('Ctrl Pts',(1.033559839496,0.9228115690148,-26.28988532136));
#23696=CARTESIAN_POINT('Ctrl Pts',(1.38555091679,-0.008705787692768,-26.34838532136));
#23697=CARTESIAN_POINT('Ctrl Pts',(1.021882146958,-0.9357264619928,-26.40688532136));
#23698=CARTESIAN_POINT('Ctrl Pts',(0.1303944337356,-1.37942902105,-26.46538532136));
#23699=CARTESIAN_POINT('Ctrl Pts',(-0.8284441504486,-1.11063379547,-26.52388532136));
#23700=CARTESIAN_POINT('Ctrl Pts',(-1.359377697933,-0.2681779299465,-26.58238532136));
#23701=CARTESIAN_POINT('Ctrl Pts',(-1.188170301526,0.712796213176,-26.64088532136));
#23702=CARTESIAN_POINT('Ctrl Pts',(-0.403253374937,1.32559951767,-26.69938532136));
#23703=CARTESIAN_POINT('Ctrl Pts',(0.5899504854742,1.253708358346,-26.75788532136));
#23704=CARTESIAN_POINT('Ctrl Pts',(1.278435472814,0.5342580719014,-26.81638532136));
#23705=CARTESIAN_POINT('Ctrl Pts',(1.306586531957,-0.461152275356,-26.87488532136));
#23706=CARTESIAN_POINT('Ctrl Pts',(0.6598677698274,-1.218343850632,-26.93338532136));
#23707=CARTESIAN_POINT('Ctrl Pts',(-0.3276970697449,-1.346337938953,-26.99188532136));
#23708=CARTESIAN_POINT('Ctrl Pts',(-1.145950536365,-0.7785637255274,-27.05038532136));
#23709=CARTESIAN_POINT('Ctrl Pts',(-1.296976815913,-0.1328557681934,-27.08938532136));
#23710=CARTESIAN_POINT('Ctrl Pts',(-1.254220581577,0.1744837446815,-27.10888532136));
#23711=CARTESIAN_POINT('Ctrl Pts',(0.2451527031279,1.379067475031,-25.31447470556));
#23712=CARTESIAN_POINT('Ctrl Pts',(0.5830852265001,1.318994220401,-25.33397470556));
#23713=CARTESIAN_POINT('Ctrl Pts',(1.210740577374,0.9394053792083,-25.37297470556));
#23714=CARTESIAN_POINT('Ctrl Pts',(1.528344130543,-0.1154607281177,-25.43147470556));
#23715=CARTESIAN_POINT('Ctrl Pts',(1.056134095176,-1.110618594357,-25.48997470556));
#23716=CARTESIAN_POINT('Ctrl Pts',(0.03852025199049,-1.532142672854,-25.54847470556));
#23717=CARTESIAN_POINT('Ctrl Pts',(-0.9990185603326,-1.162284761539,-25.60697470556));
#23718=CARTESIAN_POINT('Ctrl Pts',(-1.520540177784,-0.1920890095362,-25.66547470556));
#23719=CARTESIAN_POINT('Ctrl Pts',(-1.256679828841,0.8773242419706,-25.72397470556));
#23720=CARTESIAN_POINT('Ctrl Pts',(-0.3437231195475,1.493584988654,-25.78247470556));
#23721=CARTESIAN_POINT('Ctrl Pts',(0.7467720892358,1.3383845387,-25.84097470556));
#23722=CARTESIAN_POINT('Ctrl Pts',(1.451547265688,0.4918864450011,-25.89947470556));
#23723=CARTESIAN_POINT('Ctrl Pts',(1.406574384301,-0.6086790894146,-25.95797470556));
#23724=CARTESIAN_POINT('Ctrl Pts',(0.6350826917518,-1.394851859129,-26.01647470556));
#23725=CARTESIAN_POINT('Ctrl Pts',(-0.4644396618308,-1.460560691846,-26.07497470556));
#23726=CARTESIAN_POINT('Ctrl Pts',(-1.324071287741,-0.7718658944325,-26.13347470556));
#23727=CARTESIAN_POINT('Ctrl Pts',(-1.499798306627,0.3155103381501,-26.19197470556));
#23728=CARTESIAN_POINT('Ctrl Pts',(-0.9008548216604,1.239920289503,-26.25047470556));
#23729=CARTESIAN_POINT('Ctrl Pts',(0.1633950018263,1.523891009035,-26.30897470556));
#23730=CARTESIAN_POINT('Ctrl Pts',(1.143248618282,1.020746947487,-26.36747470556));
#23731=CARTESIAN_POINT('Ctrl Pts',(1.532595511792,-0.009629708286341,-26.42597470556));
#23732=CARTESIAN_POINT('Ctrl Pts',(1.130331605306,-1.035032461483,-26.48447470556));
#23733=CARTESIAN_POINT('Ctrl Pts',(0.1442328257187,-1.525823916594,-26.54297470556));
#23734=CARTESIAN_POINT('Ctrl Pts',(-0.9163645820317,-1.228502214935,-26.60147470556));
#23735=CARTESIAN_POINT('Ctrl Pts',(-1.503644603339,-0.296638894188,-26.65997470556));
#23736=CARTESIAN_POINT('Ctrl Pts',(-1.3142674508,0.7884432566844,-26.71847470556));
#23737=CARTESIAN_POINT('Ctrl Pts',(-0.4460495136298,1.466281640462,-26.77697470556));
#23738=CARTESIAN_POINT('Ctrl Pts',(0.6525602597933,1.386760875991,-26.83547470556));
#23739=CARTESIAN_POINT('Ctrl Pts',(1.414112209091,0.5909573680856,-26.89397470556));
#23740=CARTESIAN_POINT('Ctrl Pts',(1.445250860419,-0.510093060384,-26.95247470556));
#23741=CARTESIAN_POINT('Ctrl Pts',(0.7298976675333,-1.347643233224,-27.01097470556));
#23742=CARTESIAN_POINT('Ctrl Pts',(-0.3624746317386,-1.489220971666,-27.06947470556));
#23743=CARTESIAN_POINT('Ctrl Pts',(-1.267567021527,-0.8611904888719,-27.12797470556));
#23744=CARTESIAN_POINT('Ctrl Pts',(-1.434621292425,-0.1469553746322,-27.16697470556));
#23745=CARTESIAN_POINT('Ctrl Pts',(-1.387327460022,0.193001210377,-27.18647470556));
#23746=CARTESIAN_POINT('Ctrl Pts',(0.2686738342207,1.511381850733,-25.39206408977));
#23747=CARTESIAN_POINT('Ctrl Pts',(0.6390292315051,1.445544878716,-25.41156408977));
#23748=CARTESIAN_POINT('Ctrl Pts',(1.326904859784,1.029536455846,-25.45056408977));
#23749=CARTESIAN_POINT('Ctrl Pts',(1.674980827552,-0.126538586479,-25.50906408977));
#23750=CARTESIAN_POINT('Ctrl Pts',(1.157464687037,-1.217176691488,-25.56756408977));
#23751=CARTESIAN_POINT('Ctrl Pts',(0.0422160704956,-1.679143820308,-25.62606408977));
#23752=CARTESIAN_POINT('Ctrl Pts',(-1.094869212689,-1.273799959595,-25.68456408977));
#23753=CARTESIAN_POINT('Ctrl Pts',(-1.666428125978,-0.2105189542896,-25.74306408977));
#23754=CARTESIAN_POINT('Ctrl Pts',(-1.377251744299,0.9614989552941,-25.80156408977));
#23755=CARTESIAN_POINT('Ctrl Pts',(-0.3767015711467,1.636886726176,-25.86006408977));
#23756=CARTESIAN_POINT('Ctrl Pts',(0.818421000234,1.466795597545,-25.91856408977));
#23757=CARTESIAN_POINT('Ctrl Pts',(1.590815701598,0.5390803996589,-25.97706408977));
#23758=CARTESIAN_POINT('Ctrl Pts',(1.541527905363,-0.6670786928981,-26.03556408977));
#23759=CARTESIAN_POINT('Ctrl Pts',(0.6960155840139,-1.528680664665,-26.09406408977));
#23760=CARTESIAN_POINT('Ctrl Pts',(-0.5090002399164,-1.600693919274,-26.15256408977));
#23761=CARTESIAN_POINT('Ctrl Pts',(-1.451109064351,-0.8459224259631,-26.21106408977));
#23762=CARTESIAN_POINT('Ctrl Pts',(-1.643696179801,0.3457819196178,-26.26956408977));
#23763=CARTESIAN_POINT('Ctrl Pts',(-0.9872871721321,1.358884214036,-26.32806408977));
#23764=CARTESIAN_POINT('Ctrl Pts',(0.179071905278,1.670100452118,-26.38656408977));
#23765=CARTESIAN_POINT('Ctrl Pts',(1.252937397068,1.11868232596,-26.44506408977));
#23766=CARTESIAN_POINT('Ctrl Pts',(1.679640106794,-0.01055362887991,-26.50356408977));
#23767=CARTESIAN_POINT('Ctrl Pts',(1.238781063654,-1.134338460973,-26.56206408977));
#23768=CARTESIAN_POINT('Ctrl Pts',(0.1580712177019,-1.672218812138,-26.62056408977));
#23769=CARTESIAN_POINT('Ctrl Pts',(-1.004285013615,-1.3463706344,-26.67906408977));
#23770=CARTESIAN_POINT('Ctrl Pts',(-1.647911508744,-0.3250998584294,-26.73756408977));
#23771=CARTESIAN_POINT('Ctrl Pts',(-1.440364600074,0.8640903001927,-26.79606408977));
#23772=CARTESIAN_POINT('Ctrl Pts',(-0.4888456523225,1.606963763254,-26.85456408977));
#23773=CARTESIAN_POINT('Ctrl Pts',(0.7151700341124,1.519813393635,-26.91306408977));
#23774=CARTESIAN_POINT('Ctrl Pts',(1.549788945368,0.6476566642697,-26.97156408977));
#23775=CARTESIAN_POINT('Ctrl Pts',(1.583915188882,-0.559033845412,-27.03006408977));
#23776=CARTESIAN_POINT('Ctrl Pts',(0.7999275652393,-1.476942615815,-27.08856408977));
#23777=CARTESIAN_POINT('Ctrl Pts',(-0.3972521937322,-1.632104004379,-27.14706408977));
#23778=CARTESIAN_POINT('Ctrl Pts',(-1.389183506688,-0.9438172522165,-27.20556408977));
#23779=CARTESIAN_POINT('Ctrl Pts',(-1.572265768938,-0.161054981071,-27.24456408977));
#23780=CARTESIAN_POINT('Ctrl Pts',(-1.520434338468,0.2115186760726,-27.26406408977));
#23781=CARTESIAN_POINT('',(-1.42616365985445,-0.463388660650263,-26.7080680843046));
#23782=CARTESIAN_POINT('Ctrl Pts',(0.881253915032725,1.21298308849533,-25.4080029023648));
#23783=CARTESIAN_POINT('Ctrl Pts',(0.948747205053193,1.16388095517069,-25.4123014309742));
#23784=CARTESIAN_POINT('Ctrl Pts',(1.01215734643154,1.10916455955355,-25.4165388040928));
#23785=CARTESIAN_POINT('Ctrl Pts',(1.11653475356739,1.0027866261975,-25.4242292869111));
#23786=CARTESIAN_POINT('Ctrl Pts',(1.15943877346581,0.952944924722898,-25.4276606152218));
#23787=CARTESIAN_POINT('Ctrl Pts',(1.25513297297284,0.825512929642758,-25.4362277693364));
#23788=CARTESIAN_POINT('Ctrl Pts',(1.30428073799585,0.745337850901385,-25.4414340950019));
#23789=CARTESIAN_POINT('Ctrl Pts',(1.37248032915429,0.60659522353523,-25.4499560923802));
#23790=CARTESIAN_POINT('Ctrl Pts',(1.39606039550318,0.55021426433255,-25.4532986464789));
#23791=CARTESIAN_POINT('Ctrl Pts',(1.45534760596076,0.379668230731732,-25.4629595930959));
#23792=CARTESIAN_POINT('Ctrl Pts',(1.48087684845796,0.262130059911762,-25.4690181210202));
#23793=CARTESIAN_POINT('Ctrl Pts',(1.49896284899431,0.0744882692565386,
-25.4786488460513));
#23794=CARTESIAN_POINT('Ctrl Pts',(1.50087122287115,0.0051734444455085,
-25.482199931001));
#23795=CARTESIAN_POINT('Ctrl Pts',(1.49311577995529,-0.179378628968762,
-25.4919233531514));
#23796=CARTESIAN_POINT('Ctrl Pts',(1.47475924984555,-0.293780963306843,
-25.4983060220473));
#23797=CARTESIAN_POINT('Ctrl Pts',(1.42687768842866,-0.464801659022707,
-25.5080926753898));
#23798=CARTESIAN_POINT('Ctrl Pts',(1.40618202469664,-0.524156758629176,
-25.5115332595472));
#23799=CARTESIAN_POINT('Ctrl Pts',(1.33629576206914,-0.690000309590655,
-25.5211707534326));
#23800=CARTESIAN_POINT('Ctrl Pts',(1.27800150301672,-0.792455210852014,
-25.5271252390471));
#23801=CARTESIAN_POINT('Ctrl Pts',(1.16686294825516,-0.944010881473911,
-25.5367339393702));
#23802=CARTESIAN_POINT('Ctrl Pts',(1.12086233336162,-0.998286355735829,
-25.5403767034103));
#23803=CARTESIAN_POINT('Ctrl Pts',(0.989045661700086,-1.1330542198356,-25.5502995687537));
#23804=CARTESIAN_POINT('Ctrl Pts',(0.8971946703891,-1.20693269674559,-25.5567947553411));
#23805=CARTESIAN_POINT('Ctrl Pts',(0.74554678902829,-1.30234068942969,-25.5666683706389));
#23806=CARTESIAN_POINT('Ctrl Pts',(0.690722599936893,-1.3322540013091,-25.5700860467031));
#23807=CARTESIAN_POINT('Ctrl Pts',(0.527400614845279,-1.40845860401314,
-25.5797352638084));
#23808=CARTESIAN_POINT('Ctrl Pts',(0.414767928635027,-1.4454651523955,-25.5857194496648));
#23809=CARTESIAN_POINT('Ctrl Pts',(0.230442521142555,-1.48308713066819,
-25.5953359895283));
#23810=CARTESIAN_POINT('Ctrl Pts',(0.160389091951486,-1.49235155293721,
-25.5989543610995));
#23811=CARTESIAN_POINT('Ctrl Pts',(-0.0269482729927231,-1.50373449218106,
-25.608833930586));
#23812=CARTESIAN_POINT('Ctrl Pts',(-0.14427467802895,-1.49691490378518,
-25.615309980205));
#23813=CARTESIAN_POINT('Ctrl Pts',(-0.320435663803831,-1.46603573232472,
-25.6251661227975));
#23814=CARTESIAN_POINT('Ctrl Pts',(-0.381190857378073,-1.45144758868543,
-25.6285854264352));
#23815=CARTESIAN_POINT('Ctrl Pts',(-0.553375930513323,-1.39844997155958,
-25.63823118699));
#23816=CARTESIAN_POINT('Ctrl Pts',(-0.66165399426776,-1.35040561431633,
-25.6442110145844));
#23817=CARTESIAN_POINT('Ctrl Pts',(-0.823592491370934,-1.25473294660535,
-25.6538258085075));
#23818=CARTESIAN_POINT('Ctrl Pts',(-0.881820799163859,-1.21459372231324,
-25.6574471288747));
#23819=CARTESIAN_POINT('Ctrl Pts',(-1.02845778633262,-1.09736796129135,
-25.6673292599762));
#23820=CARTESIAN_POINT('Ctrl Pts',(-1.11090953277994,-1.0136311487283,-25.673804666259));
#23821=CARTESIAN_POINT('Ctrl Pts',(-1.22088174814917,-0.872577001693917,
-25.6836613750646));
#23822=CARTESIAN_POINT('Ctrl Pts',(-1.25617540400088,-0.82099524423784,
-25.6870817080832));
#23823=CARTESIAN_POINT('Ctrl Pts',(-1.34836098934793,-0.666191286462965,
-25.6967284301321));
#23824=CARTESIAN_POINT('Ctrl Pts',(-1.39645522725724,-0.55793791492804,
-25.7027082129281));
#23825=CARTESIAN_POINT('Ctrl Pts',(-1.45241333146443,-0.378360349758196,
-25.7123233593778));
#23826=CARTESIAN_POINT('Ctrl Pts',(-1.46868657398459,-0.309527086480265,
-25.7159451114343));
#23827=CARTESIAN_POINT('Ctrl Pts',(-1.49883862410827,-0.124207863002646,
-25.7258284243131));
#23828=CARTESIAN_POINT('Ctrl Pts',(-1.50383664266925,-0.00678408440194565,
-25.7323046241237));
#23829=CARTESIAN_POINT('Ctrl Pts',(-1.49080266440243,0.171607254565109,
-25.7421618584004));
#23830=CARTESIAN_POINT('Ctrl Pts',(-1.48238670367419,0.233534213274606,
-25.7455819557246));
#23831=CARTESIAN_POINT('Ctrl Pts',(-1.44693248446084,0.410224322075841,
-25.7552307520551));
#23832=CARTESIAN_POINT('Ctrl Pts',(-1.40998370308478,0.522816620307887,
-25.761212572804));
#23833=CARTESIAN_POINT('Ctrl Pts',(-1.33102660310492,0.693560536556842,
-25.7708288393751));
#23834=CARTESIAN_POINT('Ctrl Pts',(-1.29693788925547,0.755510746312485,
-25.7744495618416));
#23835=CARTESIAN_POINT('Ctrl Pts',(-1.19505639779183,0.913108878650343,
-25.7843280172044));
#23836=CARTESIAN_POINT('Ctrl Pts',(-1.12005931210667,1.00350446405672,-25.7908000358875));
#23837=CARTESIAN_POINT('Ctrl Pts',(-0.990794696798901,1.12706282088653,
-25.8006546684764));
#23838=CARTESIAN_POINT('Ctrl Pts',(-0.943003564918622,1.16737140311131,
-25.8040761477679));
#23839=CARTESIAN_POINT('Ctrl Pts',(-0.798069480629218,1.27476199427798,
-25.8137343929126));
#23840=CARTESIAN_POINT('Ctrl Pts',(-0.695012437837789,1.33356033067832,
-25.8197233994126));
#23841=CARTESIAN_POINT('Ctrl Pts',(-0.521828941050238,1.40724748710769,
-25.8293445130506));
#23842=CARTESIAN_POINT('Ctrl Pts',(-0.455042945148829,1.43030527422233,
-25.8329625909461));
#23843=CARTESIAN_POINT('Ctrl Pts',(-0.274113561120321,1.4787555873326,-25.8428226748611));
#23844=CARTESIAN_POINT('Ctrl Pts',(-0.158163903410276,1.49548288672185,
-25.849277389497));
#23845=CARTESIAN_POINT('Ctrl Pts',(0.0203900776809842,1.50051380193253,
-25.8591217185526));
#23846=CARTESIAN_POINT('Ctrl Pts',(0.0829797582305993,1.49837878424183,
-25.8625493155582));
#23847=CARTESIAN_POINT('Ctrl Pts',(0.263360222333621,1.48079426165296,-25.8722540845708));
#23848=CARTESIAN_POINT('Ctrl Pts',(0.379963033263763,1.45506869010588,-25.8782790333735));
#23849=CARTESIAN_POINT('Ctrl Pts',(0.558197182661076,1.39320862390086,-25.8879241287906));
#23850=CARTESIAN_POINT('Ctrl Pts',(0.622912838124379,1.36556959813383,-25.8915286432843));
#23851=CARTESIAN_POINT('Ctrl Pts',(0.787967940386338,1.2808638273995,-25.9012971323364));
#23852=CARTESIAN_POINT('Ctrl Pts',(0.883987225285216,1.21643379367,-25.9076661037997));
#23853=CARTESIAN_POINT('Ctrl Pts',(1.01934069704798,1.10134720045136,-25.9174593264319));
#23854=CARTESIAN_POINT('Ctrl Pts',(1.06479174553287,1.0575007596973,-25.9209173539813));
#23855=CARTESIAN_POINT('Ctrl Pts',(1.18981730196394,0.92051202873792,-25.93085343019));
#23856=CARTESIAN_POINT('Ctrl Pts',(1.26098625819716,0.819986923949259,-25.9370566163374));
#23857=CARTESIAN_POINT('Ctrl Pts',(1.35178546403656,0.652007903132813,-25.9468224726596));
#23858=CARTESIAN_POINT('Ctrl Pts',(1.38037429657283,0.589229391201502,-25.9503606218836));
#23859=CARTESIAN_POINT('Ctrl Pts',(1.44226544638672,0.423877658750142,-25.9596679311729));
#23860=CARTESIAN_POINT('Ctrl Pts',(1.46887074150055,0.31923451481424,-25.9656048447258));
#23861=CARTESIAN_POINT('Ctrl Pts',(1.49346482083203,0.148077541387214,-25.9751425515935));
#23862=CARTESIAN_POINT('Ctrl Pts',(1.49855032812148,0.0823615348455862,
-25.9787596154772));
#23863=CARTESIAN_POINT('Ctrl Pts',(1.5002906590474,-0.0765947816070528,
-25.9872958586034));
#23864=CARTESIAN_POINT('Ctrl Pts',(1.49250160467889,-0.169662813193452,
-25.9920890856491));
#23865=CARTESIAN_POINT('Ctrl Pts',(1.46141131564603,-0.345171139561176,
-26.0012048594846));
#23866=CARTESIAN_POINT('Ctrl Pts',(1.43939852652682,-0.427965168144118,
-26.0055441490584));
#23867=CARTESIAN_POINT('Ctrl Pts',(1.38535767557335,-0.578259379816273,
-26.013876996291));
#23868=CARTESIAN_POINT('Ctrl Pts',(1.35510480727151,-0.645989385614745,
-26.0178480574243));
#23869=CARTESIAN_POINT('Ctrl Pts',(1.27527714079766,-0.794052989329665,
-26.0270564027238));
#23870=CARTESIAN_POINT('Ctrl Pts',(1.22288066943919,-0.87260868724116,-26.0322983947709));
#23871=CARTESIAN_POINT('Ctrl Pts',(1.11488576133415,-1.00554150868028,-26.041616500911));
#23872=CARTESIAN_POINT('Ctrl Pts',(1.06174173650512,-1.06142358200637,-26.0456839391086));
#23873=CARTESIAN_POINT('Ctrl Pts',(0.926636430335163,-1.18318209801484,
-26.055091177317));
#23874=CARTESIAN_POINT('Ctrl Pts',(0.841477682492276,-1.24518505133867,
-26.0603775999692));
#23875=CARTESIAN_POINT('Ctrl Pts',(0.685498525869903,-1.33557195750662,
-26.0696977140141));
#23876=CARTESIAN_POINT('Ctrl Pts',(0.617457126019338,-1.36842541977454,
-26.0736763842373));
#23877=CARTESIAN_POINT('Ctrl Pts',(0.46872051102547,-1.42668206718181,-26.082354879253));
#23878=CARTESIAN_POINT('Ctrl Pts',(0.387881235611041,-1.45073002316929,
-26.0870274468075));
#23879=CARTESIAN_POINT('Ctrl Pts',(0.228505663239964,-1.48393811934091,
-26.0959767891238));
#23880=CARTESIAN_POINT('Ctrl Pts',(0.150177863546774,-1.49392774096055,
-26.1002435028173));
#23881=CARTESIAN_POINT('Ctrl Pts',(-0.00235132932211669,-1.50107685274736,
-26.10824952913));
#23882=CARTESIAN_POINT('Ctrl Pts',(-0.0761386409443736,-1.49908767270109,
-26.1120153566548));
#23883=CARTESIAN_POINT('Ctrl Pts',(-0.261362591202425,-1.48052766734123,
-26.1215250525544));
#23884=CARTESIAN_POINT('Ctrl Pts',(-0.372253221316257,-1.45678768684412,
-26.1272793118747));
#23885=CARTESIAN_POINT('Ctrl Pts',(-0.540398465334221,-1.40008593812626,
-26.1368085074094));
#23886=CARTESIAN_POINT('Ctrl Pts',(-0.600177814013998,-1.37549549714502,
-26.140354478175));
#23887=CARTESIAN_POINT('Ctrl Pts',(-0.761433663825177,-1.29670566194455,
-26.1502529407966));
#23888=CARTESIAN_POINT('Ctrl Pts',(-0.85911880730259,-1.23430151390798,
-26.1566166953978));
#23889=CARTESIAN_POINT('Ctrl Pts',(-1.00482069987022,-1.11509090750047,
-26.1664954267595));
#23890=CARTESIAN_POINT('Ctrl Pts',(-1.05761684173333,-1.06506374863199,
-26.1702095722915));
#23891=CARTESIAN_POINT('Ctrl Pts',(-1.1844001976096,-0.926340335232992,
-26.1798111477295));
#23892=CARTESIAN_POINT('Ctrl Pts',(-1.25261441634892,-0.83211920082608,
-26.1857052765572));
#23893=CARTESIAN_POINT('Ctrl Pts',(-1.34074826464044,-0.674326760409325,
-26.1954147409246));
#23894=CARTESIAN_POINT('Ctrl Pts',(-1.36868794552701,-0.615585478595458,
-26.1989842830473));
#23895=CARTESIAN_POINT('Ctrl Pts',(-1.43485703413466,-0.449600827717206,
-26.2088401621456));
#23896=CARTESIAN_POINT('Ctrl Pts',(-1.46506530207602,-0.338953293629063,
-26.2151353002451));
#23897=CARTESIAN_POINT('Ctrl Pts',(-1.49307424044238,-0.15424442962602,
-26.2249405220094));
#23898=CARTESIAN_POINT('Ctrl Pts',(-1.49872145505749,-0.0819601957990811,
-26.2286437288062));
#23899=CARTESIAN_POINT('Ctrl Pts',(-1.4999128142802,0.10635364717765,-26.2382653050375));
#23900=CARTESIAN_POINT('Ctrl Pts',(-1.48729611729633,0.222621170813189,
-26.2441894727905));
#23901=CARTESIAN_POINT('Ctrl Pts',(-1.44664089724751,0.399454503995218,
-26.2539378222371));
#23902=CARTESIAN_POINT('Ctrl Pts',(-1.42792282839189,0.461843884428479,
-26.257512527193));
#23903=CARTESIAN_POINT('Ctrl Pts',(-1.36567226646368,0.629155145193409,
-26.267359150332));
#23904=CARTESIAN_POINT('Ctrl Pts',(-1.3139744789766,0.731242932312221,-26.2736393537179));
#23905=CARTESIAN_POINT('Ctrl Pts',(-1.2110594246586,0.886786659230229,-26.2834285909181));
#23906=CARTESIAN_POINT('Ctrl Pts',(-1.16680806056728,0.944158793526481,
-26.2871294400225));
#23907=CARTESIAN_POINT('Ctrl Pts',(-1.04136689066287,1.08472802366668,-26.2967553749447));
#23908=CARTESIAN_POINT('Ctrl Pts',(-0.953934620650422,1.16260491289205,
-26.3026860592708));
#23909=CARTESIAN_POINT('Ctrl Pts',(-0.805047877218473,1.26658368501614,
-26.312442864928));
#23910=CARTESIAN_POINT('Ctrl Pts',(-0.749301072162544,1.30031295894254,
-26.3160187086009));
#23911=CARTESIAN_POINT('Ctrl Pts',(-0.590941438505108,1.38263225313536,
-26.3258632125988));
#23912=CARTESIAN_POINT('Ctrl Pts',(-0.484180955146683,1.4236573787086,-26.3321400480036));
#23913=CARTESIAN_POINT('Ctrl Pts',(-0.303595410153914,1.46999439523184,
-26.3419255580418));
#23914=CARTESIAN_POINT('Ctrl Pts',(-0.232307353434979,1.4828716436308,-26.3456257619413));
#23915=CARTESIAN_POINT('Ctrl Pts',(-0.0449665451035471,1.50301868666175,
-26.3552526860981));
#23916=CARTESIAN_POINT('Ctrl Pts',(0.0721499053482647,1.50214624239001,
-26.3611849503045));
#23917=CARTESIAN_POINT('Ctrl Pts',(0.252356788815005,1.47940947106688,-26.3709436521134));
#23918=CARTESIAN_POINT('Ctrl Pts',(0.316329984727802,1.46703825681549,-26.3745196087977));
#23919=CARTESIAN_POINT('Ctrl Pts',(0.489002070828588,1.4218861436686,-26.3843641477804));
#23920=CARTESIAN_POINT('Ctrl Pts',(0.595703752241775,1.38071290442607,-26.390640884777));
#23921=CARTESIAN_POINT('Ctrl Pts',(0.760732886542325,1.29396300726967,-26.4004266802352));
#23922=CARTESIAN_POINT('Ctrl Pts',(0.822251899522651,1.25569822892507,-26.4041272317976));
#23923=CARTESIAN_POINT('Ctrl Pts',(0.974721464626966,1.14499111466233,-26.4137542763936));
#23924=CARTESIAN_POINT('Ctrl Pts',(1.06100126006438,1.06579775744788,-26.4196863404273));
#23925=CARTESIAN_POINT('Ctrl Pts',(1.17942115031437,0.928064769776612,-26.4294454073568));
#23926=CARTESIAN_POINT('Ctrl Pts',(1.21858093601503,0.875972882995377,-26.4330219823601));
#23927=CARTESIAN_POINT('Ctrl Pts',(1.31635792021209,0.7266895236537,-26.4428651778376));
#23928=CARTESIAN_POINT('Ctrl Pts',(1.3678726784997,0.624617905788714,-26.4491399085815));
#23929=CARTESIAN_POINT('Ctrl Pts',(1.43208829773097,0.449639147595743,-26.4589230349693));
#23930=CARTESIAN_POINT('Ctrl Pts',(1.4520550072253,0.380012749941871,-26.4626227873655));
#23931=CARTESIAN_POINT('Ctrl Pts',(1.49091078706645,0.195638319667655,-26.4722498568713));
#23932=CARTESIAN_POINT('Ctrl Pts',(1.50180158407935,0.0790135856532134,
-26.4781826846612));
#23933=CARTESIAN_POINT('Ctrl Pts',(1.49726914081623,-0.102565685129436,
-26.4879413830688));
#23934=CARTESIAN_POINT('Ctrl Pts',(1.49138397176759,-0.167445996749231,
-26.491516694186));
#23935=CARTESIAN_POINT('Ctrl Pts',(1.46380024372253,-0.343759005058039,
-26.5013601509739));
#23936=CARTESIAN_POINT('Ctrl Pts',(1.43355155078388,-0.454047762524838,
-26.5076365685205));
#23937=CARTESIAN_POINT('Ctrl Pts',(1.36383715846955,-0.626892751013256,
-26.517418935626));
#23938=CARTESIAN_POINT('Ctrl Pts',(1.33197267114545,-0.691893101510102,
-26.521116558156));
#23939=CARTESIAN_POINT('Ctrl Pts',(1.23713794533795,-0.854747866201789,
-26.5307449733761));
#23940=CARTESIAN_POINT('Ctrl Pts',(1.16695617220513,-0.948619287037085,
-26.5366810868746));
#23941=CARTESIAN_POINT('Ctrl Pts',(1.04176467010574,-1.08030294138717,-26.5464428691456));
#23942=CARTESIAN_POINT('Ctrl Pts',(0.993893811690886,-1.12446988675267,
-26.5500173855498));
#23943=CARTESIAN_POINT('Ctrl Pts',(0.854960109142449,-1.2369267158239,-26.5598766748324));
#23944=CARTESIAN_POINT('Ctrl Pts',(0.758281496474013,-1.2985779491472,-26.5661693590029));
#23945=CARTESIAN_POINT('Ctrl Pts',(0.589926831790066,-1.3802537244995,-26.5759907249344));
#23946=CARTESIAN_POINT('Ctrl Pts',(0.522253827245407,-1.40719254860585,
-26.5797110165672));
#23947=CARTESIAN_POINT('Ctrl Pts',(0.342772001528536,-1.46406858457962,
-26.5893325854756));
#23948=CARTESIAN_POINT('Ctrl Pts',(0.228359414155081,-1.48640798527583,
-26.5952410178224));
#23949=CARTESIAN_POINT('Ctrl Pts',(0.0473981458182217,-1.50005763135903,
-26.6049927328855));
#23950=CARTESIAN_POINT('Ctrl Pts',(-0.0181333502888847,-1.50067294465087,
-26.6085898216814));
#23951=CARTESIAN_POINT('Ctrl Pts',(-0.19496047411489,-1.49080744377269,
-26.6183572236448));
#23952=CARTESIAN_POINT('Ctrl Pts',(-0.305997694094707,-1.47214363262793,
-26.6245351400502));
#23953=CARTESIAN_POINT('Ctrl Pts',(-0.482045264444345,-1.42142967465588,
-26.6341515060131));
#23954=CARTESIAN_POINT('Ctrl Pts',(-0.548680651270178,-1.39699037194736,
-26.6377773152219));
#23955=CARTESIAN_POINT('Ctrl Pts',(-0.721057963265396,-1.31966544505203,
-26.647423289794));
#23956=CARTESIAN_POINT('Ctrl Pts',(-0.823339228634004,-1.25860902335675,
-26.6534426411113));
#23957=CARTESIAN_POINT('Ctrl Pts',(-0.967377496896887,-1.14725955151277,
-26.6632185228844));
#23958=CARTESIAN_POINT('Ctrl Pts',(-1.01512851775822,-1.10520351414327,
-26.6667090527507));
#23959=CARTESIAN_POINT('Ctrl Pts',(-1.12706752532266,-0.993292725067995,
-26.675443992847));
#23960=CARTESIAN_POINT('Ctrl Pts',(-1.18780019231101,-0.919909652198967,
-26.680705639719));
#23961=CARTESIAN_POINT('Ctrl Pts',(-1.29936775096139,-0.755307651316867,
-26.6913274460603));
#23962=CARTESIAN_POINT('Ctrl Pts',(-1.34865829060901,-0.663077553166124,
-26.6966469113585));
#23963=CARTESIAN_POINT('Ctrl Pts',(-1.40190296279248,-0.532756487150161,
-26.7038489235449));
#23964=CARTESIAN_POINT('Ctrl Pts',(-1.41456019814549,-0.498231485192453,
-26.7057295679761));
#23965=CARTESIAN_POINT('Ctrl Pts',(-1.42593782207381,-0.463290149673335,
-26.7076220835797));
#23966=CARTESIAN_POINT('',(-1.42616365839152,-0.463388665150944,-27.2075569156963));
#23967=CARTESIAN_POINT('Ctrl Pts',(-1.42590316226897,-0.46327735868407,
-26.7076008391022));
#23968=CARTESIAN_POINT('Ctrl Pts',(-1.48022542784997,-0.297586107654068,
-26.7167843685386));
#23969=CARTESIAN_POINT('Ctrl Pts',(-1.50486925637141,-0.125249205425268,
-26.7263745778538));
#23970=CARTESIAN_POINT('Ctrl Pts',(-1.49291374415963,0.209427358776284,
-26.7441959507517));
#23971=CARTESIAN_POINT('Ctrl Pts',(-1.46138855081052,0.368703742541458,
-26.7524076631357));
#23972=CARTESIAN_POINT('Ctrl Pts',(-1.37516087375663,0.603706007214842,
-26.7654670202156));
#23973=CARTESIAN_POINT('Ctrl Pts',(-1.33661136820521,0.68555664639347,-26.7702202361326));
#23974=CARTESIAN_POINT('Ctrl Pts',(-1.2448441354841,0.841472035895783,-26.7800100546894));
#23975=CARTESIAN_POINT('Ctrl Pts',(-1.1916507879262,0.915262310204792,-26.7850425184109));
#23976=CARTESIAN_POINT('Ctrl Pts',(-1.00987125882251,1.12359212643019,-26.7999793803873));
#23977=CARTESIAN_POINT('Ctrl Pts',(-0.86135529066732,1.24034483336812,-26.8094788432607));
#23978=CARTESIAN_POINT('Ctrl Pts',(-0.617304190663664,1.36916322477178,
-26.823865733921));
#23979=CARTESIAN_POINT('Ctrl Pts',(-0.533635780763124,1.40423385403138,
-26.8286254950898));
#23980=CARTESIAN_POINT('Ctrl Pts',(-0.359394154914502,1.45906580714,-26.8384961681381));
#23981=CARTESIAN_POINT('Ctrl Pts',(-0.268988163959942,1.47840340652547,
-26.8436062466654));
#23982=CARTESIAN_POINT('Ctrl Pts',(0.00732540329836662,1.5107086221588,
-26.8586170253155));
#23983=CARTESIAN_POINT('Ctrl Pts',(0.195979873932844,1.49733320545277,-26.8681241570776));
#23984=CARTESIAN_POINT('Ctrl Pts',(0.463267412983477,1.42864141281074,-26.8825180045602));
#23985=CARTESIAN_POINT('Ctrl Pts',(0.548609796066798,1.39844020086262,-26.8872712335173));
#23986=CARTESIAN_POINT('Ctrl Pts',(0.714355014249309,1.32201980761357,-26.8971412079893));
#23987=CARTESIAN_POINT('Ctrl Pts',(0.794334488308791,1.27556785177849,-26.9022544655732));
#23988=CARTESIAN_POINT('Ctrl Pts',(1.02067770564489,1.11375913918672,-26.9172619308146));
#23989=CARTESIAN_POINT('Ctrl Pts',(1.15135498077534,0.977128794457907,-26.9267635866013));
#23990=CARTESIAN_POINT('Ctrl Pts',(1.32471965108333,0.713890117675608,-26.9432059032433));
#23991=CARTESIAN_POINT('Ctrl Pts',(1.38204127770906,0.596833407966587,-26.9501142277202));
#23992=CARTESIAN_POINT('Ctrl Pts',(1.46873900176316,0.336259442922926,-26.9651555553315));
#23993=CARTESIAN_POINT('Ctrl Pts',(1.49355317711586,0.193731144783341,-26.9728184717108));
#23994=CARTESIAN_POINT('Ctrl Pts',(1.50400111145276,-0.134796170383052,
-26.9899382087099));
#23995=CARTESIAN_POINT('Ctrl Pts',(1.47619648535756,-0.321142588299731,
-26.9994252155968));
#23996=CARTESIAN_POINT('Ctrl Pts',(1.38706298095157,-0.576977166917857,
-27.0140901232008));
#23997=CARTESIAN_POINT('Ctrl Pts',(1.35176410527077,-0.655426009430809,
-27.0188416980206));
#23998=CARTESIAN_POINT('Ctrl Pts',(1.26341901571074,-0.813160526073467,
-27.0286181558124));
#23999=CARTESIAN_POINT('Ctrl Pts',(1.20901892461933,-0.891452413251942,
-27.0336144797392));
#24000=CARTESIAN_POINT('Ctrl Pts',(1.0284633921148,-1.10565620989746,-27.0482109139249));
#24001=CARTESIAN_POINT('Ctrl Pts',(0.883116781281584,-1.22570860803761,
-27.0576996903132));
#24002=CARTESIAN_POINT('Ctrl Pts',(0.644888168564368,-1.35688218325702,
-27.0724070805618));
#24003=CARTESIAN_POINT('Ctrl Pts',(0.565309749810226,-1.39191973600915,
-27.0772093561898));
#24004=CARTESIAN_POINT('Ctrl Pts',(0.341617477538992,-1.4675852545328,-27.0899790753639));
#24005=CARTESIAN_POINT('Ctrl Pts',(0.192800060504756,-1.4938398680087,-27.0977154107084));
#24006=CARTESIAN_POINT('Ctrl Pts',(-0.10177151207912,-1.50249575613366,
-27.1130005942386));
#24007=CARTESIAN_POINT('Ctrl Pts',(-0.247967527283484,-1.48610526266758,
-27.1205961668103));
#24008=CARTESIAN_POINT('Ctrl Pts',(-0.499452916756478,-1.41887331687768,
-27.1347845490264));
#24009=CARTESIAN_POINT('Ctrl Pts',(-0.605605262643713,-1.37672641961951,
-27.1410472347818));
#24010=CARTESIAN_POINT('Ctrl Pts',(-0.809424221127998,-1.26706377776192,
-27.1533216201516));
#24011=CARTESIAN_POINT('Ctrl Pts',(-0.905761853669422,-1.19975808356791,
-27.1593547939893));
#24012=CARTESIAN_POINT('Ctrl Pts',(-1.09031963371981,-1.0367207065882,-27.1721305544943));
#24013=CARTESIAN_POINT('Ctrl Pts',(-1.17668388134904,-0.938483389056613,
-27.178901138905));
#24014=CARTESIAN_POINT('Ctrl Pts',(-1.32462526276729,-0.716823167178535,
-27.193351009864));
#24015=CARTESIAN_POINT('Ctrl Pts',(-1.38389132700062,-0.593751662693113,
-27.2008076632993));
#24016=CARTESIAN_POINT('Ctrl Pts',(-1.42588748976423,-0.463325593694253,
-27.2080241608977));
#24017=CARTESIAN_POINT('',(-1.109870874299,-0.360618907335,-27.01554752692));
#24018=CARTESIAN_POINT('Ctrl Pts',(0.2686738342207,1.511381850733,-24.85156091023));
#24019=CARTESIAN_POINT('Ctrl Pts',(0.6390292315051,1.445544878716,-24.87106091023));
#24020=CARTESIAN_POINT('Ctrl Pts',(1.326904859784,1.029536455846,-24.91006091023));
#24021=CARTESIAN_POINT('Ctrl Pts',(1.674980827552,-0.126538586479,-24.96856091023));
#24022=CARTESIAN_POINT('Ctrl Pts',(1.157464687037,-1.217176691488,-25.02706091023));
#24023=CARTESIAN_POINT('Ctrl Pts',(0.0422160704956,-1.679143820308,-25.08556091023));
#24024=CARTESIAN_POINT('Ctrl Pts',(-1.094869212689,-1.273799959595,-25.14406091023));
#24025=CARTESIAN_POINT('Ctrl Pts',(-1.666428125978,-0.2105189542896,-25.20256091023));
#24026=CARTESIAN_POINT('Ctrl Pts',(-1.377251744299,0.9614989552941,-25.26106091023));
#24027=CARTESIAN_POINT('Ctrl Pts',(-0.3767015711466,1.636886726176,-25.31956091023));
#24028=CARTESIAN_POINT('Ctrl Pts',(0.818421000234,1.466795597545,-25.37806091023));
#24029=CARTESIAN_POINT('Ctrl Pts',(1.590815701598,0.5390803996589,-25.43656091023));
#24030=CARTESIAN_POINT('Ctrl Pts',(1.541527905363,-0.6670786928981,-25.49506091023));
#24031=CARTESIAN_POINT('Ctrl Pts',(0.6960155840139,-1.528680664665,-25.55356091023));
#24032=CARTESIAN_POINT('Ctrl Pts',(-0.5090002399164,-1.600693919274,-25.61206091023));
#24033=CARTESIAN_POINT('Ctrl Pts',(-1.451109064351,-0.8459224259632,-25.67056091023));
#24034=CARTESIAN_POINT('Ctrl Pts',(-1.643696179801,0.3457819196178,-25.72906091023));
#24035=CARTESIAN_POINT('Ctrl Pts',(-0.9872871721321,1.358884214036,-25.78756091023));
#24036=CARTESIAN_POINT('Ctrl Pts',(0.179071905278,1.670100452118,-25.84606091023));
#24037=CARTESIAN_POINT('Ctrl Pts',(1.252937397068,1.11868232596,-25.90456091023));
#24038=CARTESIAN_POINT('Ctrl Pts',(1.679640106794,-0.0105536288799,-25.96306091023));
#24039=CARTESIAN_POINT('Ctrl Pts',(1.238781063654,-1.134338460973,-26.02156091023));
#24040=CARTESIAN_POINT('Ctrl Pts',(0.1580712177019,-1.672218812138,-26.08006091023));
#24041=CARTESIAN_POINT('Ctrl Pts',(-1.004285013615,-1.3463706344,-26.13856091023));
#24042=CARTESIAN_POINT('Ctrl Pts',(-1.647911508744,-0.3250998584294,-26.19706091023));
#24043=CARTESIAN_POINT('Ctrl Pts',(-1.440364600074,0.8640903001927,-26.25556091023));
#24044=CARTESIAN_POINT('Ctrl Pts',(-0.4888456523225,1.606963763254,-26.31406091023));
#24045=CARTESIAN_POINT('Ctrl Pts',(0.7151700341124,1.519813393635,-26.37256091023));
#24046=CARTESIAN_POINT('Ctrl Pts',(1.549788945368,0.6476566642697,-26.43106091023));
#24047=CARTESIAN_POINT('Ctrl Pts',(1.583915188882,-0.559033845412,-26.48956091023));
#24048=CARTESIAN_POINT('Ctrl Pts',(0.7999275652393,-1.476942615815,-26.54806091023));
#24049=CARTESIAN_POINT('Ctrl Pts',(-0.3972521937322,-1.632104004379,-26.60656091023));
#24050=CARTESIAN_POINT('Ctrl Pts',(-1.389183506688,-0.9438172522165,-26.66506091023));
#24051=CARTESIAN_POINT('Ctrl Pts',(-1.572265768938,-0.161054981071,-26.70406091023));
#24052=CARTESIAN_POINT('Ctrl Pts',(-1.520434338468,0.2115186760726,-26.72356091023));
#24053=CARTESIAN_POINT('Ctrl Pts',(0.2451527031279,1.379067475031,-24.92915029444));
#24054=CARTESIAN_POINT('Ctrl Pts',(0.5830852265001,1.318994220401,-24.94865029444));
#24055=CARTESIAN_POINT('Ctrl Pts',(1.210740577374,0.9394053792083,-24.98765029444));
#24056=CARTESIAN_POINT('Ctrl Pts',(1.528344130543,-0.1154607281177,-25.04615029444));
#24057=CARTESIAN_POINT('Ctrl Pts',(1.056134095176,-1.110618594357,-25.10465029444));
#24058=CARTESIAN_POINT('Ctrl Pts',(0.0385202519905,-1.532142672854,-25.16315029444));
#24059=CARTESIAN_POINT('Ctrl Pts',(-0.9990185603326,-1.162284761539,-25.22165029444));
#24060=CARTESIAN_POINT('Ctrl Pts',(-1.520540177784,-0.1920890095362,-25.28015029444));
#24061=CARTESIAN_POINT('Ctrl Pts',(-1.256679828841,0.8773242419706,-25.33865029444));
#24062=CARTESIAN_POINT('Ctrl Pts',(-0.3437231195475,1.493584988654,-25.39715029444));
#24063=CARTESIAN_POINT('Ctrl Pts',(0.7467720892358,1.3383845387,-25.45565029444));
#24064=CARTESIAN_POINT('Ctrl Pts',(1.451547265688,0.4918864450011,-25.51415029444));
#24065=CARTESIAN_POINT('Ctrl Pts',(1.406574384301,-0.6086790894146,-25.57265029444));
#24066=CARTESIAN_POINT('Ctrl Pts',(0.6350826917518,-1.394851859129,-25.63115029444));
#24067=CARTESIAN_POINT('Ctrl Pts',(-0.4644396618308,-1.460560691846,-25.68965029444));
#24068=CARTESIAN_POINT('Ctrl Pts',(-1.324071287741,-0.7718658944325,-25.74815029444));
#24069=CARTESIAN_POINT('Ctrl Pts',(-1.499798306627,0.3155103381501,-25.80665029444));
#24070=CARTESIAN_POINT('Ctrl Pts',(-0.9008548216604,1.239920289503,-25.86515029444));
#24071=CARTESIAN_POINT('Ctrl Pts',(0.1633950018263,1.523891009035,-25.92365029444));
#24072=CARTESIAN_POINT('Ctrl Pts',(1.143248618282,1.020746947487,-25.98215029444));
#24073=CARTESIAN_POINT('Ctrl Pts',(1.532595511792,-0.00962970828634,-26.04065029444));
#24074=CARTESIAN_POINT('Ctrl Pts',(1.130331605306,-1.035032461483,-26.09915029444));
#24075=CARTESIAN_POINT('Ctrl Pts',(0.1442328257187,-1.525823916594,-26.15765029444));
#24076=CARTESIAN_POINT('Ctrl Pts',(-0.9163645820317,-1.228502214935,-26.21615029444));
#24077=CARTESIAN_POINT('Ctrl Pts',(-1.503644603339,-0.296638894188,-26.27465029444));
#24078=CARTESIAN_POINT('Ctrl Pts',(-1.3142674508,0.7884432566844,-26.33315029444));
#24079=CARTESIAN_POINT('Ctrl Pts',(-0.4460495136298,1.466281640462,-26.39165029444));
#24080=CARTESIAN_POINT('Ctrl Pts',(0.6525602597933,1.386760875991,-26.45015029444));
#24081=CARTESIAN_POINT('Ctrl Pts',(1.414112209091,0.5909573680856,-26.50865029444));
#24082=CARTESIAN_POINT('Ctrl Pts',(1.445250860419,-0.510093060384,-26.56715029444));
#24083=CARTESIAN_POINT('Ctrl Pts',(0.7298976675334,-1.347643233224,-26.62565029444));
#24084=CARTESIAN_POINT('Ctrl Pts',(-0.3624746317386,-1.489220971666,-26.68415029444));
#24085=CARTESIAN_POINT('Ctrl Pts',(-1.267567021527,-0.8611904888719,-26.74265029444));
#24086=CARTESIAN_POINT('Ctrl Pts',(-1.434621292425,-0.1469553746322,-26.78165029444));
#24087=CARTESIAN_POINT('Ctrl Pts',(-1.387327460022,0.193001210377,-26.80115029444));
#24088=CARTESIAN_POINT('Ctrl Pts',(0.2216315720351,1.246753099329,-25.00673967864));
#24089=CARTESIAN_POINT('Ctrl Pts',(0.527141221495,1.192443562085,-25.02623967864));
#24090=CARTESIAN_POINT('Ctrl Pts',(1.094576294964,0.8492743025702,-25.06523967864));
#24091=CARTESIAN_POINT('Ctrl Pts',(1.381707433535,-0.1043828697565,-25.12373967864));
#24092=CARTESIAN_POINT('Ctrl Pts',(0.9548035033152,-1.004060497225,-25.18223967864));
#24093=CARTESIAN_POINT('Ctrl Pts',(0.0348244334854,-1.385141525401,-25.24073967864));
#24094=CARTESIAN_POINT('Ctrl Pts',(-0.9031679079763,-1.050769563483,-25.29923967864));
#24095=CARTESIAN_POINT('Ctrl Pts',(-1.37465222959,-0.1736590647829,-25.35773967864));
#24096=CARTESIAN_POINT('Ctrl Pts',(-1.136107913383,0.793149528647,-25.41623967864));
#24097=CARTESIAN_POINT('Ctrl Pts',(-0.3107446679484,1.350283251132,-25.47473967864));
#24098=CARTESIAN_POINT('Ctrl Pts',(0.6751231782377,1.209973479856,-25.53323967864));
#24099=CARTESIAN_POINT('Ctrl Pts',(1.312278829779,0.4446924903434,-25.59173967864));
#24100=CARTESIAN_POINT('Ctrl Pts',(1.27162086324,-0.5502794859312,-25.65023967864));
#24101=CARTESIAN_POINT('Ctrl Pts',(0.5741497994896,-1.261023053592,-25.70873967864));
#24102=CARTESIAN_POINT('Ctrl Pts',(-0.4198790837452,-1.320427464418,-25.76723967864));
#24103=CARTESIAN_POINT('Ctrl Pts',(-1.197033511132,-0.6978093629019,-25.82573967864));
#24104=CARTESIAN_POINT('Ctrl Pts',(-1.355900433453,0.2852387566824,-25.88423967864));
#24105=CARTESIAN_POINT('Ctrl Pts',(-0.8144224711886,1.120956364969,-25.94273967864));
#24106=CARTESIAN_POINT('Ctrl Pts',(0.1477180983746,1.377681565952,-26.00123967864));
#24107=CARTESIAN_POINT('Ctrl Pts',(1.033559839496,0.9228115690148,-26.05973967864));
#24108=CARTESIAN_POINT('Ctrl Pts',(1.38555091679,-0.008705787692769,-26.11823967864));
#24109=CARTESIAN_POINT('Ctrl Pts',(1.021882146958,-0.9357264619928,-26.17673967864));
#24110=CARTESIAN_POINT('Ctrl Pts',(0.1303944337356,-1.37942902105,-26.23523967864));
#24111=CARTESIAN_POINT('Ctrl Pts',(-0.8284441504486,-1.11063379547,-26.29373967864));
#24112=CARTESIAN_POINT('Ctrl Pts',(-1.359377697933,-0.2681779299465,-26.35223967864));
#24113=CARTESIAN_POINT('Ctrl Pts',(-1.188170301526,0.712796213176,-26.41073967864));
#24114=CARTESIAN_POINT('Ctrl Pts',(-0.403253374937,1.32559951767,-26.46923967864));
#24115=CARTESIAN_POINT('Ctrl Pts',(0.5899504854742,1.253708358346,-26.52773967864));
#24116=CARTESIAN_POINT('Ctrl Pts',(1.278435472814,0.5342580719014,-26.58623967864));
#24117=CARTESIAN_POINT('Ctrl Pts',(1.306586531957,-0.461152275356,-26.64473967864));
#24118=CARTESIAN_POINT('Ctrl Pts',(0.6598677698274,-1.218343850632,-26.70323967864));
#24119=CARTESIAN_POINT('Ctrl Pts',(-0.3276970697449,-1.346337938953,-26.76173967864));
#24120=CARTESIAN_POINT('Ctrl Pts',(-1.145950536365,-0.7785637255274,-26.82023967864));
#24121=CARTESIAN_POINT('Ctrl Pts',(-1.296976815913,-0.1328557681934,-26.85923967864));
#24122=CARTESIAN_POINT('Ctrl Pts',(-1.254220581577,0.1744837446815,-26.87873967864));
#24123=CARTESIAN_POINT('Ctrl Pts',(0.1981104409423,1.114438723627,-25.08432906285));
#24124=CARTESIAN_POINT('Ctrl Pts',(0.47119721649,1.065892903769,-25.10382906285));
#24125=CARTESIAN_POINT('Ctrl Pts',(0.9784120125535,0.7591432259322,-25.14282906285));
#24126=CARTESIAN_POINT('Ctrl Pts',(1.235070736526,-0.09330501139523,-25.20132906285));
#24127=CARTESIAN_POINT('Ctrl Pts',(0.8534729114545,-0.8975024000936,-25.25982906285));
#24128=CARTESIAN_POINT('Ctrl Pts',(0.03112861498029,-1.238140377948,-25.31832906285));
#24129=CARTESIAN_POINT('Ctrl Pts',(-0.80731725562,-0.9392543654266,-25.37682906285));
#24130=CARTESIAN_POINT('Ctrl Pts',(-1.228764281396,-0.1552291200295,-25.43532906285));
#24131=CARTESIAN_POINT('Ctrl Pts',(-1.015535997925,0.7089748153235,-25.49382906285));
#24132=CARTESIAN_POINT('Ctrl Pts',(-0.2777662163492,1.206981513611,-25.55232906285));
#24133=CARTESIAN_POINT('Ctrl Pts',(0.6034742672396,1.081562421011,-25.61082906285));
#24134=CARTESIAN_POINT('Ctrl Pts',(1.173010393869,0.3974985356856,-25.66932906285));
#24135=CARTESIAN_POINT('Ctrl Pts',(1.136667342178,-0.4918798824477,-25.72782906285));
#24136=CARTESIAN_POINT('Ctrl Pts',(0.5132169072275,-1.127194248056,-25.78632906285));
#24137=CARTESIAN_POINT('Ctrl Pts',(-0.3753185056597,-1.180294236991,-25.84482906285));
#24138=CARTESIAN_POINT('Ctrl Pts',(-1.069995734522,-0.6237528313713,-25.90332906285));
#24139=CARTESIAN_POINT('Ctrl Pts',(-1.212002560279,0.2549671752147,-25.96182906285));
#24140=CARTESIAN_POINT('Ctrl Pts',(-0.7279901207168,1.001992440436,-26.02032906285));
#24141=CARTESIAN_POINT('Ctrl Pts',(0.1320411949229,1.231472122869,-26.07882906285));
#24142=CARTESIAN_POINT('Ctrl Pts',(0.9238710607092,0.8248761905421,-26.13732906285));
#24143=CARTESIAN_POINT('Ctrl Pts',(1.238506321788,-0.007781867099204,-26.19582906285));
#24144=CARTESIAN_POINT('Ctrl Pts',(0.9134326886102,-0.8364204625026,-26.25432906285));
#24145=CARTESIAN_POINT('Ctrl Pts',(0.1165560417524,-1.233034125506,-26.31282906285));
#24146=CARTESIAN_POINT('Ctrl Pts',(-0.7405237188655,-0.992765376005,-26.37132906285));
#24147=CARTESIAN_POINT('Ctrl Pts',(-1.215110792527,-0.2397169657051,-26.42982906285));
#24148=CARTESIAN_POINT('Ctrl Pts',(-1.062073152252,0.6371491696676,-26.48832906285));
#24149=CARTESIAN_POINT('Ctrl Pts',(-0.3604572362442,1.184917394878,-26.54682906285));
#24150=CARTESIAN_POINT('Ctrl Pts',(0.5273407111551,1.120655840702,-26.60532906285));
#24151=CARTESIAN_POINT('Ctrl Pts',(1.142758736536,0.4775587757172,-26.66382906285));
#24152=CARTESIAN_POINT('Ctrl Pts',(1.167922203495,-0.412211490328,-26.72232906285));
#24153=CARTESIAN_POINT('Ctrl Pts',(0.5898378721215,-1.089044468041,-26.78082906285));
#24154=CARTESIAN_POINT('Ctrl Pts',(-0.2929195077513,-1.20345490624,-26.83932906285));
#24155=CARTESIAN_POINT('Ctrl Pts',(-1.024334051204,-0.6959369621828,-26.89782906285));
#24156=CARTESIAN_POINT('Ctrl Pts',(-1.1593323394,-0.1187561617546,-26.93682906285));
#24157=CARTESIAN_POINT('Ctrl Pts',(-1.121113703131,0.1559662789859,-26.95632906285));
#24158=CARTESIAN_POINT('',(-1.426584774443,-0.4635254915624,-26.7078125));
#24159=CARTESIAN_POINT('Ctrl Pts',(-1.105729660272,-1.064811084801,-26.65156091023));
#24160=CARTESIAN_POINT('Ctrl Pts',(-1.366655469426,-0.7938584149506,-26.67106091023));
#24161=CARTESIAN_POINT('Ctrl Pts',(-1.678634926928,-0.05297738133179,-26.71006091023));
#24162=CARTESIAN_POINT('Ctrl Pts',(-1.280710439764,1.086900895213,-26.76856091023));
#24163=CARTESIAN_POINT('Ctrl Pts',(-0.2209700935106,1.665057301661,-26.82706091023));
#24164=CARTESIAN_POINT('Ctrl Pts',(0.9528224555883,1.383269870276,-26.88556091023));
#24165=CARTESIAN_POINT('Ctrl Pts',(1.634488630304,0.386977838339,-26.94406091023));
#24166=CARTESIAN_POINT('Ctrl Pts',(1.47190861048,-0.809188464797,-27.00256091023));
#24167=CARTESIAN_POINT('Ctrl Pts',(0.549065160654,-1.5873972589,-27.06106091023));
#24168=CARTESIAN_POINT('Ctrl Pts',(-0.657379904454,-1.545688807378,-27.11956091023));
#24169=CARTESIAN_POINT('Ctrl Pts',(-1.524277318107,-0.7056067715846,-27.17806091023));
#24170=CARTESIAN_POINT('Ctrl Pts',(-1.603860446231,0.4989328038561,-27.23656091023));
#24171=CARTESIAN_POINT('Ctrl Pts',(-0.8550232549381,1.44576536791,-27.29506091023));
#24172=CARTESIAN_POINT('Ctrl Pts',(0.3354475143376,1.645836332335,-27.35356091023));
#24173=CARTESIAN_POINT('Ctrl Pts',(1.352654123417,0.9958057490488,-27.41206091023));
#24174=CARTESIAN_POINT('Ctrl Pts',(1.671192620316,-0.1685748889662,-27.47056091023));
#24175=CARTESIAN_POINT('Ctrl Pts',(1.126532630187,-1.245883823055,-27.52906091023));
#24176=CARTESIAN_POINT('Ctrl Pts',(0.,-1.6796732621,-27.58756091023));
#24177=CARTESIAN_POINT('Ctrl Pts',(-1.126532630187,-1.245883823055,-27.64606091023));
#24178=CARTESIAN_POINT('Ctrl Pts',(-1.671192620316,-0.1685748889661,-27.70456091023));
#24179=CARTESIAN_POINT('Ctrl Pts',(-1.352654123417,0.9958057490488,-27.76306091023));
#24180=CARTESIAN_POINT('Ctrl Pts',(-0.3354475143376,1.645836332335,-27.82156091023));
#24181=CARTESIAN_POINT('Ctrl Pts',(0.8550232549381,1.44576536791,-27.88006091023));
#24182=CARTESIAN_POINT('Ctrl Pts',(1.603860446231,0.4989328038561,-27.93856091023));
#24183=CARTESIAN_POINT('Ctrl Pts',(1.524277318107,-0.7056067715846,-27.99706091023));
#24184=CARTESIAN_POINT('Ctrl Pts',(0.657379904454,-1.545688807378,-28.05556091023));
#24185=CARTESIAN_POINT('Ctrl Pts',(-0.549065160654,-1.5873972589,-28.11406091023));
#24186=CARTESIAN_POINT('Ctrl Pts',(-1.47190861048,-0.809188464797,-28.17256091023));
#24187=CARTESIAN_POINT('Ctrl Pts',(-1.634488630304,0.3869778383391,-28.23106091023));
#24188=CARTESIAN_POINT('Ctrl Pts',(-0.9528224555883,1.383269870276,-28.28956091023));
#24189=CARTESIAN_POINT('Ctrl Pts',(0.2209700935106,1.665057301661,-28.34806091023));
#24190=CARTESIAN_POINT('Ctrl Pts',(1.280710439764,1.086900895213,-28.40656091023));
#24191=CARTESIAN_POINT('Ctrl Pts',(1.678634926928,-0.05297738133181,-28.46506091023));
#24192=CARTESIAN_POINT('Ctrl Pts',(1.366655469426,-0.7938584149506,-28.50406091023));
#24193=CARTESIAN_POINT('Ctrl Pts',(1.105729660272,-1.064811084801,-28.52356091023));
#24194=CARTESIAN_POINT('Ctrl Pts',(-1.008928226787,-0.9715918802313,-26.72915029444));
#24195=CARTESIAN_POINT('Ctrl Pts',(-1.247011208018,-0.7243598428201,-26.74865029444));
#24196=CARTESIAN_POINT('Ctrl Pts',(-1.531678330698,-0.0483394606542,-26.78765029444));
#24197=CARTESIAN_POINT('Ctrl Pts',(-1.168590261656,0.9917478315913,-26.84615029444));
#24198=CARTESIAN_POINT('Ctrl Pts',(-0.2016252006515,1.519289362691,-26.90465029444));
#24199=CARTESIAN_POINT('Ctrl Pts',(0.8694073290239,1.262171096181,-26.96315029444));
#24200=CARTESIAN_POINT('Ctrl Pts',(1.491396834802,0.3530997478581,-27.02165029444));
#24201=CARTESIAN_POINT('Ctrl Pts',(1.34304993139,-0.7383478188722,-27.08015029444));
#24202=CARTESIAN_POINT('Ctrl Pts',(0.5009970871116,-1.448428091577,-27.13865029444));
#24203=CARTESIAN_POINT('Ctrl Pts',(-0.5998293843028,-1.410371018906,-27.19715029444));
#24204=CARTESIAN_POINT('Ctrl Pts',(-1.390834004861,-0.6438342159409,-27.25565029444));
#24205=CARTESIAN_POINT('Ctrl Pts',(-1.463450004255,0.4552535824685,-27.31415029444));
#24206=CARTESIAN_POINT('Ctrl Pts',(-0.7801699886157,1.319195406802,-27.37265029444));
#24207=CARTESIAN_POINT('Ctrl Pts',(0.3060806614679,1.501751098868,-27.43115029444));
#24208=CARTESIAN_POINT('Ctrl Pts',(1.234235614028,0.9086276372156,-27.48965029444));
#24209=CARTESIAN_POINT('Ctrl Pts',(1.524887563041,-0.1538169499438,-27.54815029444));
#24210=CARTESIAN_POINT('Ctrl Pts',(1.027909994485,-1.136812551513,-27.60665029444));
#24211=CARTESIAN_POINT('Ctrl Pts',(0.,-1.532625764506,-27.66515029444));
#24212=CARTESIAN_POINT('Ctrl Pts',(-1.027909994485,-1.136812551513,-27.72365029444));
#24213=CARTESIAN_POINT('Ctrl Pts',(-1.524887563041,-0.1538169499438,-27.78215029444));
#24214=CARTESIAN_POINT('Ctrl Pts',(-1.234235614028,0.9086276372156,-27.84065029444));
#24215=CARTESIAN_POINT('Ctrl Pts',(-0.3060806614679,1.501751098868,-27.89915029444));
#24216=CARTESIAN_POINT('Ctrl Pts',(0.7801699886157,1.319195406802,-27.95765029444));
#24217=CARTESIAN_POINT('Ctrl Pts',(1.463450004255,0.4552535824684,-28.01615029444));
#24218=CARTESIAN_POINT('Ctrl Pts',(1.390834004861,-0.6438342159409,-28.07465029444));
#24219=CARTESIAN_POINT('Ctrl Pts',(0.5998293843027,-1.410371018906,-28.13315029444));
#24220=CARTESIAN_POINT('Ctrl Pts',(-0.5009970871116,-1.448428091577,-28.19165029444));
#24221=CARTESIAN_POINT('Ctrl Pts',(-1.34304993139,-0.7383478188722,-28.25015029444));
#24222=CARTESIAN_POINT('Ctrl Pts',(-1.491396834802,0.3530997478581,-28.30865029444));
#24223=CARTESIAN_POINT('Ctrl Pts',(-0.8694073290239,1.262171096181,-28.36715029444));
#24224=CARTESIAN_POINT('Ctrl Pts',(0.2016252006515,1.519289362691,-28.42565029444));
#24225=CARTESIAN_POINT('Ctrl Pts',(1.168590261656,0.9917478315913,-28.48415029444));
#24226=CARTESIAN_POINT('Ctrl Pts',(1.531678330698,-0.04833946065422,-28.54265029444));
#24227=CARTESIAN_POINT('Ctrl Pts',(1.247011208018,-0.7243598428201,-28.58165029444));
#24228=CARTESIAN_POINT('Ctrl Pts',(1.008928226787,-0.9715918802313,-28.60115029444));
#24229=CARTESIAN_POINT('Ctrl Pts',(-0.9121267933018,-0.8783726756619,-26.80673967864));
#24230=CARTESIAN_POINT('Ctrl Pts',(-1.12736694661,-0.6548612706895,-26.82623967864));
#24231=CARTESIAN_POINT('Ctrl Pts',(-1.384721734467,-0.04370153997662,-26.86523967864));
#24232=CARTESIAN_POINT('Ctrl Pts',(-1.056470083549,0.8965947679692,-26.92373967864));
#24233=CARTESIAN_POINT('Ctrl Pts',(-0.1822803077923,1.373521423722,-26.98223967864));
#24234=CARTESIAN_POINT('Ctrl Pts',(0.7859922024595,1.141072322086,-27.04073967864));
#24235=CARTESIAN_POINT('Ctrl Pts',(1.3483050393,0.3192216573772,-27.09923967864));
#24236=CARTESIAN_POINT('Ctrl Pts',(1.2141912523,-0.6675071729475,-27.15773967864));
#24237=CARTESIAN_POINT('Ctrl Pts',(0.4529290135692,-1.309458924255,-27.21623967864));
#24238=CARTESIAN_POINT('Ctrl Pts',(-0.5422788641515,-1.275053230434,-27.27473967864));
#24239=CARTESIAN_POINT('Ctrl Pts',(-1.257390691615,-0.5820616602972,-27.33323967864));
#24240=CARTESIAN_POINT('Ctrl Pts',(-1.323039562278,0.4115743610808,-27.39173967864));
#24241=CARTESIAN_POINT('Ctrl Pts',(-0.7053167222932,1.192625445694,-27.45023967864));
#24242=CARTESIAN_POINT('Ctrl Pts',(0.2767138085983,1.357665865401,-27.50873967864));
#24243=CARTESIAN_POINT('Ctrl Pts',(1.11581710464,0.8214495253824,-27.56723967864));
#24244=CARTESIAN_POINT('Ctrl Pts',(1.378582505767,-0.1390590109215,-27.62573967864));
#24245=CARTESIAN_POINT('Ctrl Pts',(0.9292873587837,-1.027741279971,-27.68423967864));
#24246=CARTESIAN_POINT('Ctrl Pts',(0.,-1.385578266913,-27.74273967864));
#24247=CARTESIAN_POINT('Ctrl Pts',(-0.9292873587837,-1.027741279971,-27.80123967864));
#24248=CARTESIAN_POINT('Ctrl Pts',(-1.378582505767,-0.1390590109214,-27.85973967864));
#24249=CARTESIAN_POINT('Ctrl Pts',(-1.11581710464,0.8214495253824,-27.91823967864));
#24250=CARTESIAN_POINT('Ctrl Pts',(-0.2767138085983,1.357665865401,-27.97673967864));
#24251=CARTESIAN_POINT('Ctrl Pts',(0.7053167222932,1.192625445694,-28.03523967864));
#24252=CARTESIAN_POINT('Ctrl Pts',(1.323039562278,0.4115743610808,-28.09373967864));
#24253=CARTESIAN_POINT('Ctrl Pts',(1.257390691615,-0.5820616602972,-28.15223967864));
#24254=CARTESIAN_POINT('Ctrl Pts',(0.5422788641515,-1.275053230434,-28.21073967864));
#24255=CARTESIAN_POINT('Ctrl Pts',(-0.4529290135692,-1.309458924255,-28.26923967864));
#24256=CARTESIAN_POINT('Ctrl Pts',(-1.2141912523,-0.6675071729475,-28.32773967864));
#24257=CARTESIAN_POINT('Ctrl Pts',(-1.3483050393,0.3192216573772,-28.38623967864));
#24258=CARTESIAN_POINT('Ctrl Pts',(-0.7859922024595,1.141072322086,-28.44473967864));
#24259=CARTESIAN_POINT('Ctrl Pts',(0.1822803077923,1.373521423722,-28.50323967864));
#24260=CARTESIAN_POINT('Ctrl Pts',(1.056470083549,0.8965947679692,-28.56173967864));
#24261=CARTESIAN_POINT('Ctrl Pts',(1.384721734467,-0.04370153997664,-28.62023967864));
#24262=CARTESIAN_POINT('Ctrl Pts',(1.12736694661,-0.6548612706895,-28.65923967864));
#24263=CARTESIAN_POINT('Ctrl Pts',(0.9121267933018,-0.8783726756619,-28.67873967864));
#24264=CARTESIAN_POINT('Ctrl Pts',(-0.8153253598169,-0.7851534710925,-26.88432906285));
#24265=CARTESIAN_POINT('Ctrl Pts',(-1.007722685201,-0.585362698559,-26.90382906285));
#24266=CARTESIAN_POINT('Ctrl Pts',(-1.237765138237,-0.03906361929903,-26.94282906285));
#24267=CARTESIAN_POINT('Ctrl Pts',(-0.9443499054416,0.8014417043471,-27.00132906285));
#24268=CARTESIAN_POINT('Ctrl Pts',(-0.1629354149332,1.227753484752,-27.05982906285));
#24269=CARTESIAN_POINT('Ctrl Pts',(0.7025770758952,1.019973547991,-27.11832906285));
#24270=CARTESIAN_POINT('Ctrl Pts',(1.205213243798,0.2853435668963,-27.17682906285));
#24271=CARTESIAN_POINT('Ctrl Pts',(1.08533257321,-0.5966665270227,-27.23532906285));
#24272=CARTESIAN_POINT('Ctrl Pts',(0.4048609400268,-1.170489756933,-27.29382906285));
#24273=CARTESIAN_POINT('Ctrl Pts',(-0.4847283440002,-1.139735441963,-27.35232906285));
#24274=CARTESIAN_POINT('Ctrl Pts',(-1.123947378369,-0.5202891046535,-27.41082906285));
#24275=CARTESIAN_POINT('Ctrl Pts',(-1.182629120302,0.3678951396931,-27.46932906285));
#24276=CARTESIAN_POINT('Ctrl Pts',(-0.6304634559708,1.066055484586,-27.52782906285));
#24277=CARTESIAN_POINT('Ctrl Pts',(0.2473469557286,1.213580631934,-27.58632906285));
#24278=CARTESIAN_POINT('Ctrl Pts',(0.9973985952512,0.7342714135492,-27.64482906285));
#24279=CARTESIAN_POINT('Ctrl Pts',(1.232277448493,-0.1243010718991,-27.70332906285));
#24280=CARTESIAN_POINT('Ctrl Pts',(0.8306647230819,-0.9186700084293,-27.76182906285));
#24281=CARTESIAN_POINT('Ctrl Pts',(0.,-1.23853076932,-27.82032906285));
#24282=CARTESIAN_POINT('Ctrl Pts',(-0.8306647230819,-0.9186700084293,-27.87882906285));
#24283=CARTESIAN_POINT('Ctrl Pts',(-1.232277448493,-0.1243010718991,-27.93732906285));
#24284=CARTESIAN_POINT('Ctrl Pts',(-0.9973985952511,0.7342714135493,-27.99582906285));
#24285=CARTESIAN_POINT('Ctrl Pts',(-0.2473469557286,1.213580631934,-28.05432906285));
#24286=CARTESIAN_POINT('Ctrl Pts',(0.6304634559708,1.066055484586,-28.11282906285));
#24287=CARTESIAN_POINT('Ctrl Pts',(1.182629120302,0.3678951396931,-28.17132906285));
#24288=CARTESIAN_POINT('Ctrl Pts',(1.123947378369,-0.5202891046535,-28.22982906285));
#24289=CARTESIAN_POINT('Ctrl Pts',(0.4847283440002,-1.139735441963,-28.28832906285));
#24290=CARTESIAN_POINT('Ctrl Pts',(-0.4048609400269,-1.170489756933,-28.34682906285));
#24291=CARTESIAN_POINT('Ctrl Pts',(-1.08533257321,-0.5966665270227,-28.40532906285));
#24292=CARTESIAN_POINT('Ctrl Pts',(-1.205213243798,0.2853435668963,-28.46382906285));
#24293=CARTESIAN_POINT('Ctrl Pts',(-0.7025770758952,1.019973547991,-28.52232906285));
#24294=CARTESIAN_POINT('Ctrl Pts',(0.1629354149332,1.227753484752,-28.58082906285));
#24295=CARTESIAN_POINT('Ctrl Pts',(0.9443499054416,0.8014417043471,-28.63932906285));
#24296=CARTESIAN_POINT('Ctrl Pts',(1.237765138237,-0.03906361929905,-28.69782906285));
#24297=CARTESIAN_POINT('Ctrl Pts',(1.007722685201,-0.585362698559,-28.73682906285));
#24298=CARTESIAN_POINT('Ctrl Pts',(0.8153253598169,-0.7851534710925,-28.75632906285));
#24299=CARTESIAN_POINT('',(1.42616365839207,-0.463388665150997,-28.5080680843046));
#24300=CARTESIAN_POINT('',(1.426584774443,-0.4635254915624,-28.5078125));
#24301=CARTESIAN_POINT('Ctrl Pts',(1.42592296431875,-0.463335877700853,
-28.5076220976351));
#24302=CARTESIAN_POINT('Ctrl Pts',(1.4516646730899,-0.383939856993698,-28.503323569032));
#24303=CARTESIAN_POINT('Ctrl Pts',(1.47080306466018,-0.302401817242002,
-28.4990861959195));
#24304=CARTESIAN_POINT('Ctrl Pts',(1.49271878036586,-0.154988761660788,
-28.4913957131492));
#24305=CARTESIAN_POINT('Ctrl Pts',(1.49813264451624,-0.0894476287888264,
-28.4879643848815));
#24306=CARTESIAN_POINT('Ctrl Pts',(1.5006482312565,0.0698946699337639,-28.4793972302415));
#24307=CARTESIAN_POINT('Ctrl Pts',(1.49328387783098,0.163646013371891,-28.4741909039621));
#24308=CARTESIAN_POINT('Ctrl Pts',(1.46690763178642,0.315977876498846,-28.4656689062437));
#24309=CARTESIAN_POINT('Ctrl Pts',(1.45284440993149,0.375451041534454,-28.4623263523921));
#24310=CARTESIAN_POINT('Ctrl Pts',(1.40056433535711,0.548273795567868,-28.4526654076531));
#24311=CARTESIAN_POINT('Ctrl Pts',(1.35213073740469,0.658369858497446,-28.4466068811747));
#24312=CARTESIAN_POINT('Ctrl Pts',(1.25646955925034,0.820805928945592,-28.436976157127));
#24313=CARTESIAN_POINT('Ctrl Pts',(1.21727123019692,0.878004524876435,-28.4334250716445));
#24314=CARTESIAN_POINT('Ctrl Pts',(1.10251991809743,1.02275181198366,-28.4237016458728));
#24315=CARTESIAN_POINT('Ctrl Pts',(1.02042512302908,1.10451558663737,-28.4173189735821));
#24316=CARTESIAN_POINT('Ctrl Pts',(0.881164643456005,1.21473017110051,-28.4075323182098));
#24317=CARTESIAN_POINT('Ctrl Pts',(0.829533462102437,1.25058483394728,-28.4040917352513));
#24318=CARTESIAN_POINT('Ctrl Pts',(0.675514033222316,1.34367687607065,-28.3944542505251));
#24319=CARTESIAN_POINT('Ctrl Pts',(0.568131647479671,1.39230007563897,-28.3884997720049));
#24320=CARTESIAN_POINT('Ctrl Pts',(0.389136578471147,1.44958560114917,-28.37889107636));
#24321=CARTESIAN_POINT('Ctrl Pts',(0.320018924005801,1.46645692540373,-28.3752483096082));
#24322=CARTESIAN_POINT('Ctrl Pts',(0.134162099992888,1.4980066036685,-28.3653254266851));
#24323=CARTESIAN_POINT('Ctrl Pts',(0.0164281179871881,1.50378688439387,
-28.3588302237474));
#24324=CARTESIAN_POINT('Ctrl Pts',(-0.162337185079902,1.49183709314879,
-28.3489565986272));
#24325=CARTESIAN_POINT('Ctrl Pts',(-0.224273388847288,1.48381261253025,
-28.3455389282578));
#24326=CARTESIAN_POINT('Ctrl Pts',(-0.401194807636539,1.44946528421081,
-28.335889754369));
#24327=CARTESIAN_POINT('Ctrl Pts',(-0.514067816300854,1.41320064504075,
-28.3299056019057));
#24328=CARTESIAN_POINT('Ctrl Pts',(-0.685303550305146,1.33529407650487,
-28.3202890842721));
#24329=CARTESIAN_POINT('Ctrl Pts',(-0.74742371702866,1.30161270724248,-28.3166707000832));
#24330=CARTESIAN_POINT('Ctrl Pts',(-0.905674963820369,1.20070679515175,
-28.306791048473));
#24331=CARTESIAN_POINT('Ctrl Pts',(-0.99658655727132,1.12622597733011,-28.3003149224196));
#24332=CARTESIAN_POINT('Ctrl Pts',(-1.12095380474306,0.997698499287579,
-28.2904587338548));
#24333=CARTESIAN_POINT('Ctrl Pts',(-1.16153071863231,0.950185721820537,
-28.2870394568104));
#24334=CARTESIAN_POINT('Ctrl Pts',(-1.2696777687758,0.806104733354828,-28.277393898246));
#24335=CARTESIAN_POINT('Ctrl Pts',(-1.32903537158566,0.703594749870364,
-28.2714142267783));
#24336=CARTESIAN_POINT('Ctrl Pts',(-1.40381150836108,0.53101108089913,-28.2617995366514));
#24337=CARTESIAN_POINT('Ctrl Pts',(-1.42732663669233,0.464310956122346,
-28.2581781571965));
#24338=CARTESIAN_POINT('Ctrl Pts',(-1.47705738103529,0.283275185944521,
-28.2482956416959));
#24339=CARTESIAN_POINT('Ctrl Pts',(-1.49454352171617,0.167060440209565,
-28.2418198776906));
#24340=CARTESIAN_POINT('Ctrl Pts',(-1.50060179387312,-0.0116989017369946,
-28.2319629537923));
#24341=CARTESIAN_POINT('Ctrl Pts',(-1.49883556041021,-0.0741723425411832,
-28.2285427453193));
#24342=CARTESIAN_POINT('Ctrl Pts',(-1.48242439855621,-0.253579384345749,
-28.2188969692646));
#24343=CARTESIAN_POINT('Ctrl Pts',(-1.45770808385869,-0.369412498303161,
-28.2129179176856));
#24344=CARTESIAN_POINT('Ctrl Pts',(-1.39743345394519,-0.547577876420512,
-28.2033032573019));
#24345=CARTESIAN_POINT('Ctrl Pts',(-1.37013861575826,-0.612836186582772,
-28.1996812284657));
#24346=CARTESIAN_POINT('Ctrl Pts',(-1.28559069101167,-0.780517974958821,
-28.1897961151518));
#24347=CARTESIAN_POINT('Ctrl Pts',(-1.22059622835544,-0.878477224158937,
-28.1833182398528));
#24348=CARTESIAN_POINT('Ctrl Pts',(-1.10517739974363,-1.01514695362663,
-28.1734599981016));
#24349=CARTESIAN_POINT('Ctrl Pts',(-1.06197439538667,-1.06029133708738,
-28.1700404840139));
#24350=CARTESIAN_POINT('Ctrl Pts',(-0.929492016747349,-1.18233895555091,
-28.1603961172978));
#24351=CARTESIAN_POINT('Ctrl Pts',(-0.833481330188796,-1.25167244016774,
-28.1544177203215));
#24352=CARTESIAN_POINT('Ctrl Pts',(-0.669291333748551,-1.34339519624346,
-28.1448037300712));
#24353=CARTESIAN_POINT('Ctrl Pts',(-0.605277730231828,-1.37349435639921,
-28.1411817119154));
#24354=CARTESIAN_POINT('Ctrl Pts',(-0.430071077583583,-1.44117968319116,
-28.1312948271126));
#24355=CARTESIAN_POINT('Ctrl Pts',(-0.316127250170529,-1.47025476212026,
-28.1248149638959));
#24356=CARTESIAN_POINT('Ctrl Pts',(-0.13883142420414,-1.49421045876829,
-28.1149556143986));
#24357=CARTESIAN_POINT('Ctrl Pts',(-0.0765212037758559,-1.49871626806615,
-28.1115368660599));
#24358=CARTESIAN_POINT('Ctrl Pts',(0.103476408041793,-1.5003822934613,-28.1018993613209));
#24359=CARTESIAN_POINT('Ctrl Pts',(0.22107994522376,-1.48743842556337,-28.0959263852764));
#24360=CARTESIAN_POINT('Ctrl Pts',(0.404325714405427,-1.44540238901112,
-28.0863159307243));
#24361=CARTESIAN_POINT('Ctrl Pts',(0.472039677844878,-1.4247919824078,-28.0826917867747));
#24362=CARTESIAN_POINT('Ctrl Pts',(0.647640177920739,-1.35741391816062,
-28.0727916994037));
#24363=CARTESIAN_POINT('Ctrl Pts',(0.751841587366556,-1.30244714266978,
-28.0662996627543));
#24364=CARTESIAN_POINT('Ctrl Pts',(0.899497233796535,-1.20118067772247,
-28.056432960265));
#24365=CARTESIAN_POINT('Ctrl Pts',(0.948670279861992,-1.16276469467675,
-28.0530184176353));
#24366=CARTESIAN_POINT('Ctrl Pts',(1.08284208874631,-1.04364124354584,-28.0434127722028));
#24367=CARTESIAN_POINT('Ctrl Pts',(1.16107831074709,-0.955578476827092,
-28.037464424286));
#24368=CARTESIAN_POINT('Ctrl Pts',(1.26875583948425,-0.801842443670456,
-28.0278703050064));
#24369=CARTESIAN_POINT('Ctrl Pts',(1.30529835608295,-0.740996048005445,
-28.0242368253798));
#24370=CARTESIAN_POINT('Ctrl Pts',(1.39096959843416,-0.57223109919015,-28.0142761029451));
#24371=CARTESIAN_POINT('Ctrl Pts',(1.43167640473481,-0.460613253287086,
-28.0077276139323));
#24372=CARTESIAN_POINT('Ctrl Pts',(1.47316553590904,-0.285785232077346,
-27.9978269398273));
#24373=CARTESIAN_POINT('Ctrl Pts',(1.48374413368801,-0.224631418430332,
-27.9944319379755));
#24374=CARTESIAN_POINT('Ctrl Pts',(1.50292114375066,-0.0489988829097152,
-27.984976375275));
#24375=CARTESIAN_POINT('Ctrl Pts',(1.50209457818614,0.0663516175829957,
-27.9791444841177));
#24376=CARTESIAN_POINT('Ctrl Pts',(1.47976056185988,0.251244628382758,-27.9696267163725));
#24377=CARTESIAN_POINT('Ctrl Pts',(1.46608945011532,0.321842819328718,-27.965948568838));
#24378=CARTESIAN_POINT('Ctrl Pts',(1.42554988683578,0.47224606533571,-27.9577565207606));
#24379=CARTESIAN_POINT('Ctrl Pts',(1.396869339743,0.551196312457827,-27.9531910439495));
#24380=CARTESIAN_POINT('Ctrl Pts',(1.32828966134185,0.700068795939468,-27.9441614169721));
#24381=CARTESIAN_POINT('Ctrl Pts',(1.28886638514574,0.770287049061794,-27.9397080725723));
#24382=CARTESIAN_POINT('Ctrl Pts',(1.20105115222611,0.900844271197268,-27.9311879209186));
#24383=CARTESIAN_POINT('Ctrl Pts',(1.15323605214701,0.961173009596781,-27.927159390159));
#24384=CARTESIAN_POINT('Ctrl Pts',(1.03113117407888,1.09313678043491,-27.9178923624111));
#24385=CARTESIAN_POINT('Ctrl Pts',(0.953425800183683,1.16155713534289,-27.9126923047804));
#24386=CARTESIAN_POINT('Ctrl Pts',(0.806967245432844,1.26598668165696,-27.9033645286779));
#24387=CARTESIAN_POINT('Ctrl Pts',(0.741210820501912,1.30561869878126,-27.8992943166603));
#24388=CARTESIAN_POINT('Ctrl Pts',(0.583394542925378,1.38477568346781,-27.8896647037835));
#24389=CARTESIAN_POINT('Ctrl Pts',(0.489886871548345,1.42055251867229,-27.8841013444146));
#24390=CARTESIAN_POINT('Ctrl Pts',(0.31938036937766,1.46698849926037,-27.8744730836011));
#24391=CARTESIAN_POINT('Ctrl Pts',(0.243795335422544,1.48137909149889,-27.8704031474391));
#24392=CARTESIAN_POINT('Ctrl Pts',(0.0683128605550142,1.50095679663137,
-27.8612572972935));
#24393=CARTESIAN_POINT('Ctrl Pts',(-0.0317413520965657,1.50215917195855,
-27.8562262675331));
#24394=CARTESIAN_POINT('Ctrl Pts',(-0.209504424270073,1.48668492189799,
-27.84703302098));
#24395=CARTESIAN_POINT('Ctrl Pts',(-0.287482309193275,1.47367742627492,
-27.8428971115734));
#24396=CARTESIAN_POINT('Ctrl Pts',(-0.439655506240912,1.43555467259612,
-27.834397355129));
#24397=CARTESIAN_POINT('Ctrl Pts',(-0.513570900963485,1.41077773370975,
-27.8300876827913));
#24398=CARTESIAN_POINT('Ctrl Pts',(-0.668050563795896,1.3453186100834,-27.8208425020254));
#24399=CARTESIAN_POINT('Ctrl Pts',(-0.747822759524413,1.30272527256634,
-27.8159338884917));
#24400=CARTESIAN_POINT('Ctrl Pts',(-0.885124648788246,1.21236367813823,
-27.807317523479));
#24401=CARTESIAN_POINT('Ctrl Pts',(-0.943812698786729,1.16718169249958,
-27.8035396650792));
#24402=CARTESIAN_POINT('Ctrl Pts',(-1.08231919829256,1.04341463201487,-27.7940507301813));
#24403=CARTESIAN_POINT('Ctrl Pts',(-1.1575952931583,0.959492955612986,-27.7883285298767));
#24404=CARTESIAN_POINT('Ctrl Pts',(-1.25989871101654,0.815423160489302,
-27.7788404489654));
#24405=CARTESIAN_POINT('Ctrl Pts',(-1.29377727498199,0.760480307524973,
-27.7752997519017));
#24406=CARTESIAN_POINT('Ctrl Pts',(-1.37807329817412,0.601832309402957,
-27.7653917063489));
#24407=CARTESIAN_POINT('Ctrl Pts',(-1.42053833023185,0.493679521843405,
-27.7590125196674));
#24408=CARTESIAN_POINT('Ctrl Pts',(-1.46840257130333,0.311276579656757,
-27.7491172618014));
#24409=CARTESIAN_POINT('Ctrl Pts',(-1.48170726052789,0.239717958079749,
-27.7454006524031));
#24410=CARTESIAN_POINT('Ctrl Pts',(-1.50268591701451,0.0530482402031576,
-27.7358035549755));
#24411=CARTESIAN_POINT('Ctrl Pts',(-1.50248033205375,-0.0631325833269582,
-27.7299161711196));
#24412=CARTESIAN_POINT('Ctrl Pts',(-1.48106199660676,-0.242436234610995,
-27.7202154298389));
#24413=CARTESIAN_POINT('Ctrl Pts',(-1.4691465541843,-0.306362650752422,
-27.7166470421241));
#24414=CARTESIAN_POINT('Ctrl Pts',(-1.42512121626003,-0.47958137707748,
-27.7067890874004));
#24415=CARTESIAN_POINT('Ctrl Pts',(-1.38450563573437,-0.586910041995524,
-27.700490602839));
#24416=CARTESIAN_POINT('Ctrl Pts',(-1.29855947816122,-0.752865717018401,
-27.6906817952317));
#24417=CARTESIAN_POINT('Ctrl Pts',(-1.26063238477963,-0.814672299671888,
-27.6869780558361));
#24418=CARTESIAN_POINT('Ctrl Pts',(-1.15091158538457,-0.967701024939023,
-27.6773574534304));
#24419=CARTESIAN_POINT('Ctrl Pts',(-1.07238295580389,-1.05432331995669,
-27.6714347471479));
#24420=CARTESIAN_POINT('Ctrl Pts',(-0.935579451561983,-1.1734668006248,
-27.6616882873619));
#24421=CARTESIAN_POINT('Ctrl Pts',(-0.883768673628082,-1.21293683651046,
-27.6581138308857));
#24422=CARTESIAN_POINT('Ctrl Pts',(-0.735058866113722,-1.3117119427223,
-27.6482667621033));
#24423=CARTESIAN_POINT('Ctrl Pts',(-0.633217770969367,-1.36392203649838,
-27.6419858399696));
#24424=CARTESIAN_POINT('Ctrl Pts',(-0.458516968014841,-1.42927184788114,
-27.6321958325746));
#24425=CARTESIAN_POINT('Ctrl Pts',(-0.388991906692596,-1.44967668597002,
-27.6284948692181));
#24426=CARTESIAN_POINT('Ctrl Pts',(-0.204886892472027,-1.48966431845479,
-27.6188691445367));
#24427=CARTESIAN_POINT('Ctrl Pts',(-0.088384316819463,-1.50127550237707,
-27.6129387749736));
#24428=CARTESIAN_POINT('Ctrl Pts',(0.0931773509636978,-1.49788323251699,
-27.603182377091));
#24429=CARTESIAN_POINT('Ctrl Pts',(0.158102115673349,-1.49240393028911,
-27.5996065876513));
#24430=CARTESIAN_POINT('Ctrl Pts',(0.334605703811802,-1.46592065586156,
-27.5897619864405));
#24431=CARTESIAN_POINT('Ctrl Pts',(0.445093451049737,-1.43635788839267,
-27.5834849942358));
#24432=CARTESIAN_POINT('Ctrl Pts',(0.618429402724692,-1.36769837238986,
-27.573699316174));
#24433=CARTESIAN_POINT('Ctrl Pts',(0.68367212242673,-1.33621387385003,-27.5699990873574));
#24434=CARTESIAN_POINT('Ctrl Pts',(0.847075172364305,-1.24239707625671,
-27.5603722090784));
#24435=CARTESIAN_POINT('Ctrl Pts',(0.941310341369421,-1.17285269806391,
-27.5544400135388));
#24436=CARTESIAN_POINT('Ctrl Pts',(1.07373531512154,-1.04853649392191,-27.5446814006941));
#24437=CARTESIAN_POINT('Ctrl Pts',(1.11821899467738,-1.00092565180024,-27.5411054558441));
#24438=CARTESIAN_POINT('Ctrl Pts',(1.23137427531208,-0.86290252007411,-27.5312608956508));
#24439=CARTESIAN_POINT('Ctrl Pts',(1.29349708821054,-0.76687450479305,-27.5249841244415));
#24440=CARTESIAN_POINT('Ctrl Pts',(1.37601842237683,-0.59969000756072,-27.5151982923214));
#24441=CARTESIAN_POINT('Ctrl Pts',(1.40329689371724,-0.532573066997368,
-27.5114977353222));
#24442=CARTESIAN_POINT('Ctrl Pts',(1.46157520466307,-0.353389922872069,
-27.5018707007339));
#24443=CARTESIAN_POINT('Ctrl Pts',(1.4848282527389,-0.238607462222975,-27.4959386516808));
#24444=CARTESIAN_POINT('Ctrl Pts',(1.49967452896699,-0.0575740238518383,
-27.4861796041596));
#24445=CARTESIAN_POINT('Ctrl Pts',(1.50073662771819,0.00758669747972766,
-27.4826030317379));
#24446=CARTESIAN_POINT('Ctrl Pts',(1.49209334404164,0.185831428521481,-27.4727598316343));
#24447=CARTESIAN_POINT('Ctrl Pts',(1.47377345415873,0.298688849505142,-27.4664850934286));
#24448=CARTESIAN_POINT('Ctrl Pts',(1.42287499434697,0.477994779563694,-27.4567019590445));
#24449=CARTESIAN_POINT('Ctrl Pts',(1.39810301767802,0.546059877122668,-27.4530022054626));
#24450=CARTESIAN_POINT('Ctrl Pts',(1.3211654313417,0.718060732051041,-27.4433751381407));
#24451=CARTESIAN_POINT('Ctrl Pts',(1.26142600296818,0.818813512273715,-27.437442313619));
#24452=CARTESIAN_POINT('Ctrl Pts',(1.15102961233378,0.963050066249823,-27.4276836194461));
#24453=CARTESIAN_POINT('Ctrl Pts',(1.10813272831953,1.01208011949452,-27.4241083088924));
#24454=CARTESIAN_POINT('Ctrl Pts',(0.982182829837723,1.13850704971315,-27.4142648510938));
#24455=CARTESIAN_POINT('Ctrl Pts',(0.89288499655155,1.20995281268992,-27.4079884319172));
#24456=CARTESIAN_POINT('Ctrl Pts',(0.734889103031064,1.30881027007612,-27.3982060630653));
#24457=CARTESIAN_POINT('Ctrl Pts',(0.670903938435668,1.34266718389571,-27.3945084402764));
#24458=CARTESIAN_POINT('Ctrl Pts',(0.498457411270812,1.41867699508727,-27.384880025534));
#24459=CARTESIAN_POINT('Ctrl Pts',(0.386502941276246,1.45336875310848,-27.3789439127497));
#24460=CARTESIAN_POINT('Ctrl Pts',(0.207819195303042,1.4863173466136,-27.369182131404));
#24461=CARTESIAN_POINT('Ctrl Pts',(0.143130180356492,1.49391137164654,-27.3656076151228));
#24462=CARTESIAN_POINT('Ctrl Pts',(-0.0353700157144279,1.50322767800781,
-27.3557483256202));
#24463=CARTESIAN_POINT('Ctrl Pts',(-0.149822348418008,1.49627831076344,
-27.3494556410944));
#24464=CARTESIAN_POINT('Ctrl Pts',(-0.334031956674721,1.46339901016027,
-27.3396342747821));
#24465=CARTESIAN_POINT('Ctrl Pts',(-0.404614812010914,1.44541578204513,
-27.3359139830926));
#24466=CARTESIAN_POINT('Ctrl Pts',(-0.583249552166997,1.38593269121057,
-27.3262924142867));
#24467=CARTESIAN_POINT('Ctrl Pts',(-0.688942046966698,1.33675561562416,
-27.3203839820944));
#24468=CARTESIAN_POINT('Ctrl Pts',(-0.843365846049652,1.24143204859706,
-27.310632267231));
#24469=CARTESIAN_POINT('Ctrl Pts',(-0.896743611832975,1.20341140088442,
-27.3070351784615));
#24470=CARTESIAN_POINT('Ctrl Pts',(-1.03400096505333,1.09149366715439,-27.2972677764508));
#24471=CARTESIAN_POINT('Ctrl Pts',(-1.11286165108869,1.01112828548998,-27.2910898599694));
#24472=CARTESIAN_POINT('Ctrl Pts',(-1.2254782116242,0.866621664760356,-27.2814734939252));
#24473=CARTESIAN_POINT('Ctrl Pts',(-1.2650223103723,0.807682555639639,-27.2778476847045));
#24474=CARTESIAN_POINT('Ctrl Pts',(-1.35902803315271,0.643804534153842,
-27.2682017101556));
#24475=CARTESIAN_POINT('Ctrl Pts',(-1.40588725048421,0.534289432650414,
-27.2621823588722));
#24476=CARTESIAN_POINT('Ctrl Pts',(-1.45696707977077,0.35954224854904,-27.2524064771433));
#24477=CARTESIAN_POINT('Ctrl Pts',(-1.47087854861132,0.297450853862337,
-27.2489159472829));
#24478=CARTESIAN_POINT('Ctrl Pts',(-1.49565959677105,0.141117025706754,
-27.2401810071786));
#24479=CARTESIAN_POINT('Ctrl Pts',(-1.50165986851533,0.0460511064130723,
-27.234919360292));
#24480=CARTESIAN_POINT('Ctrl Pts',(-1.49516929085166,-0.152692475519053,
-27.2242975539347));
#24481=CARTESIAN_POINT('Ctrl Pts',(-1.48083468356298,-0.256280444645493,
-27.2189780886341));
#24482=CARTESIAN_POINT('Ctrl Pts',(-1.4473097275385,-0.393008834830006,
-27.2117760764486));
#24483=CARTESIAN_POINT('Ctrl Pts',(-1.4372563590701,-0.428379884357375,
-27.2098954320207));
#24484=CARTESIAN_POINT('Ctrl Pts',(-1.42592304848998,-0.463335618088616,
-27.2080029164204));
#24485=CARTESIAN_POINT('Ctrl Pts',(-0.8153253598169,-0.7851534710925,-26.95929593715));
#24486=CARTESIAN_POINT('Ctrl Pts',(-1.007722685201,-0.585362698559,-26.97879593715));
#24487=CARTESIAN_POINT('Ctrl Pts',(-1.237765138237,-0.03906361929903,-27.01779593715));
#24488=CARTESIAN_POINT('Ctrl Pts',(-0.9443499054416,0.8014417043471,-27.07629593715));
#24489=CARTESIAN_POINT('Ctrl Pts',(-0.1629354149332,1.227753484752,-27.13479593715));
#24490=CARTESIAN_POINT('Ctrl Pts',(0.7025770758952,1.019973547991,-27.19329593715));
#24491=CARTESIAN_POINT('Ctrl Pts',(1.205213243798,0.2853435668963,-27.25179593715));
#24492=CARTESIAN_POINT('Ctrl Pts',(1.08533257321,-0.5966665270227,-27.31029593715));
#24493=CARTESIAN_POINT('Ctrl Pts',(0.4048609400268,-1.170489756933,-27.36879593715));
#24494=CARTESIAN_POINT('Ctrl Pts',(-0.4847283440002,-1.139735441963,-27.42729593715));
#24495=CARTESIAN_POINT('Ctrl Pts',(-1.123947378369,-0.5202891046535,-27.48579593715));
#24496=CARTESIAN_POINT('Ctrl Pts',(-1.182629120302,0.3678951396931,-27.54429593715));
#24497=CARTESIAN_POINT('Ctrl Pts',(-0.6304634559708,1.066055484586,-27.60279593715));
#24498=CARTESIAN_POINT('Ctrl Pts',(0.2473469557286,1.213580631934,-27.66129593715));
#24499=CARTESIAN_POINT('Ctrl Pts',(0.9973985952512,0.7342714135492,-27.71979593715));
#24500=CARTESIAN_POINT('Ctrl Pts',(1.232277448493,-0.1243010718991,-27.77829593715));
#24501=CARTESIAN_POINT('Ctrl Pts',(0.8306647230819,-0.9186700084293,-27.83679593715));
#24502=CARTESIAN_POINT('Ctrl Pts',(0.,-1.23853076932,-27.89529593715));
#24503=CARTESIAN_POINT('Ctrl Pts',(-0.8306647230819,-0.9186700084293,-27.95379593715));
#24504=CARTESIAN_POINT('Ctrl Pts',(-1.232277448493,-0.1243010718991,-28.01229593715));
#24505=CARTESIAN_POINT('Ctrl Pts',(-0.9973985952511,0.7342714135493,-28.07079593715));
#24506=CARTESIAN_POINT('Ctrl Pts',(-0.2473469557286,1.213580631934,-28.12929593715));
#24507=CARTESIAN_POINT('Ctrl Pts',(0.6304634559708,1.066055484586,-28.18779593715));
#24508=CARTESIAN_POINT('Ctrl Pts',(1.182629120302,0.3678951396931,-28.24629593715));
#24509=CARTESIAN_POINT('Ctrl Pts',(1.123947378369,-0.5202891046535,-28.30479593715));
#24510=CARTESIAN_POINT('Ctrl Pts',(0.4847283440002,-1.139735441963,-28.36329593715));
#24511=CARTESIAN_POINT('Ctrl Pts',(-0.4048609400269,-1.170489756933,-28.42179593715));
#24512=CARTESIAN_POINT('Ctrl Pts',(-1.08533257321,-0.5966665270227,-28.48029593715));
#24513=CARTESIAN_POINT('Ctrl Pts',(-1.205213243798,0.2853435668963,-28.53879593715));
#24514=CARTESIAN_POINT('Ctrl Pts',(-0.7025770758952,1.019973547991,-28.59729593715));
#24515=CARTESIAN_POINT('Ctrl Pts',(0.1629354149332,1.227753484752,-28.65579593715));
#24516=CARTESIAN_POINT('Ctrl Pts',(0.9443499054416,0.8014417043471,-28.71429593715));
#24517=CARTESIAN_POINT('Ctrl Pts',(1.237765138237,-0.03906361929905,-28.77279593715));
#24518=CARTESIAN_POINT('Ctrl Pts',(1.007722685201,-0.585362698559,-28.81179593715));
#24519=CARTESIAN_POINT('Ctrl Pts',(0.8153253598169,-0.7851534710925,-28.83129593715));
#24520=CARTESIAN_POINT('Ctrl Pts',(-0.9121267933018,-0.8783726756619,-27.03688532136));
#24521=CARTESIAN_POINT('Ctrl Pts',(-1.12736694661,-0.6548612706895,-27.05638532136));
#24522=CARTESIAN_POINT('Ctrl Pts',(-1.384721734467,-0.04370153997662,-27.09538532136));
#24523=CARTESIAN_POINT('Ctrl Pts',(-1.056470083549,0.8965947679692,-27.15388532136));
#24524=CARTESIAN_POINT('Ctrl Pts',(-0.1822803077923,1.373521423722,-27.21238532136));
#24525=CARTESIAN_POINT('Ctrl Pts',(0.7859922024595,1.141072322086,-27.27088532136));
#24526=CARTESIAN_POINT('Ctrl Pts',(1.3483050393,0.3192216573772,-27.32938532136));
#24527=CARTESIAN_POINT('Ctrl Pts',(1.2141912523,-0.6675071729475,-27.38788532136));
#24528=CARTESIAN_POINT('Ctrl Pts',(0.4529290135692,-1.309458924255,-27.44638532136));
#24529=CARTESIAN_POINT('Ctrl Pts',(-0.5422788641515,-1.275053230434,-27.50488532136));
#24530=CARTESIAN_POINT('Ctrl Pts',(-1.257390691615,-0.5820616602972,-27.56338532136));
#24531=CARTESIAN_POINT('Ctrl Pts',(-1.323039562278,0.4115743610808,-27.62188532136));
#24532=CARTESIAN_POINT('Ctrl Pts',(-0.7053167222932,1.192625445694,-27.68038532136));
#24533=CARTESIAN_POINT('Ctrl Pts',(0.2767138085983,1.357665865401,-27.73888532136));
#24534=CARTESIAN_POINT('Ctrl Pts',(1.11581710464,0.8214495253824,-27.79738532136));
#24535=CARTESIAN_POINT('Ctrl Pts',(1.378582505767,-0.1390590109215,-27.85588532136));
#24536=CARTESIAN_POINT('Ctrl Pts',(0.9292873587837,-1.027741279971,-27.91438532136));
#24537=CARTESIAN_POINT('Ctrl Pts',(0.,-1.385578266913,-27.97288532136));
#24538=CARTESIAN_POINT('Ctrl Pts',(-0.9292873587837,-1.027741279971,-28.03138532136));
#24539=CARTESIAN_POINT('Ctrl Pts',(-1.378582505767,-0.1390590109215,-28.08988532136));
#24540=CARTESIAN_POINT('Ctrl Pts',(-1.11581710464,0.8214495253824,-28.14838532136));
#24541=CARTESIAN_POINT('Ctrl Pts',(-0.2767138085983,1.357665865401,-28.20688532136));
#24542=CARTESIAN_POINT('Ctrl Pts',(0.7053167222932,1.192625445694,-28.26538532136));
#24543=CARTESIAN_POINT('Ctrl Pts',(1.323039562278,0.4115743610808,-28.32388532136));
#24544=CARTESIAN_POINT('Ctrl Pts',(1.257390691615,-0.5820616602972,-28.38238532136));
#24545=CARTESIAN_POINT('Ctrl Pts',(0.5422788641515,-1.275053230434,-28.44088532136));
#24546=CARTESIAN_POINT('Ctrl Pts',(-0.4529290135692,-1.309458924255,-28.49938532136));
#24547=CARTESIAN_POINT('Ctrl Pts',(-1.2141912523,-0.6675071729475,-28.55788532136));
#24548=CARTESIAN_POINT('Ctrl Pts',(-1.3483050393,0.3192216573772,-28.61638532136));
#24549=CARTESIAN_POINT('Ctrl Pts',(-0.7859922024595,1.141072322086,-28.67488532136));
#24550=CARTESIAN_POINT('Ctrl Pts',(0.1822803077923,1.373521423722,-28.73338532136));
#24551=CARTESIAN_POINT('Ctrl Pts',(1.056470083549,0.8965947679692,-28.79188532136));
#24552=CARTESIAN_POINT('Ctrl Pts',(1.384721734467,-0.04370153997664,-28.85038532136));
#24553=CARTESIAN_POINT('Ctrl Pts',(1.12736694661,-0.6548612706895,-28.88938532136));
#24554=CARTESIAN_POINT('Ctrl Pts',(0.9121267933018,-0.8783726756619,-28.90888532136));
#24555=CARTESIAN_POINT('Ctrl Pts',(-1.008928226787,-0.9715918802313,-27.11447470556));
#24556=CARTESIAN_POINT('Ctrl Pts',(-1.247011208018,-0.7243598428201,-27.13397470556));
#24557=CARTESIAN_POINT('Ctrl Pts',(-1.531678330698,-0.0483394606542,-27.17297470556));
#24558=CARTESIAN_POINT('Ctrl Pts',(-1.168590261656,0.9917478315913,-27.23147470556));
#24559=CARTESIAN_POINT('Ctrl Pts',(-0.2016252006515,1.519289362691,-27.28997470556));
#24560=CARTESIAN_POINT('Ctrl Pts',(0.8694073290239,1.262171096181,-27.34847470556));
#24561=CARTESIAN_POINT('Ctrl Pts',(1.491396834802,0.3530997478581,-27.40697470556));
#24562=CARTESIAN_POINT('Ctrl Pts',(1.34304993139,-0.7383478188722,-27.46547470556));
#24563=CARTESIAN_POINT('Ctrl Pts',(0.5009970871116,-1.448428091577,-27.52397470556));
#24564=CARTESIAN_POINT('Ctrl Pts',(-0.5998293843028,-1.410371018906,-27.58247470556));
#24565=CARTESIAN_POINT('Ctrl Pts',(-1.390834004861,-0.6438342159409,-27.64097470556));
#24566=CARTESIAN_POINT('Ctrl Pts',(-1.463450004255,0.4552535824685,-27.69947470556));
#24567=CARTESIAN_POINT('Ctrl Pts',(-0.7801699886157,1.319195406802,-27.75797470556));
#24568=CARTESIAN_POINT('Ctrl Pts',(0.3060806614679,1.501751098868,-27.81647470556));
#24569=CARTESIAN_POINT('Ctrl Pts',(1.234235614028,0.9086276372156,-27.87497470556));
#24570=CARTESIAN_POINT('Ctrl Pts',(1.524887563041,-0.1538169499438,-27.93347470556));
#24571=CARTESIAN_POINT('Ctrl Pts',(1.027909994485,-1.136812551513,-27.99197470556));
#24572=CARTESIAN_POINT('Ctrl Pts',(0.,-1.532625764506,-28.05047470556));
#24573=CARTESIAN_POINT('Ctrl Pts',(-1.027909994485,-1.136812551513,-28.10897470556));
#24574=CARTESIAN_POINT('Ctrl Pts',(-1.524887563041,-0.1538169499438,-28.16747470556));
#24575=CARTESIAN_POINT('Ctrl Pts',(-1.234235614028,0.9086276372156,-28.22597470556));
#24576=CARTESIAN_POINT('Ctrl Pts',(-0.3060806614679,1.501751098868,-28.28447470556));
#24577=CARTESIAN_POINT('Ctrl Pts',(0.7801699886157,1.319195406802,-28.34297470556));
#24578=CARTESIAN_POINT('Ctrl Pts',(1.463450004255,0.4552535824684,-28.40147470556));
#24579=CARTESIAN_POINT('Ctrl Pts',(1.390834004861,-0.6438342159409,-28.45997470556));
#24580=CARTESIAN_POINT('Ctrl Pts',(0.5998293843027,-1.410371018906,-28.51847470556));
#24581=CARTESIAN_POINT('Ctrl Pts',(-0.5009970871116,-1.448428091577,-28.57697470556));
#24582=CARTESIAN_POINT('Ctrl Pts',(-1.34304993139,-0.7383478188722,-28.63547470556));
#24583=CARTESIAN_POINT('Ctrl Pts',(-1.491396834802,0.3530997478581,-28.69397470556));
#24584=CARTESIAN_POINT('Ctrl Pts',(-0.8694073290239,1.262171096181,-28.75247470556));
#24585=CARTESIAN_POINT('Ctrl Pts',(0.2016252006515,1.519289362691,-28.81097470556));
#24586=CARTESIAN_POINT('Ctrl Pts',(1.168590261656,0.9917478315913,-28.86947470556));
#24587=CARTESIAN_POINT('Ctrl Pts',(1.531678330698,-0.04833946065422,-28.92797470556));
#24588=CARTESIAN_POINT('Ctrl Pts',(1.247011208018,-0.7243598428201,-28.96697470556));
#24589=CARTESIAN_POINT('Ctrl Pts',(1.008928226787,-0.9715918802313,-28.98647470556));
#24590=CARTESIAN_POINT('Ctrl Pts',(-1.105729660272,-1.064811084801,-27.19206408977));
#24591=CARTESIAN_POINT('Ctrl Pts',(-1.366655469426,-0.7938584149506,-27.21156408977));
#24592=CARTESIAN_POINT('Ctrl Pts',(-1.678634926928,-0.05297738133179,-27.25056408977));
#24593=CARTESIAN_POINT('Ctrl Pts',(-1.280710439764,1.086900895213,-27.30906408977));
#24594=CARTESIAN_POINT('Ctrl Pts',(-0.2209700935106,1.665057301661,-27.36756408977));
#24595=CARTESIAN_POINT('Ctrl Pts',(0.9528224555883,1.383269870276,-27.42606408977));
#24596=CARTESIAN_POINT('Ctrl Pts',(1.634488630304,0.386977838339,-27.48456408977));
#24597=CARTESIAN_POINT('Ctrl Pts',(1.47190861048,-0.809188464797,-27.54306408977));
#24598=CARTESIAN_POINT('Ctrl Pts',(0.549065160654,-1.5873972589,-27.60156408977));
#24599=CARTESIAN_POINT('Ctrl Pts',(-0.657379904454,-1.545688807378,-27.66006408977));
#24600=CARTESIAN_POINT('Ctrl Pts',(-1.524277318107,-0.7056067715846,-27.71856408977));
#24601=CARTESIAN_POINT('Ctrl Pts',(-1.603860446231,0.4989328038561,-27.77706408977));
#24602=CARTESIAN_POINT('Ctrl Pts',(-0.8550232549381,1.44576536791,-27.83556408977));
#24603=CARTESIAN_POINT('Ctrl Pts',(0.3354475143376,1.645836332335,-27.89406408977));
#24604=CARTESIAN_POINT('Ctrl Pts',(1.352654123417,0.9958057490488,-27.95256408977));
#24605=CARTESIAN_POINT('Ctrl Pts',(1.671192620316,-0.1685748889662,-28.01106408977));
#24606=CARTESIAN_POINT('Ctrl Pts',(1.126532630187,-1.245883823055,-28.06956408977));
#24607=CARTESIAN_POINT('Ctrl Pts',(0.,-1.6796732621,-28.12806408977));
#24608=CARTESIAN_POINT('Ctrl Pts',(-1.126532630187,-1.245883823055,-28.18656408977));
#24609=CARTESIAN_POINT('Ctrl Pts',(-1.671192620316,-0.1685748889661,-28.24506408977));
#24610=CARTESIAN_POINT('Ctrl Pts',(-1.352654123417,0.9958057490488,-28.30356408977));
#24611=CARTESIAN_POINT('Ctrl Pts',(-0.3354475143376,1.645836332335,-28.36206408977));
#24612=CARTESIAN_POINT('Ctrl Pts',(0.8550232549381,1.44576536791,-28.42056408977));
#24613=CARTESIAN_POINT('Ctrl Pts',(1.603860446231,0.4989328038561,-28.47906408977));
#24614=CARTESIAN_POINT('Ctrl Pts',(1.524277318107,-0.7056067715846,-28.53756408977));
#24615=CARTESIAN_POINT('Ctrl Pts',(0.657379904454,-1.545688807378,-28.59606408977));
#24616=CARTESIAN_POINT('Ctrl Pts',(-0.549065160654,-1.5873972589,-28.65456408977));
#24617=CARTESIAN_POINT('Ctrl Pts',(-1.47190861048,-0.809188464797,-28.71306408977));
#24618=CARTESIAN_POINT('Ctrl Pts',(-1.634488630304,0.3869778383391,-28.77156408977));
#24619=CARTESIAN_POINT('Ctrl Pts',(-0.9528224555883,1.383269870276,-28.83006408977));
#24620=CARTESIAN_POINT('Ctrl Pts',(0.2209700935106,1.665057301661,-28.88856408977));
#24621=CARTESIAN_POINT('Ctrl Pts',(1.280710439764,1.086900895213,-28.94706408977));
#24622=CARTESIAN_POINT('Ctrl Pts',(1.678634926928,-0.05297738133181,-29.00556408977));
#24623=CARTESIAN_POINT('Ctrl Pts',(1.366655469426,-0.7938584149506,-29.04456408977));
#24624=CARTESIAN_POINT('Ctrl Pts',(1.105729660272,-1.064811084801,-29.06406408977));
#24625=CARTESIAN_POINT('',(1.4261636598539,-0.463388660650212,-29.0075569156963));
#24626=CARTESIAN_POINT('Ctrl Pts',(1.42588748976426,-0.463325593694187,
-28.5076008391023));
#24627=CARTESIAN_POINT('Ctrl Pts',(1.36763435850362,-0.644240382503966,
-28.5176108865489));
#24628=CARTESIAN_POINT('Ctrl Pts',(1.27635777503622,-0.810368050117181,
-28.5280493786989));
#24629=CARTESIAN_POINT('Ctrl Pts',(1.04966047086561,-1.08239655987774,-28.5467699661616));
#24630=CARTESIAN_POINT('Ctrl Pts',(0.92408437639176,-1.19119500289366,-28.5551483209267));
#24631=CARTESIAN_POINT('Ctrl Pts',(0.650993762866597,-1.35990451072788,
-28.5719826080011));
#24632=CARTESIAN_POINT('Ctrl Pts',(0.506122406967541,-1.42066853677114,
-28.5805563431055));
#24633=CARTESIAN_POINT('Ctrl Pts',(0.17319726482727,-1.50083470355692,-28.5991123122149));
#24634=CARTESIAN_POINT('Ctrl Pts',(-0.0154175621686597,-1.51001365521321,
-28.6086217388051));
#24635=CARTESIAN_POINT('Ctrl Pts',(-0.290548624637289,-1.47357359252911,
-28.6230737569627));
#24636=CARTESIAN_POINT('Ctrl Pts',(-0.380656394221635,-1.4532427499571,
-28.6279092732768));
#24637=CARTESIAN_POINT('Ctrl Pts',(-0.55146398302981,-1.39751115884482,
-28.6375975079592));
#24638=CARTESIAN_POINT('Ctrl Pts',(-0.631949162462057,-1.36300673570578,
-28.6424324236474));
#24639=CARTESIAN_POINT('Ctrl Pts',(-0.872545759602894,-1.23342936288932,
-28.6572473951109));
#24640=CARTESIAN_POINT('Ctrl Pts',(-1.01929935175539,-1.1141922477245,-28.6667738905754));
#24641=CARTESIAN_POINT('Ctrl Pts',(-1.20040868387976,-0.902724249081157,
-28.6812689206855));
#24642=CARTESIAN_POINT('Ctrl Pts',(-1.25431324256695,-0.826787649429299,
-28.6861411185158));
#24643=CARTESIAN_POINT('Ctrl Pts',(-1.34485942327074,-0.669797661876857,
-28.6959089784289));
#24644=CARTESIAN_POINT('Ctrl Pts',(-1.38190065281194,-0.589606962202177,
-28.7007869332204));
#24645=CARTESIAN_POINT('Ctrl Pts',(-1.47404045297103,-0.331532746153138,
-28.7156502560038));
#24646=CARTESIAN_POINT('Ctrl Pts',(-1.50313736921478,-0.14475772903156,
-28.7251754824662));
#24647=CARTESIAN_POINT('Ctrl Pts',(-1.4946984766088,0.184912210312043,-28.7423412654415));
#24648=CARTESIAN_POINT('Ctrl Pts',(-1.47059029656801,0.328302251719719,
-28.7500231835792));
#24649=CARTESIAN_POINT('Ctrl Pts',(-1.38029529461018,0.604358529743169,
-28.7659327193717));
#24650=CARTESIAN_POINT('Ctrl Pts',(-1.31482559171509,0.734543079084308,
-28.7736172520995));
#24651=CARTESIAN_POINT('Ctrl Pts',(-1.12699633808168,1.00498587237804,-28.790749820465));
#24652=CARTESIAN_POINT('Ctrl Pts',(-0.993718884421314,1.13801109826558,
-28.80024663256));
#24653=CARTESIAN_POINT('Ctrl Pts',(-0.767703357131606,1.2914636138517,-28.8150755728019));
#24654=CARTESIAN_POINT('Ctrl Pts',(-0.690707069155562,1.33422204109302,
-28.819937578582));
#24655=CARTESIAN_POINT('Ctrl Pts',(-0.521044176936707,1.40932035982866,
-28.829930987713));
#24656=CARTESIAN_POINT('Ctrl Pts',(-0.42823822289558,1.43987608466915,-28.835031597656));
#24657=CARTESIAN_POINT('Ctrl Pts',(-0.15314209694067,1.50221839993919,-28.8497015983913));
#24658=CARTESIAN_POINT('Ctrl Pts',(0.0350342398075006,1.51046308074883,
-28.8592116967669));
#24659=CARTESIAN_POINT('Ctrl Pts',(0.310681305755836,1.47026975261959,-28.8743513270056));
#24660=CARTESIAN_POINT('Ctrl Pts',(0.401173810472036,1.44817012665623,-28.8794868055435));
#24661=CARTESIAN_POINT('Ctrl Pts',(0.584487442095495,1.38436006314717,-28.8898945742583));
#24662=CARTESIAN_POINT('Ctrl Pts',(0.676037547156664,1.34165567091835,-28.8951444215516));
#24663=CARTESIAN_POINT('Ctrl Pts',(0.907732947634239,1.20443826480559,-28.9091253563677));
#24664=CARTESIAN_POINT('Ctrl Pts',(1.05426821906179,1.08526766225066,-28.9186722332121));
#24665=CARTESIAN_POINT('Ctrl Pts',(1.23666629088399,0.853735003985556,-28.9347757104616));
#24666=CARTESIAN_POINT('Ctrl Pts',(1.28715303728387,0.775330858687689,-28.9398939533167));
#24667=CARTESIAN_POINT('Ctrl Pts',(1.37900484632935,0.597594224210385,-28.9505712707679));
#24668=CARTESIAN_POINT('Ctrl Pts',(1.41770465425374,0.497920187231623,-28.9560998903939));
#24669=CARTESIAN_POINT('Ctrl Pts',(1.48279256077328,0.259677223472442,-28.9689074648145));
#24670=CARTESIAN_POINT('Ctrl Pts',(1.50120345823689,0.118782629153447,-28.9761921486419));
#24671=CARTESIAN_POINT('Ctrl Pts',(1.49761271373553,-0.172199249620244,
-28.9918596395611));
#24672=CARTESIAN_POINT('Ctrl Pts',(1.47277821573864,-0.320301248088973,
-29.0000996307118));
#24673=CARTESIAN_POINT('Ctrl Pts',(1.42590316226892,-0.463277358684229,
-29.0080241608978));
#24674=CARTESIAN_POINT('',(1.109870874299,-0.360618907335,-28.81554752692));
#24675=CARTESIAN_POINT('Ctrl Pts',(1.121113703131,0.1559662789859,-28.75929593715));
#24676=CARTESIAN_POINT('Ctrl Pts',(1.1593323394,-0.1187561617546,-28.77879593715));
#24677=CARTESIAN_POINT('Ctrl Pts',(1.024334051204,-0.6959369621828,-28.81779593715));
#24678=CARTESIAN_POINT('Ctrl Pts',(0.2929195077513,-1.20345490624,-28.87629593715));
#24679=CARTESIAN_POINT('Ctrl Pts',(-0.5898378721215,-1.089044468041,-28.93479593715));
#24680=CARTESIAN_POINT('Ctrl Pts',(-1.167922203495,-0.4122114903279,-28.99329593715));
#24681=CARTESIAN_POINT('Ctrl Pts',(-1.142758736536,0.4775587757172,-29.05179593715));
#24682=CARTESIAN_POINT('Ctrl Pts',(-0.5273407111551,1.120655840702,-29.11029593715));
#24683=CARTESIAN_POINT('Ctrl Pts',(0.3604572362443,1.184917394878,-29.16879593715));
#24684=CARTESIAN_POINT('Ctrl Pts',(1.062073152252,0.6371491696676,-29.22729593715));
#24685=CARTESIAN_POINT('Ctrl Pts',(1.215110792527,-0.2397169657051,-29.28579593715));
#24686=CARTESIAN_POINT('Ctrl Pts',(0.7405237188655,-0.992765376005,-29.34429593715));
#24687=CARTESIAN_POINT('Ctrl Pts',(-0.1165560417524,-1.233034125506,-29.40279593715));
#24688=CARTESIAN_POINT('Ctrl Pts',(-0.9134326886102,-0.8364204625026,-29.46129593715));
#24689=CARTESIAN_POINT('Ctrl Pts',(-1.238506321788,-0.007781867099199,-29.51979593715));
#24690=CARTESIAN_POINT('Ctrl Pts',(-0.9238710607092,0.8248761905421,-29.57829593715));
#24691=CARTESIAN_POINT('Ctrl Pts',(-0.1320411949229,1.231472122869,-29.63679593715));
#24692=CARTESIAN_POINT('Ctrl Pts',(0.7279901207168,1.001992440436,-29.69529593715));
#24693=CARTESIAN_POINT('Ctrl Pts',(1.212002560279,0.2549671752147,-29.75379593715));
#24694=CARTESIAN_POINT('Ctrl Pts',(1.069995734522,-0.6237528313713,-29.81229593715));
#24695=CARTESIAN_POINT('Ctrl Pts',(0.3753185056597,-1.180294236991,-29.87079593715));
#24696=CARTESIAN_POINT('Ctrl Pts',(-0.5132169072275,-1.127194248056,-29.92929593715));
#24697=CARTESIAN_POINT('Ctrl Pts',(-1.136667342178,-0.4918798824477,-29.98779593715));
#24698=CARTESIAN_POINT('Ctrl Pts',(-1.173010393869,0.3974985356856,-30.04629593715));
#24699=CARTESIAN_POINT('Ctrl Pts',(-0.6034742672396,1.081562421011,-30.10479593715));
#24700=CARTESIAN_POINT('Ctrl Pts',(0.2777662163492,1.206981513611,-30.16329593715));
#24701=CARTESIAN_POINT('Ctrl Pts',(1.015535997925,0.7089748153235,-30.22179593715));
#24702=CARTESIAN_POINT('Ctrl Pts',(1.228764281396,-0.1552291200295,-30.28029593715));
#24703=CARTESIAN_POINT('Ctrl Pts',(0.80731725562,-0.9392543654266,-30.33879593715));
#24704=CARTESIAN_POINT('Ctrl Pts',(-0.03112861498029,-1.238140377948,-30.39729593715));
#24705=CARTESIAN_POINT('Ctrl Pts',(-0.8534729114545,-0.8975024000936,-30.45579593715));
#24706=CARTESIAN_POINT('Ctrl Pts',(-1.235070736526,-0.09330501139524,-30.51429593715));
#24707=CARTESIAN_POINT('Ctrl Pts',(-0.9784120125535,0.7591432259322,-30.57279593715));
#24708=CARTESIAN_POINT('Ctrl Pts',(-0.47119721649,1.065892903769,-30.61179593715));
#24709=CARTESIAN_POINT('Ctrl Pts',(-0.1981104409423,1.114438723627,-30.63129593715));
#24710=CARTESIAN_POINT('Ctrl Pts',(1.254220581577,0.1744837446815,-28.83688532136));
#24711=CARTESIAN_POINT('Ctrl Pts',(1.296976815913,-0.1328557681934,-28.85638532136));
#24712=CARTESIAN_POINT('Ctrl Pts',(1.145950536365,-0.7785637255274,-28.89538532136));
#24713=CARTESIAN_POINT('Ctrl Pts',(0.3276970697449,-1.346337938953,-28.95388532136));
#24714=CARTESIAN_POINT('Ctrl Pts',(-0.6598677698274,-1.218343850632,-29.01238532136));
#24715=CARTESIAN_POINT('Ctrl Pts',(-1.306586531957,-0.461152275356,-29.07088532136));
#24716=CARTESIAN_POINT('Ctrl Pts',(-1.278435472814,0.5342580719014,-29.12938532136));
#24717=CARTESIAN_POINT('Ctrl Pts',(-0.5899504854742,1.253708358346,-29.18788532136));
#24718=CARTESIAN_POINT('Ctrl Pts',(0.403253374937,1.32559951767,-29.24638532136));
#24719=CARTESIAN_POINT('Ctrl Pts',(1.188170301526,0.712796213176,-29.30488532136));
#24720=CARTESIAN_POINT('Ctrl Pts',(1.359377697933,-0.2681779299465,-29.36338532136));
#24721=CARTESIAN_POINT('Ctrl Pts',(0.8284441504486,-1.11063379547,-29.42188532136));
#24722=CARTESIAN_POINT('Ctrl Pts',(-0.1303944337356,-1.37942902105,-29.48038532136));
#24723=CARTESIAN_POINT('Ctrl Pts',(-1.021882146958,-0.9357264619928,-29.53888532136));
#24724=CARTESIAN_POINT('Ctrl Pts',(-1.38555091679,-0.008705787692765,-29.59738532136));
#24725=CARTESIAN_POINT('Ctrl Pts',(-1.033559839496,0.9228115690148,-29.65588532136));
#24726=CARTESIAN_POINT('Ctrl Pts',(-0.1477180983746,1.377681565952,-29.71438532136));
#24727=CARTESIAN_POINT('Ctrl Pts',(0.8144224711886,1.120956364969,-29.77288532136));
#24728=CARTESIAN_POINT('Ctrl Pts',(1.355900433453,0.2852387566824,-29.83138532136));
#24729=CARTESIAN_POINT('Ctrl Pts',(1.197033511132,-0.6978093629019,-29.88988532136));
#24730=CARTESIAN_POINT('Ctrl Pts',(0.4198790837453,-1.320427464418,-29.94838532136));
#24731=CARTESIAN_POINT('Ctrl Pts',(-0.5741497994896,-1.261023053592,-30.00688532136));
#24732=CARTESIAN_POINT('Ctrl Pts',(-1.27162086324,-0.5502794859312,-30.06538532136));
#24733=CARTESIAN_POINT('Ctrl Pts',(-1.312278829779,0.4446924903434,-30.12388532136));
#24734=CARTESIAN_POINT('Ctrl Pts',(-0.6751231782377,1.209973479856,-30.18238532136));
#24735=CARTESIAN_POINT('Ctrl Pts',(0.3107446679484,1.350283251132,-30.24088532136));
#24736=CARTESIAN_POINT('Ctrl Pts',(1.136107913383,0.793149528647,-30.29938532136));
#24737=CARTESIAN_POINT('Ctrl Pts',(1.37465222959,-0.1736590647829,-30.35788532136));
#24738=CARTESIAN_POINT('Ctrl Pts',(0.9031679079763,-1.050769563483,-30.41638532136));
#24739=CARTESIAN_POINT('Ctrl Pts',(-0.03482443348539,-1.385141525401,-30.47488532136));
#24740=CARTESIAN_POINT('Ctrl Pts',(-0.9548035033152,-1.004060497225,-30.53338532136));
#24741=CARTESIAN_POINT('Ctrl Pts',(-1.381707433535,-0.1043828697565,-30.59188532136));
#24742=CARTESIAN_POINT('Ctrl Pts',(-1.094576294964,0.8492743025702,-30.65038532136));
#24743=CARTESIAN_POINT('Ctrl Pts',(-0.527141221495,1.192443562085,-30.68938532136));
#24744=CARTESIAN_POINT('Ctrl Pts',(-0.2216315720351,1.246753099329,-30.70888532136));
#24745=CARTESIAN_POINT('Ctrl Pts',(1.387327460022,0.193001210377,-28.91447470556));
#24746=CARTESIAN_POINT('Ctrl Pts',(1.434621292425,-0.1469553746322,-28.93397470556));
#24747=CARTESIAN_POINT('Ctrl Pts',(1.267567021527,-0.8611904888719,-28.97297470556));
#24748=CARTESIAN_POINT('Ctrl Pts',(0.3624746317385,-1.489220971666,-29.03147470556));
#24749=CARTESIAN_POINT('Ctrl Pts',(-0.7298976675334,-1.347643233224,-29.08997470556));
#24750=CARTESIAN_POINT('Ctrl Pts',(-1.445250860419,-0.510093060384,-29.14847470556));
#24751=CARTESIAN_POINT('Ctrl Pts',(-1.414112209091,0.5909573680856,-29.20697470556));
#24752=CARTESIAN_POINT('Ctrl Pts',(-0.6525602597933,1.386760875991,-29.26547470556));
#24753=CARTESIAN_POINT('Ctrl Pts',(0.4460495136298,1.466281640462,-29.32397470556));
#24754=CARTESIAN_POINT('Ctrl Pts',(1.3142674508,0.7884432566843,-29.38247470556));
#24755=CARTESIAN_POINT('Ctrl Pts',(1.503644603339,-0.296638894188,-29.44097470556));
#24756=CARTESIAN_POINT('Ctrl Pts',(0.9163645820317,-1.228502214935,-29.49947470556));
#24757=CARTESIAN_POINT('Ctrl Pts',(-0.1442328257188,-1.525823916594,-29.55797470556));
#24758=CARTESIAN_POINT('Ctrl Pts',(-1.130331605306,-1.035032461483,-29.61647470556));
#24759=CARTESIAN_POINT('Ctrl Pts',(-1.532595511792,-0.009629708286331,-29.67497470556));
#24760=CARTESIAN_POINT('Ctrl Pts',(-1.143248618282,1.020746947487,-29.73347470556));
#24761=CARTESIAN_POINT('Ctrl Pts',(-0.1633950018263,1.523891009035,-29.79197470556));
#24762=CARTESIAN_POINT('Ctrl Pts',(0.9008548216604,1.239920289503,-29.85047470556));
#24763=CARTESIAN_POINT('Ctrl Pts',(1.499798306627,0.3155103381501,-29.90897470556));
#24764=CARTESIAN_POINT('Ctrl Pts',(1.324071287741,-0.7718658944325,-29.96747470556));
#24765=CARTESIAN_POINT('Ctrl Pts',(0.4644396618308,-1.460560691846,-30.02597470556));
#24766=CARTESIAN_POINT('Ctrl Pts',(-0.6350826917518,-1.394851859129,-30.08447470556));
#24767=CARTESIAN_POINT('Ctrl Pts',(-1.406574384301,-0.6086790894146,-30.14297470556));
#24768=CARTESIAN_POINT('Ctrl Pts',(-1.451547265688,0.4918864450011,-30.20147470556));
#24769=CARTESIAN_POINT('Ctrl Pts',(-0.7467720892358,1.3383845387,-30.25997470556));
#24770=CARTESIAN_POINT('Ctrl Pts',(0.3437231195475,1.493584988654,-30.31847470556));
#24771=CARTESIAN_POINT('Ctrl Pts',(1.256679828841,0.8773242419706,-30.37697470556));
#24772=CARTESIAN_POINT('Ctrl Pts',(1.520540177784,-0.1920890095362,-30.43547470556));
#24773=CARTESIAN_POINT('Ctrl Pts',(0.9990185603327,-1.162284761539,-30.49397470556));
#24774=CARTESIAN_POINT('Ctrl Pts',(-0.03852025199049,-1.532142672854,-30.55247470556));
#24775=CARTESIAN_POINT('Ctrl Pts',(-1.056134095176,-1.110618594357,-30.61097470556));
#24776=CARTESIAN_POINT('Ctrl Pts',(-1.528344130543,-0.1154607281177,-30.66947470556));
#24777=CARTESIAN_POINT('Ctrl Pts',(-1.210740577374,0.9394053792083,-30.72797470556));
#24778=CARTESIAN_POINT('Ctrl Pts',(-0.5830852265001,1.318994220401,-30.76697470556));
#24779=CARTESIAN_POINT('Ctrl Pts',(-0.2451527031279,1.379067475031,-30.78647470556));
#24780=CARTESIAN_POINT('Ctrl Pts',(1.520434338468,0.2115186760726,-28.99206408977));
#24781=CARTESIAN_POINT('Ctrl Pts',(1.572265768938,-0.161054981071,-29.01156408977));
#24782=CARTESIAN_POINT('Ctrl Pts',(1.389183506688,-0.9438172522165,-29.05056408977));
#24783=CARTESIAN_POINT('Ctrl Pts',(0.3972521937322,-1.632104004379,-29.10906408977));
#24784=CARTESIAN_POINT('Ctrl Pts',(-0.7999275652393,-1.476942615815,-29.16756408977));
#24785=CARTESIAN_POINT('Ctrl Pts',(-1.583915188882,-0.559033845412,-29.22606408977));
#24786=CARTESIAN_POINT('Ctrl Pts',(-1.549788945368,0.6476566642697,-29.28456408977));
#24787=CARTESIAN_POINT('Ctrl Pts',(-0.7151700341124,1.519813393635,-29.34306408977));
#24788=CARTESIAN_POINT('Ctrl Pts',(0.4888456523225,1.606963763254,-29.40156408977));
#24789=CARTESIAN_POINT('Ctrl Pts',(1.440364600074,0.8640903001927,-29.46006408977));
#24790=CARTESIAN_POINT('Ctrl Pts',(1.647911508744,-0.3250998584294,-29.51856408977));
#24791=CARTESIAN_POINT('Ctrl Pts',(1.004285013615,-1.3463706344,-29.57706408977));
#24792=CARTESIAN_POINT('Ctrl Pts',(-0.1580712177019,-1.672218812138,-29.63556408977));
#24793=CARTESIAN_POINT('Ctrl Pts',(-1.238781063654,-1.134338460973,-29.69406408977));
#24794=CARTESIAN_POINT('Ctrl Pts',(-1.679640106794,-0.0105536288799,-29.75256408977));
#24795=CARTESIAN_POINT('Ctrl Pts',(-1.252937397068,1.11868232596,-29.81106408977));
#24796=CARTESIAN_POINT('Ctrl Pts',(-0.179071905278,1.670100452118,-29.86956408977));
#24797=CARTESIAN_POINT('Ctrl Pts',(0.9872871721321,1.358884214036,-29.92806408977));
#24798=CARTESIAN_POINT('Ctrl Pts',(1.643696179801,0.3457819196178,-29.98656408977));
#24799=CARTESIAN_POINT('Ctrl Pts',(1.451109064351,-0.8459224259632,-30.04506408977));
#24800=CARTESIAN_POINT('Ctrl Pts',(0.5090002399164,-1.600693919274,-30.10356408977));
#24801=CARTESIAN_POINT('Ctrl Pts',(-0.6960155840139,-1.528680664665,-30.16206408977));
#24802=CARTESIAN_POINT('Ctrl Pts',(-1.541527905363,-0.6670786928981,-30.22056408977));
#24803=CARTESIAN_POINT('Ctrl Pts',(-1.590815701598,0.5390803996589,-30.27906408977));
#24804=CARTESIAN_POINT('Ctrl Pts',(-0.818421000234,1.466795597545,-30.33756408977));
#24805=CARTESIAN_POINT('Ctrl Pts',(0.3767015711466,1.636886726176,-30.39606408977));
#24806=CARTESIAN_POINT('Ctrl Pts',(1.377251744299,0.9614989552941,-30.45456408977));
#24807=CARTESIAN_POINT('Ctrl Pts',(1.666428125978,-0.2105189542896,-30.51306408977));
#24808=CARTESIAN_POINT('Ctrl Pts',(1.094869212689,-1.273799959595,-30.57156408977));
#24809=CARTESIAN_POINT('Ctrl Pts',(-0.0422160704956,-1.679143820308,-30.63006408977));
#24810=CARTESIAN_POINT('Ctrl Pts',(-1.157464687037,-1.217176691488,-30.68856408977));
#24811=CARTESIAN_POINT('Ctrl Pts',(-1.674980827552,-0.126538586479,-30.74706408977));
#24812=CARTESIAN_POINT('Ctrl Pts',(-1.326904859784,1.029536455846,-30.80556408977));
#24813=CARTESIAN_POINT('Ctrl Pts',(-0.6390292315051,1.445544878716,-30.84456408977));
#24814=CARTESIAN_POINT('Ctrl Pts',(-0.2686738342207,1.511381850733,-30.86406408977));
#24815=CARTESIAN_POINT('Ctrl Pts',(1.42593782207375,-0.463290149673499,
-29.0080029164203));
#24816=CARTESIAN_POINT('Ctrl Pts',(1.4000955218869,-0.542653335440824,-29.0123014375039));
#24817=CARTESIAN_POINT('Ctrl Pts',(1.36765200184006,-0.619868124763615,
-29.0165388034481));
#24818=CARTESIAN_POINT('Ctrl Pts',(1.29873520723083,-0.752009101820746,
-29.0242292609336));
#24819=CARTESIAN_POINT('Ctrl Pts',(1.26459120876806,-0.808214901017139,
-29.0276605707244));
#24820=CARTESIAN_POINT('Ctrl Pts',(1.17296738697668,-0.93860426373619,-29.036227725297));
#24821=CARTESIAN_POINT('Ctrl Pts',(1.11190361127669,-1.01012236415906,-29.0414340737163));
#24822=CARTESIAN_POINT('Ctrl Pts',(1.00102607386565,-1.11785813869305,-29.049956093286));
#24823=CARTESIAN_POINT('Ctrl Pts',(0.95469123817742,-1.15770678670362,-29.0532986472221));
#24824=CARTESIAN_POINT('Ctrl Pts',(0.810813094380322,-1.26679388253448,
-29.0629595926022));
#24825=CARTESIAN_POINT('Ctrl Pts',(0.70691663902075,-1.32739491843066,-29.0690181195741));
#24826=CARTESIAN_POINT('Ctrl Pts',(0.534047586467599,-1.40258022987199,
-29.0786488439575));
#24827=CARTESIAN_POINT('Ctrl Pts',(0.468714984262451,-1.42581466419004,
-29.0821999292582));
#24828=CARTESIAN_POINT('Ctrl Pts',(0.290798924709339,-1.4754685423226,-29.0919233537941));
#24829=CARTESIAN_POINT('Ctrl Pts',(0.176323319900497,-1.49336271384772,
-29.0983060249261));
#24830=CARTESIAN_POINT('Ctrl Pts',(-0.0011232688530839,-1.50067293458033,
-29.1080926796056));
#24831=CARTESIAN_POINT('Ctrl Pts',(-0.0639686211733561,-1.49933192056413,
-29.1115332629733));
#24832=CARTESIAN_POINT('Ctrl Pts',(-0.243291143340492,-1.4841146140882,
-29.1211707508265));
#24833=CARTESIAN_POINT('Ctrl Pts',(-0.358745366957707,-1.46033381204158,
-29.1271252317688));
#24834=CARTESIAN_POINT('Ctrl Pts',(-0.537227030820788,-1.40146808975044,
-29.1367339290109));
#24835=CARTESIAN_POINT('Ctrl Pts',(-0.603061083869039,-1.37449094299913,
-29.1403766948368));
#24836=CARTESIAN_POINT('Ctrl Pts',(-0.771966740133044,-1.29077131310097,
-29.1502995717576));
#24837=CARTESIAN_POINT('Ctrl Pts',(-0.870613016983697,-1.22624541954956,
-29.1567947691127));
#24838=CARTESIAN_POINT('Ctrl Pts',(-1.00821324287481,-1.11150228748402,
-29.1666683908791));
#24839=CARTESIAN_POINT('Ctrl Pts',(-1.05360404238008,-1.0686051413095,-29.1700860631929));
#24840=CARTESIAN_POINT('Ctrl Pts',(-1.17654781894306,-0.936825581166674,
-29.1797352518379));
#24841=CARTESIAN_POINT('Ctrl Pts',(-1.24654830775745,-0.841141577531135,
-29.1857194157032));
#24842=CARTESIAN_POINT('Ctrl Pts',(-1.33928860282852,-0.677463839254871,
-29.1953359409272));
#24843=CARTESIAN_POINT('Ctrl Pts',(-1.36974740351839,-0.613701793509182,
-29.1989543208077));
#24844=CARTESIAN_POINT('Ctrl Pts',(-1.43846410791663,-0.4390499407593,-29.2088339443768));
#24845=CARTESIAN_POINT('Ctrl Pts',(-1.46823431736669,-0.325357653795937,
-29.2153100443318));
#24846=CARTESIAN_POINT('Ctrl Pts',(-1.49330306011693,-0.148275815140815,
-29.2251662171994));
#24847=CARTESIAN_POINT('Ctrl Pts',(-1.49820320931145,-0.0859865051388653,
-29.228585503324));
#24848=CARTESIAN_POINT('Ctrl Pts',(-1.5010074205354,0.0941459644453279,
-29.2382311308569));
#24849=CARTESIAN_POINT('Ctrl Pts',(-1.48877467195723,0.211968912555517,
-29.2442108556331));
#24850=CARTESIAN_POINT('Ctrl Pts',(-1.4478272251766,0.395544928525086,-29.2538255812004));
#24851=CARTESIAN_POINT('Ctrl Pts',(-1.42764604026499,0.463327876329372,
-29.25744694048));
#24852=CARTESIAN_POINT('Ctrl Pts',(-1.36146963093795,0.639017431313202,
-29.2673293247307));
#24853=CARTESIAN_POINT('Ctrl Pts',(-1.30730802162139,0.743313376844862,
-29.2738049665947));
#24854=CARTESIAN_POINT('Ctrl Pts',(-1.20713841752504,0.891492870058028,
-29.2836618170511));
#24855=CARTESIAN_POINT('Ctrl Pts',(-1.16898821411711,0.940997459424659,
-29.2870820680485));
#24856=CARTESIAN_POINT('Ctrl Pts',(-1.05025484597231,1.07649922644131,-29.2967281671057));
#24857=CARTESIAN_POINT('Ctrl Pts',(-0.962169757854717,1.15568550758944,
-29.3027074683553));
#24858=CARTESIAN_POINT('Ctrl Pts',(-0.808680084431039,1.26439632004502,
-29.312322294698));
#24859=CARTESIAN_POINT('Ctrl Pts',(-0.748241673711729,1.30114647916462,
-29.3159442290259));
#24860=CARTESIAN_POINT('Ctrl Pts',(-0.581290337223563,1.38710162391503,
-29.3258287276009));
#24861=CARTESIAN_POINT('Ctrl Pts',(-0.471139424218073,1.42814660880992,
-29.3323060308231));
#24862=CARTESIAN_POINT('Ctrl Pts',(-0.297438103245898,1.47087436946332,
-29.3421639285785));
#24863=CARTESIAN_POINT('Ctrl Pts',(-0.235947676930806,1.48200420050721,
-29.3455836417905));
#24864=CARTESIAN_POINT('Ctrl Pts',(-0.0570020925865009,1.50287634541186,
-29.3552295209647));
#24865=CARTESIAN_POINT('Ctrl Pts',(0.0614499559187976,1.50253268545666,
-29.3612090870096));
#24866=CARTESIAN_POINT('Ctrl Pts',(0.24820953664258,1.48022037915887,-29.3708238543927));
#24867=CARTESIAN_POINT('Ctrl Pts',(0.317679980760958,1.4669444814521,-29.3744454300582));
#24868=CARTESIAN_POINT('Ctrl Pts',(0.499154349324895,1.41872967225326,-29.3843294368258));
#24869=CARTESIAN_POINT('Ctrl Pts',(0.608383825636182,1.37529774561873,-29.3908066217182));
#24870=CARTESIAN_POINT('Ctrl Pts',(0.765879412679508,1.29049204594782,-29.4006643606365));
#24871=CARTESIAN_POINT('Ctrl Pts',(0.818953429590234,1.25750673778986,-29.4040840410556));
#24872=CARTESIAN_POINT('Ctrl Pts',(0.965663498578195,1.15298535586764,-29.4137286274331));
#24873=CARTESIAN_POINT('Ctrl Pts',(1.05327773123505,1.07330395093089,-29.4197070779835));
#24874=CARTESIAN_POINT('Ctrl Pts',(1.17683781014979,0.931511944925617,-29.4293211698108));
#24875=CARTESIAN_POINT('Ctrl Pts',(1.21947089419789,0.875065016530118,-29.432943240646));
#24876=CARTESIAN_POINT('Ctrl Pts',(1.32177199388042,0.717549504139619,-29.4428298530652));
#24877=CARTESIAN_POINT('Ctrl Pts',(1.37367890501952,0.612037813295693,-29.44930934989));
#24878=CARTESIAN_POINT('Ctrl Pts',(1.43362095888831,0.443475239829729,-29.4591685104264));
#24879=CARTESIAN_POINT('Ctrl Pts',(1.45085892857129,0.3834248374722,-29.4625874127304));
#24880=CARTESIAN_POINT('Ctrl Pts',(1.48955047484412,0.207602469875726,-29.4722262250227));
#24881=CARTESIAN_POINT('Ctrl Pts',(1.50109445264084,0.0898315631773016,
-29.4782002269599));
#24882=CARTESIAN_POINT('Ctrl Pts',(1.49767544684285,-0.0981555915514404,
-29.4878113535259));
#24883=CARTESIAN_POINT('Ctrl Pts',(1.49144511132647,-0.168653636923899,
-29.4914350984059));
#24884=CARTESIAN_POINT('Ctrl Pts',(1.46166396955629,-0.354315276620493,
-29.5013327052724));
#24885=CARTESIAN_POINT('Ctrl Pts',(1.42933928187306,-0.4675621445785,-29.5078224540884));
#24886=CARTESIAN_POINT('Ctrl Pts',(1.3606586283959,-0.632882317148081,-29.5176877742471));
#24887=CARTESIAN_POINT('Ctrl Pts',(1.33318501212234,-0.688924104651172,
-29.5211031065141));
#24888=CARTESIAN_POINT('Ctrl Pts',(1.24418462634253,-0.844844025520772,
-29.5307147857776));
#24889=CARTESIAN_POINT('Ctrl Pts',(1.17404956835561,-0.939607737096756,
-29.5366678050766));
#24890=CARTESIAN_POINT('Ctrl Pts',(1.04571137208454,-1.07665016627595,-29.546265015286));
#24891=CARTESIAN_POINT('Ctrl Pts',(0.993712342102203,-1.12490439718285,
-29.5498967185494));
#24892=CARTESIAN_POINT('Ctrl Pts',(0.846363214782337,-1.24333002925605,
-29.5598459409067));
#24893=CARTESIAN_POINT('Ctrl Pts',(0.745683333010676,-1.30605320820971,
-29.5663837258148));
#24894=CARTESIAN_POINT('Ctrl Pts',(0.583272603705027,-1.38263899253368,
-29.5762779547346));
#24895=CARTESIAN_POINT('Ctrl Pts',(0.525552156721495,-1.40561680906026,
-29.5796766498336));
#24896=CARTESIAN_POINT('Ctrl Pts',(0.357140973166551,-1.46072903308538,
-29.5891607967467));
#24897=CARTESIAN_POINT('Ctrl Pts',(0.243627541970809,-1.48372465370254,
-29.5950149192744));
#24898=CARTESIAN_POINT('Ctrl Pts',(0.0578093582639404,-1.49981650319702,
-29.6045471525713));
#24899=CARTESIAN_POINT('Ctrl Pts',(-0.0139122887500927,-1.50092767768368,
-29.6082167101067));
#24900=CARTESIAN_POINT('Ctrl Pts',(-0.207419868633202,-1.49001433957701,
-29.6184109075986));
#24901=CARTESIAN_POINT('Ctrl Pts',(-0.32808953137425,-1.46803030233152,
-29.6251771153634));
#24902=CARTESIAN_POINT('Ctrl Pts',(-0.502081418207972,-1.41409095323784,
-29.6352089803415));
#24903=CARTESIAN_POINT('Ctrl Pts',(-0.55894291523991,-1.39261798704368,
-29.6385298514441));
#24904=CARTESIAN_POINT('Ctrl Pts',(-0.709589558883048,-1.32491590422671,
-29.6473577240915));
#24905=CARTESIAN_POINT('Ctrl Pts',(-0.80028128622474,-1.27203083155135,
-29.6526918901923));
#24906=CARTESIAN_POINT('Ctrl Pts',(-0.970678122639343,-1.14751854395336,
-29.663472590764));
#24907=CARTESIAN_POINT('Ctrl Pts',(-1.05026685851864,-1.07537692391356,
-29.6689386958154));
#24908=CARTESIAN_POINT('Ctrl Pts',(-1.16364069583314,-0.947688958144565,
-29.6781017466052));
#24909=CARTESIAN_POINT('Ctrl Pts',(-1.20288749268217,-0.897310890384465,
-29.6816027079286));
#24910=CARTESIAN_POINT('Ctrl Pts',(-1.30485094509196,-0.747746430700471,
-29.6915841548083));
#24911=CARTESIAN_POINT('Ctrl Pts',(-1.35969032092745,-0.642944917584904,
-29.698081098428));
#24912=CARTESIAN_POINT('Ctrl Pts',(-1.42743368712507,-0.464312075170907,
-29.7081027051918));
#24913=CARTESIAN_POINT('Ctrl Pts',(-1.44831173355896,-0.394167874022602,
-29.7118384577069));
#24914=CARTESIAN_POINT('Ctrl Pts',(-1.48860958462676,-0.211378996370762,
-29.7214010962492));
#24915=CARTESIAN_POINT('Ctrl Pts',(-1.5005971977563,-0.0969130400351905,
-29.727236335208));
#24916=CARTESIAN_POINT('Ctrl Pts',(-1.49850151240142,0.082424701531096,
-29.7368697375097));
#24917=CARTESIAN_POINT('Ctrl Pts',(-1.49351601330572,0.14710677398852,-29.7404292575701));
#24918=CARTESIAN_POINT('Ctrl Pts',(-1.46828906970983,0.324341670760753,
-29.7503031910294));
#24919=CARTESIAN_POINT('Ctrl Pts',(-1.43925965497355,0.435838974217578,
-29.7566274304292));
#24920=CARTESIAN_POINT('Ctrl Pts',(-1.37126409426303,0.610499512478932,
-29.7664638324321));
#24921=CARTESIAN_POINT('Ctrl Pts',(-1.3400864136786,0.676065726814819,-29.770171673663));
#24922=CARTESIAN_POINT('Ctrl Pts',(-1.24731552899021,0.839758478885043,
-29.7797847505764));
#24923=CARTESIAN_POINT('Ctrl Pts',(-1.1785941035599,0.934058007629023,-29.785696171446));
#24924=CARTESIAN_POINT('Ctrl Pts',(-1.05546483765357,1.06692218661126,-29.7954280112206));
#24925=CARTESIAN_POINT('Ctrl Pts',(-1.00818706494207,1.11167326541079,-29.7990005193374));
#24926=CARTESIAN_POINT('Ctrl Pts',(-0.870823071904622,1.22580137835212,
-29.8088510704562));
#24927=CARTESIAN_POINT('Ctrl Pts',(-0.775048385234494,1.28863138475216,
-29.8151376173598));
#24928=CARTESIAN_POINT('Ctrl Pts',(-0.608201585969179,1.372278790715,-29.8249336332071));
#24929=CARTESIAN_POINT('Ctrl Pts',(-0.541229418304693,1.39998227251173,
-29.8286354732767));
#24930=CARTESIAN_POINT('Ctrl Pts',(-0.362461907410498,1.45934520329591,
-29.8382595610624));
#24931=CARTESIAN_POINT('Ctrl Pts',(-0.247910310152804,1.48329652730199,
-29.8441874915178));
#24932=CARTESIAN_POINT('Ctrl Pts',(-0.067079679465184,1.49927833357457,
-29.8539407146482));
#24933=CARTESIAN_POINT('Ctrl Pts',(-0.00194837874329868,1.50075347353078,
-29.8575160674771));
#24934=CARTESIAN_POINT('Ctrl Pts',(0.176388759810885,1.49324364664456,-29.8673615289051));
#24935=CARTESIAN_POINT('Ctrl Pts',(0.289422272377968,1.47562607794796,-29.8736398585918));
#24936=CARTESIAN_POINT('Ctrl Pts',(0.469118635181389,1.42582691494393,-29.8834270879709));
#24937=CARTESIAN_POINT('Ctrl Pts',(0.537351848546642,1.40147387957845,-29.8871276392637));
#24938=CARTESIAN_POINT('Ctrl Pts',(0.709816341005259,1.32561097995918,-29.896754122299));
#24939=CARTESIAN_POINT('Ctrl Pts',(0.810915190645302,1.26651567965261,-29.9026856271651));
#24940=CARTESIAN_POINT('Ctrl Pts',(0.955828205322697,1.15703460075147,-29.9124434958545));
#24941=CARTESIAN_POINT('Ctrl Pts',(1.00513484970065,1.11443713551617,-29.9160194809169));
#24942=CARTESIAN_POINT('Ctrl Pts',(1.13235626326785,0.989268123702891,-29.9258637314856));
#24943=CARTESIAN_POINT('Ctrl Pts',(1.20435935345013,0.900415694635981,-29.9321401581186));
#24944=CARTESIAN_POINT('Ctrl Pts',(1.30422842122028,0.742995114867555,-29.9419252301247));
#24945=CARTESIAN_POINT('Ctrl Pts',(1.33850428637846,0.679176789630696,-29.9456253690681));
#24946=CARTESIAN_POINT('Ctrl Pts',(1.41555872677202,0.507229225985164,-29.9552524128281));
#24947=CARTESIAN_POINT('Ctrl Pts',(1.45092135482842,0.395571776845064,-29.9611848560455));
#24948=CARTESIAN_POINT('Ctrl Pts',(1.48498494282667,0.217154597218618,-29.9709437897809));
#24949=CARTESIAN_POINT('Ctrl Pts',(1.49298796863473,0.152489011855701,-29.974519777317));
#24950=CARTESIAN_POINT('Ctrl Pts',(1.50340388108982,-0.0256836768169241,
-29.9843642610041));
#24951=CARTESIAN_POINT('Ctrl Pts',(1.49721842404337,-0.139884647900195,
-29.9906409088091));
#24952=CARTESIAN_POINT('Ctrl Pts',(1.46571162513833,-0.323642057804169,
-30.0004266086903));
#24953=CARTESIAN_POINT('Ctrl Pts',(1.44833022129799,-0.393974312375014,
-30.0041271460791));
#24954=CARTESIAN_POINT('Ctrl Pts',(1.39015726367332,-0.573192420094281,
-30.0137542167653));
#24955=CARTESIAN_POINT('Ctrl Pts',(1.34150154456984,-0.679722243649215,
-30.0196863198532));
#24956=CARTESIAN_POINT('Ctrl Pts',(1.24710292264637,-0.834908846390197,
-30.0294454373799));
#24957=CARTESIAN_POINT('Ctrl Pts',(1.20966154490511,-0.888249374199367,
-30.0330220191137));
#24958=CARTESIAN_POINT('Ctrl Pts',(1.09789944996753,-1.02737167537288,-30.0428652025311));
#24959=CARTESIAN_POINT('Ctrl Pts',(1.01674273887224,-1.10790672760907,-30.0491399138216));
#24960=CARTESIAN_POINT('Ctrl Pts',(0.870172106627214,-1.22305059251458,
-30.0589230193631));
#24961=CARTESIAN_POINT('Ctrl Pts',(0.810123582582305,-1.26355577891347,
-30.0626227686683));
#24962=CARTESIAN_POINT('Ctrl Pts',(0.646780107007148,-1.35748475497531,
-30.0722498438669));
#24963=CARTESIAN_POINT('Ctrl Pts',(0.539228676745347,-1.40388162608679,
-30.0781826801763));
#24964=CARTESIAN_POINT('Ctrl Pts',(0.365135729805777,-1.45568214313488,
-30.087941389622));
#24965=CARTESIAN_POINT('Ctrl Pts',(0.301612243337302,-1.47013413365298,
-30.0915167022075));
#24966=CARTESIAN_POINT('Ctrl Pts',(0.125404811940233,-1.49838413751754,
-30.1013601563619));
#24967=CARTESIAN_POINT('Ctrl Pts',(0.0111666855167293,-1.5036970131519,
-30.1076365696618));
#24968=CARTESIAN_POINT('Ctrl Pts',(-0.174761510899895,-1.49080673748828,
-30.1174189322172));
#24969=CARTESIAN_POINT('Ctrl Pts',(-0.246427172421646,-1.48058802757682,
-30.121116554073));
#24970=CARTESIAN_POINT('Ctrl Pts',(-0.430616825462687,-1.44071973987913,
-30.1307449705376));
#24971=CARTESIAN_POINT('Ctrl Pts',(-0.541581250336894,-1.40298076176452,
-30.136681085897));
#24972=CARTESIAN_POINT('Ctrl Pts',(-0.705506188167064,-1.32460903371917,
-30.1464428705794));
#24973=CARTESIAN_POINT('Ctrl Pts',(-0.762304362372859,-1.29272947476832,
-30.1500173873045));
#24974=CARTESIAN_POINT('Ctrl Pts',(-0.912190026328416,-1.19534674499311,
-30.1598766760129));
#24975=CARTESIAN_POINT('Ctrl Pts',(-1.00069915444838,-1.12245120893206,
-30.1661693592564));
#24976=CARTESIAN_POINT('Ctrl Pts',(-1.13040187285673,-0.987575625605336,
-30.1759907241941));
#24977=CARTESIAN_POINT('Ctrl Pts',(-1.17693432414073,-0.931539330981527,
-30.1797110156791));
#24978=CARTESIAN_POINT('Ctrl Pts',(-1.28648958818024,-0.778417630040102,
-30.1893325848552));
#24979=CARTESIAN_POINT('Ctrl Pts',(-1.34309105930442,-0.676508040664117,
-30.1952410176057));
#24980=CARTESIAN_POINT('Ctrl Pts',(-1.41199275451509,-0.508621610801896,
-30.2049927331912));
#24981=CARTESIAN_POINT('Ctrl Pts',(-1.43282829831979,-0.446487595443442,
-30.2085898220565));
#24982=CARTESIAN_POINT('Ctrl Pts',(-1.47808823425589,-0.275266401610107,
-30.2183572238959));
#24983=CARTESIAN_POINT('Ctrl Pts',(-1.49465028229549,-0.163896298659272,
-30.2245351401014));
#24984=CARTESIAN_POINT('Ctrl Pts',(-1.50082013332007,0.0192063609786526,
-30.2341515058503));
#24985=CARTESIAN_POINT('Ctrl Pts',(-1.4981684423692,0.0901325390511118,
-30.2377773150278));
#24986=CARTESIAN_POINT('Ctrl Pts',(-1.47789558605186,0.277967822606107,
-30.2474232896606));
#24987=CARTESIAN_POINT('Ctrl Pts',(-1.45143412726189,0.394110560301101,
-30.2534426410668));
#24988=CARTESIAN_POINT('Ctrl Pts',(-1.39004475838229,0.565507974979767,
-30.2632185229554));
#24989=CARTESIAN_POINT('Ctrl Pts',(-1.36480296677769,0.623917925008732,
-30.2667090528369));
#24990=CARTESIAN_POINT('Ctrl Pts',(-1.29296053725923,0.764960582826655,
-30.2754439929124));
#24991=CARTESIAN_POINT('Ctrl Pts',(-1.24193651414017,0.845397397549996,
-30.2807056397472));
#24992=CARTESIAN_POINT('Ctrl Pts',(-1.11986698073447,1.0023692661947,-30.2913274460477));
#24993=CARTESIAN_POINT('Ctrl Pts',(-1.04738255940246,1.07774802276584,-30.2966469113402));
#24994=CARTESIAN_POINT('Ctrl Pts',(-0.939893368921114,1.16865813938709,
-30.3038489235285));
#24995=CARTESIAN_POINT('Ctrl Pts',(-0.91096944153804,1.19136469798677,-30.3057295679678));
#24996=CARTESIAN_POINT('Ctrl Pts',(-0.88125413572515,1.21298292793906,-30.3076220835796));
#24997=CARTESIAN_POINT('Ctrl Pts',(1.520434338468,0.2115186760726,-28.45156091023));
#24998=CARTESIAN_POINT('Ctrl Pts',(1.572265768938,-0.161054981071,-28.47106091023));
#24999=CARTESIAN_POINT('Ctrl Pts',(1.389183506688,-0.9438172522165,-28.51006091023));
#25000=CARTESIAN_POINT('Ctrl Pts',(0.3972521937322,-1.632104004379,-28.56856091023));
#25001=CARTESIAN_POINT('Ctrl Pts',(-0.7999275652393,-1.476942615815,-28.62706091023));
#25002=CARTESIAN_POINT('Ctrl Pts',(-1.583915188882,-0.559033845412,-28.68556091023));
#25003=CARTESIAN_POINT('Ctrl Pts',(-1.549788945368,0.6476566642697,-28.74406091023));
#25004=CARTESIAN_POINT('Ctrl Pts',(-0.7151700341124,1.519813393635,-28.80256091023));
#25005=CARTESIAN_POINT('Ctrl Pts',(0.4888456523225,1.606963763254,-28.86106091023));
#25006=CARTESIAN_POINT('Ctrl Pts',(1.440364600074,0.8640903001927,-28.91956091023));
#25007=CARTESIAN_POINT('Ctrl Pts',(1.647911508744,-0.3250998584294,-28.97806091023));
#25008=CARTESIAN_POINT('Ctrl Pts',(1.004285013615,-1.3463706344,-29.03656091023));
#25009=CARTESIAN_POINT('Ctrl Pts',(-0.1580712177019,-1.672218812138,-29.09506091023));
#25010=CARTESIAN_POINT('Ctrl Pts',(-1.238781063654,-1.134338460973,-29.15356091023));
#25011=CARTESIAN_POINT('Ctrl Pts',(-1.679640106794,-0.0105536288799,-29.21206091023));
#25012=CARTESIAN_POINT('Ctrl Pts',(-1.252937397068,1.11868232596,-29.27056091023));
#25013=CARTESIAN_POINT('Ctrl Pts',(-0.179071905278,1.670100452118,-29.32906091023));
#25014=CARTESIAN_POINT('Ctrl Pts',(0.9872871721321,1.358884214036,-29.38756091023));
#25015=CARTESIAN_POINT('Ctrl Pts',(1.643696179801,0.3457819196178,-29.44606091023));
#25016=CARTESIAN_POINT('Ctrl Pts',(1.451109064351,-0.8459224259632,-29.50456091023));
#25017=CARTESIAN_POINT('Ctrl Pts',(0.5090002399164,-1.600693919274,-29.56306091023));
#25018=CARTESIAN_POINT('Ctrl Pts',(-0.6960155840139,-1.528680664665,-29.62156091023));
#25019=CARTESIAN_POINT('Ctrl Pts',(-1.541527905363,-0.6670786928981,-29.68006091023));
#25020=CARTESIAN_POINT('Ctrl Pts',(-1.590815701598,0.5390803996589,-29.73856091023));
#25021=CARTESIAN_POINT('Ctrl Pts',(-0.818421000234,1.466795597545,-29.79706091023));
#25022=CARTESIAN_POINT('Ctrl Pts',(0.3767015711466,1.636886726176,-29.85556091023));
#25023=CARTESIAN_POINT('Ctrl Pts',(1.377251744299,0.9614989552941,-29.91406091023));
#25024=CARTESIAN_POINT('Ctrl Pts',(1.666428125978,-0.2105189542896,-29.97256091023));
#25025=CARTESIAN_POINT('Ctrl Pts',(1.094869212689,-1.273799959595,-30.03106091023));
#25026=CARTESIAN_POINT('Ctrl Pts',(-0.0422160704956,-1.679143820308,-30.08956091023));
#25027=CARTESIAN_POINT('Ctrl Pts',(-1.157464687037,-1.217176691488,-30.14806091023));
#25028=CARTESIAN_POINT('Ctrl Pts',(-1.674980827552,-0.126538586479,-30.20656091023));
#25029=CARTESIAN_POINT('Ctrl Pts',(-1.326904859784,1.029536455846,-30.26506091023));
#25030=CARTESIAN_POINT('Ctrl Pts',(-0.6390292315051,1.445544878716,-30.30406091023));
#25031=CARTESIAN_POINT('Ctrl Pts',(-0.2686738342207,1.511381850733,-30.32356091023));
#25032=CARTESIAN_POINT('Ctrl Pts',(1.387327460022,0.193001210377,-28.52915029444));
#25033=CARTESIAN_POINT('Ctrl Pts',(1.434621292425,-0.1469553746322,-28.54865029444));
#25034=CARTESIAN_POINT('Ctrl Pts',(1.267567021527,-0.8611904888719,-28.58765029444));
#25035=CARTESIAN_POINT('Ctrl Pts',(0.3624746317385,-1.489220971666,-28.64615029444));
#25036=CARTESIAN_POINT('Ctrl Pts',(-0.7298976675334,-1.347643233224,-28.70465029444));
#25037=CARTESIAN_POINT('Ctrl Pts',(-1.445250860419,-0.510093060384,-28.76315029444));
#25038=CARTESIAN_POINT('Ctrl Pts',(-1.414112209091,0.5909573680856,-28.82165029444));
#25039=CARTESIAN_POINT('Ctrl Pts',(-0.6525602597933,1.386760875991,-28.88015029444));
#25040=CARTESIAN_POINT('Ctrl Pts',(0.4460495136298,1.466281640462,-28.93865029444));
#25041=CARTESIAN_POINT('Ctrl Pts',(1.3142674508,0.7884432566843,-28.99715029444));
#25042=CARTESIAN_POINT('Ctrl Pts',(1.503644603339,-0.296638894188,-29.05565029444));
#25043=CARTESIAN_POINT('Ctrl Pts',(0.9163645820317,-1.228502214935,-29.11415029444));
#25044=CARTESIAN_POINT('Ctrl Pts',(-0.1442328257188,-1.525823916594,-29.17265029444));
#25045=CARTESIAN_POINT('Ctrl Pts',(-1.130331605306,-1.035032461483,-29.23115029444));
#25046=CARTESIAN_POINT('Ctrl Pts',(-1.532595511792,-0.009629708286331,-29.28965029444));
#25047=CARTESIAN_POINT('Ctrl Pts',(-1.143248618282,1.020746947487,-29.34815029444));
#25048=CARTESIAN_POINT('Ctrl Pts',(-0.1633950018263,1.523891009035,-29.40665029444));
#25049=CARTESIAN_POINT('Ctrl Pts',(0.9008548216604,1.239920289503,-29.46515029444));
#25050=CARTESIAN_POINT('Ctrl Pts',(1.499798306627,0.3155103381501,-29.52365029444));
#25051=CARTESIAN_POINT('Ctrl Pts',(1.324071287741,-0.7718658944325,-29.58215029444));
#25052=CARTESIAN_POINT('Ctrl Pts',(0.4644396618308,-1.460560691846,-29.64065029444));
#25053=CARTESIAN_POINT('Ctrl Pts',(-0.6350826917518,-1.394851859129,-29.69915029444));
#25054=CARTESIAN_POINT('Ctrl Pts',(-1.406574384302,-0.6086790894146,-29.75765029444));
#25055=CARTESIAN_POINT('Ctrl Pts',(-1.451547265688,0.4918864450011,-29.81615029444));
#25056=CARTESIAN_POINT('Ctrl Pts',(-0.7467720892358,1.3383845387,-29.87465029444));
#25057=CARTESIAN_POINT('Ctrl Pts',(0.3437231195475,1.493584988654,-29.93315029444));
#25058=CARTESIAN_POINT('Ctrl Pts',(1.256679828841,0.8773242419706,-29.99165029444));
#25059=CARTESIAN_POINT('Ctrl Pts',(1.520540177784,-0.1920890095362,-30.05015029444));
#25060=CARTESIAN_POINT('Ctrl Pts',(0.9990185603327,-1.162284761539,-30.10865029444));
#25061=CARTESIAN_POINT('Ctrl Pts',(-0.03852025199049,-1.532142672854,-30.16715029444));
#25062=CARTESIAN_POINT('Ctrl Pts',(-1.056134095176,-1.110618594357,-30.22565029444));
#25063=CARTESIAN_POINT('Ctrl Pts',(-1.528344130543,-0.1154607281177,-30.28415029444));
#25064=CARTESIAN_POINT('Ctrl Pts',(-1.210740577374,0.9394053792083,-30.34265029444));
#25065=CARTESIAN_POINT('Ctrl Pts',(-0.5830852265001,1.318994220401,-30.38165029444));
#25066=CARTESIAN_POINT('Ctrl Pts',(-0.2451527031279,1.379067475031,-30.40115029444));
#25067=CARTESIAN_POINT('Ctrl Pts',(1.254220581577,0.1744837446815,-28.60673967864));
#25068=CARTESIAN_POINT('Ctrl Pts',(1.296976815913,-0.1328557681934,-28.62623967864));
#25069=CARTESIAN_POINT('Ctrl Pts',(1.145950536365,-0.7785637255274,-28.66523967864));
#25070=CARTESIAN_POINT('Ctrl Pts',(0.3276970697449,-1.346337938953,-28.72373967864));
#25071=CARTESIAN_POINT('Ctrl Pts',(-0.6598677698274,-1.218343850632,-28.78223967864));
#25072=CARTESIAN_POINT('Ctrl Pts',(-1.306586531957,-0.461152275356,-28.84073967864));
#25073=CARTESIAN_POINT('Ctrl Pts',(-1.278435472814,0.5342580719014,-28.89923967864));
#25074=CARTESIAN_POINT('Ctrl Pts',(-0.5899504854742,1.253708358346,-28.95773967864));
#25075=CARTESIAN_POINT('Ctrl Pts',(0.403253374937,1.32559951767,-29.01623967864));
#25076=CARTESIAN_POINT('Ctrl Pts',(1.188170301526,0.712796213176,-29.07473967864));
#25077=CARTESIAN_POINT('Ctrl Pts',(1.359377697933,-0.2681779299465,-29.13323967864));
#25078=CARTESIAN_POINT('Ctrl Pts',(0.8284441504486,-1.11063379547,-29.19173967864));
#25079=CARTESIAN_POINT('Ctrl Pts',(-0.1303944337356,-1.37942902105,-29.25023967864));
#25080=CARTESIAN_POINT('Ctrl Pts',(-1.021882146958,-0.9357264619928,-29.30873967864));
#25081=CARTESIAN_POINT('Ctrl Pts',(-1.38555091679,-0.008705787692765,-29.36723967864));
#25082=CARTESIAN_POINT('Ctrl Pts',(-1.033559839496,0.9228115690148,-29.42573967864));
#25083=CARTESIAN_POINT('Ctrl Pts',(-0.1477180983746,1.377681565952,-29.48423967864));
#25084=CARTESIAN_POINT('Ctrl Pts',(0.8144224711886,1.120956364969,-29.54273967864));
#25085=CARTESIAN_POINT('Ctrl Pts',(1.355900433453,0.2852387566824,-29.60123967864));
#25086=CARTESIAN_POINT('Ctrl Pts',(1.197033511132,-0.6978093629019,-29.65973967864));
#25087=CARTESIAN_POINT('Ctrl Pts',(0.4198790837453,-1.320427464418,-29.71823967864));
#25088=CARTESIAN_POINT('Ctrl Pts',(-0.5741497994896,-1.261023053592,-29.77673967864));
#25089=CARTESIAN_POINT('Ctrl Pts',(-1.27162086324,-0.5502794859312,-29.83523967864));
#25090=CARTESIAN_POINT('Ctrl Pts',(-1.312278829779,0.4446924903434,-29.89373967864));
#25091=CARTESIAN_POINT('Ctrl Pts',(-0.6751231782377,1.209973479856,-29.95223967864));
#25092=CARTESIAN_POINT('Ctrl Pts',(0.3107446679484,1.350283251132,-30.01073967864));
#25093=CARTESIAN_POINT('Ctrl Pts',(1.136107913383,0.793149528647,-30.06923967864));
#25094=CARTESIAN_POINT('Ctrl Pts',(1.37465222959,-0.1736590647829,-30.12773967864));
#25095=CARTESIAN_POINT('Ctrl Pts',(0.9031679079763,-1.050769563483,-30.18623967864));
#25096=CARTESIAN_POINT('Ctrl Pts',(-0.03482443348539,-1.385141525401,-30.24473967864));
#25097=CARTESIAN_POINT('Ctrl Pts',(-0.9548035033152,-1.004060497225,-30.30323967864));
#25098=CARTESIAN_POINT('Ctrl Pts',(-1.381707433535,-0.1043828697565,-30.36173967864));
#25099=CARTESIAN_POINT('Ctrl Pts',(-1.094576294964,0.8492743025702,-30.42023967864));
#25100=CARTESIAN_POINT('Ctrl Pts',(-0.527141221495,1.192443562085,-30.45923967864));
#25101=CARTESIAN_POINT('Ctrl Pts',(-0.2216315720351,1.246753099329,-30.47873967864));
#25102=CARTESIAN_POINT('Ctrl Pts',(1.121113703131,0.1559662789859,-28.68432906285));
#25103=CARTESIAN_POINT('Ctrl Pts',(1.1593323394,-0.1187561617546,-28.70382906285));
#25104=CARTESIAN_POINT('Ctrl Pts',(1.024334051204,-0.6959369621828,-28.74282906285));
#25105=CARTESIAN_POINT('Ctrl Pts',(0.2929195077513,-1.20345490624,-28.80132906285));
#25106=CARTESIAN_POINT('Ctrl Pts',(-0.5898378721215,-1.089044468041,-28.85982906285));
#25107=CARTESIAN_POINT('Ctrl Pts',(-1.167922203495,-0.4122114903279,-28.91832906285));
#25108=CARTESIAN_POINT('Ctrl Pts',(-1.142758736536,0.4775587757172,-28.97682906285));
#25109=CARTESIAN_POINT('Ctrl Pts',(-0.5273407111551,1.120655840702,-29.03532906285));
#25110=CARTESIAN_POINT('Ctrl Pts',(0.3604572362443,1.184917394878,-29.09382906285));
#25111=CARTESIAN_POINT('Ctrl Pts',(1.062073152252,0.6371491696676,-29.15232906285));
#25112=CARTESIAN_POINT('Ctrl Pts',(1.215110792527,-0.2397169657051,-29.21082906285));
#25113=CARTESIAN_POINT('Ctrl Pts',(0.7405237188655,-0.992765376005,-29.26932906285));
#25114=CARTESIAN_POINT('Ctrl Pts',(-0.1165560417524,-1.233034125506,-29.32782906285));
#25115=CARTESIAN_POINT('Ctrl Pts',(-0.9134326886102,-0.8364204625026,-29.38632906285));
#25116=CARTESIAN_POINT('Ctrl Pts',(-1.238506321788,-0.007781867099199,-29.44482906285));
#25117=CARTESIAN_POINT('Ctrl Pts',(-0.9238710607092,0.8248761905421,-29.50332906285));
#25118=CARTESIAN_POINT('Ctrl Pts',(-0.1320411949229,1.231472122869,-29.56182906285));
#25119=CARTESIAN_POINT('Ctrl Pts',(0.7279901207168,1.001992440436,-29.62032906285));
#25120=CARTESIAN_POINT('Ctrl Pts',(1.212002560279,0.2549671752147,-29.67882906285));
#25121=CARTESIAN_POINT('Ctrl Pts',(1.069995734522,-0.6237528313713,-29.73732906285));
#25122=CARTESIAN_POINT('Ctrl Pts',(0.3753185056597,-1.180294236991,-29.79582906285));
#25123=CARTESIAN_POINT('Ctrl Pts',(-0.5132169072275,-1.127194248056,-29.85432906285));
#25124=CARTESIAN_POINT('Ctrl Pts',(-1.136667342178,-0.4918798824477,-29.91282906285));
#25125=CARTESIAN_POINT('Ctrl Pts',(-1.173010393869,0.3974985356856,-29.97132906285));
#25126=CARTESIAN_POINT('Ctrl Pts',(-0.6034742672396,1.081562421011,-30.02982906285));
#25127=CARTESIAN_POINT('Ctrl Pts',(0.2777662163492,1.206981513611,-30.08832906285));
#25128=CARTESIAN_POINT('Ctrl Pts',(1.015535997925,0.7089748153235,-30.14682906285));
#25129=CARTESIAN_POINT('Ctrl Pts',(1.228764281396,-0.1552291200295,-30.20532906285));
#25130=CARTESIAN_POINT('Ctrl Pts',(0.80731725562,-0.9392543654266,-30.26382906285));
#25131=CARTESIAN_POINT('Ctrl Pts',(-0.03112861498029,-1.238140377948,-30.32232906285));
#25132=CARTESIAN_POINT('Ctrl Pts',(-0.8534729114545,-0.8975024000936,-30.38082906285));
#25133=CARTESIAN_POINT('Ctrl Pts',(-1.235070736526,-0.09330501139524,-30.43932906285));
#25134=CARTESIAN_POINT('Ctrl Pts',(-0.9784120125535,0.7591432259322,-30.49782906285));
#25135=CARTESIAN_POINT('Ctrl Pts',(-0.47119721649,1.065892903769,-30.53682906285));
#25136=CARTESIAN_POINT('Ctrl Pts',(-0.1981104409423,1.114438723627,-30.55632906285));
#25137=CARTESIAN_POINT('Origin',(0.,-1.5,-32.2));
#52138=UNCERTAINTY_MEASURE_WITH_UNIT(LENGTH_MEASURE(0.01),#52165,
'DISTANCE_ACCURACY_VALUE',
'Maximum model space distance between geometric entities at asserted c
onnectivities');
#52149=UNCERTAINTY_MEASURE_WITH_UNIT(LENGTH_MEASURE(0.01),#52165,
'DISTANCE_ACCURACY_VALUE',
'Maximum model space distance between geometric entities at asserted c
onnectivities');
#52153=(
GEOMETRIC_REPRESENTATION_CONTEXT(3)
GLOBAL_UNCERTAINTY_ASSIGNED_CONTEXT((#52138))
GLOBAL_UNIT_ASSIGNED_CONTEXT((#52165,#52167,#52168))
REPRESENTATION_CONTEXT('','3D')
);
#52164=(
GEOMETRIC_REPRESENTATION_CONTEXT(3)
GLOBAL_UNCERTAINTY_ASSIGNED_CONTEXT((#52149))
GLOBAL_UNIT_ASSIGNED_CONTEXT((#52165,#52167,#52168))
REPRESENTATION_CONTEXT('','3D')
);
#52165=(
LENGTH_UNIT()
NAMED_UNIT(*)
SI_UNIT(.MILLI.,.METRE.)
);
#52167=(
NAMED_UNIT(*)
PLANE_ANGLE_UNIT()
SI_UNIT($,.RADIAN.)
);
#52168=(
NAMED_UNIT(*)
SI_UNIT($,.STERADIAN.)
SOLID_ANGLE_UNIT()
);
#52172=SHAPE_DEFINITION_REPRESENTATION(#52186,#52213);
#52186=PRODUCT_DEFINITION_SHAPE('',$,#52228);
#52213=SHAPE_REPRESENTATION('',(#9667),#52153);
#52224=PRODUCT_DEFINITION_CONTEXT('part definition',#52268,'design');
#52228=PRODUCT_DEFINITION('String Post / Peg Shaft',
'String Post / Peg Shaft',#52242,#52224);
#52242=PRODUCT_DEFINITION_FORMATION('',$,#52273);
#52268=APPLICATION_CONTEXT('Managed model based 3d engineering');
#52269=PRODUCT_CONTEXT('part definition',#52268,'mechanical');
#52273=PRODUCT('String Post / Peg Shaft','String Post / Peg Shaft',
'NOT SPECIFIED',(#52269));
#52312=COLOUR_RGB('Grey',0.48,0.52,0.57);
#52313=FILL_AREA_STYLE_COLOUR('',#52312);
#52314=FILL_AREA_STYLE('',(#52313));
#52315=SURFACE_STYLE_FILL_AREA(#52314);
#52316=SURFACE_SIDE_STYLE('',(#52315));
#52317=SURFACE_STYLE_USAGE(.BOTH.,#52316);
#52318=PRESENTATION_STYLE_ASSIGNMENT((#52317));
ENDSEC;
END-ISO-10303-21;
